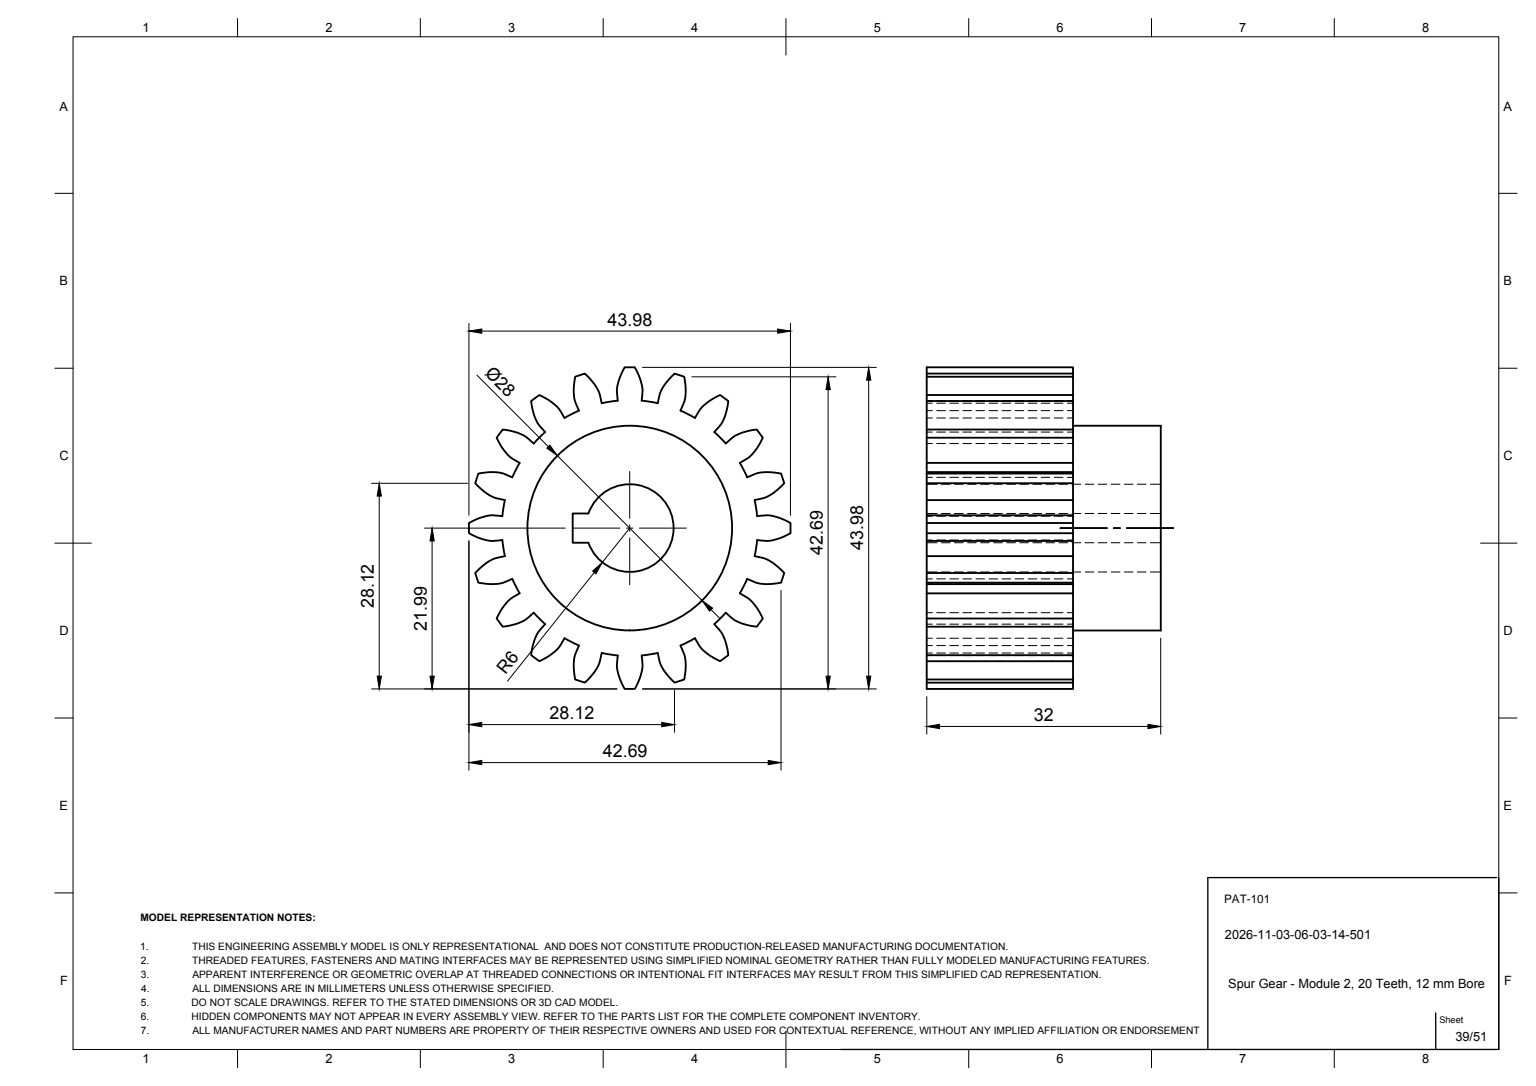
ISO-10303-21;
HEADER;
/* Generated by software containing ST-Developer
 * from STEP Tools, Inc. (www.steptools.com) 
 */

FILE_DESCRIPTION(
/* description */ ('Spur gear reduction stage 2-1 on bearing plates'),
/* implementation_level */ '2;1');

FILE_NAME(
/* name */ 'Spur Gear - Module 2, 20 Teeth, 12 mm Bore.step',
/* time_stamp */ '2026-10-28T03:22:07-07:00',
/* author */ (''),
/* organization */ (''),
/* preprocessor_version */ 'ST-DEVELOPER v20.2',
/* originating_system */ 'Autodesk Translation Framework v15.17.0.0',
/* authorisation */ '');

FILE_SCHEMA (('AUTOMOTIVE_DESIGN { 1 0 10303 214 3 1 1 }'));
ENDSEC;

DATA;
#10=MECHANICAL_DESIGN_GEOMETRIC_PRESENTATION_REPRESENTATION('',(#993),#53909);
#11=(
BOUNDED_SURFACE()
B_SPLINE_SURFACE(5,1,((#21141,#21142),(#21143,#21144),(#21145,#21146),(#21147,
#21148),(#21149,#21150),(#21151,#21152),(#21153,#21154),(#21155,#21156),
(#21157,#21158),(#21159,#21160),(#21161,#21162),(#21163,#21164),(#21165,
#21166),(#21167,#21168),(#21169,#21170),(#21171,#21172),(#21173,#21174),
(#21175,#21176),(#21177,#21178),(#21179,#21180),(#21181,#21182),(#21183,
#21184),(#21185,#21186),(#21187,#21188),(#21189,#21190),(#21191,#21192),
(#21193,#21194),(#21195,#21196),(#21197,#21198),(#21199,#21200),(#21201,
#21202),(#21203,#21204),(#21205,#21206),(#21207,#21208),(#21209,#21210),
(#21211,#21212),(#21213,#21214),(#21215,#21216),(#21217,#21218),(#21219,
#21220),(#21221,#21222),(#21223,#21224),(#21225,#21226),(#21227,#21228),
(#21229,#21230),(#21231,#21232),(#21233,#21234),(#21235,#21236),(#21237,
#21238),(#21239,#21240),(#21241,#21242),(#21243,#21244),(#21245,#21246),
(#21247,#21248),(#21249,#21250),(#21251,#21252),(#21253,#21254),(#21255,
#21256),(#21257,#21258),(#21259,#21260),(#21261,#21262),(#21263,#21264),
(#21265,#21266),(#21267,#21268),(#21269,#21270),(#21271,#21272),(#21273,
#21274),(#21275,#21276),(#21277,#21278),(#21279,#21280)),.UNSPECIFIED.,
 .F.,.F.,.F.)
B_SPLINE_SURFACE_WITH_KNOTS((6,1,1,1,1,1,1,1,1,1,1,1,1,1,1,1,1,1,1,1,1,
1,1,1,1,1,1,1,1,1,1,1,1,1,1,1,1,1,1,1,1,1,1,1,1,1,1,1,1,1,1,1,1,1,1,1,1,
1,1,1,1,1,1,1,1,6),(2,2),(-1.,-0.984615384615383,-0.969230769230768,-0.953846153846152,
-0.938461538461537,-0.923076923076922,-0.907692307692306,-0.892307692307691,
-0.876923076923076,-0.86153846153846,-0.846153846153845,-0.83076923076923,
-0.815384615384614,-0.799999999999999,-0.784615384615384,-0.769230769230768,
-0.753846153846153,-0.738461538461538,-0.723076923076922,-0.707692307692307,
-0.692307692307692,-0.676923076923076,-0.661538461538461,-0.646153846153846,
-0.63076923076923,-0.615384615384615,-0.6,-0.584615384615384,-0.569230769230769,
-0.553846153846154,-0.538461538461538,-0.523076923076923,-0.507692307692308,
-0.492307692307692,-0.476923076923077,-0.461538461538462,-0.446153846153846,
-0.430769230769231,-0.415384615384615,-0.4,-0.384615384615385,-0.369230769230769,
-0.353846153846154,-0.338461538461538,-0.323076923076923,-0.307692307692308,
-0.292307692307692,-0.276923076923077,-0.261538461538462,-0.246153846153846,
-0.230769230769231,-0.215384615384615,-0.2,-0.184615384615385,-0.169230769230769,
-0.153846153846154,-0.138461538461538,-0.123076923076923,-0.107692307692308,
-0.0923076923076923,-0.0769230769230769,-0.0615384615384615,-0.0461538461538462,
-0.0307692307692308,-0.0153846153846154,0.),(-1.,1.),.UNSPECIFIED.)
GEOMETRIC_REPRESENTATION_ITEM()
RATIONAL_B_SPLINE_SURFACE(((1.,1.),(1.,1.),(1.,1.),(1.,1.),(1.,1.),(1.,
1.),(1.,1.),(1.,1.),(1.,1.),(1.,1.),(1.,1.),(1.,1.),(1.,1.),(1.,1.),(1.,
1.),(1.,1.),(1.,1.),(1.,1.),(1.,1.),(1.,1.),(1.,1.),(1.,1.),(1.,1.),(1.,
1.),(1.,1.),(1.,1.),(1.,1.),(1.,1.),(1.,1.),(1.,1.),(1.,1.),(1.,1.),(1.,
1.),(1.,1.),(1.,1.),(1.,1.),(1.,1.),(1.,1.),(1.,1.),(1.,1.),(1.,1.),(1.,
1.),(1.,1.),(1.,1.),(1.,1.),(1.,1.),(1.,1.),(1.,1.),(1.,1.),(1.,1.),(1.,
1.),(1.,1.),(1.,1.),(1.,1.),(1.,1.),(1.,1.),(1.,1.),(1.,1.),(1.,1.),(1.,
1.),(1.,1.),(1.,1.),(1.,1.),(1.,1.),(1.,1.),(1.,1.),(1.,1.),(1.,1.),(1.,
1.),(1.,1.)))
REPRESENTATION_ITEM('')
SURFACE()
);
#12=(
BOUNDED_SURFACE()
B_SPLINE_SURFACE(5,1,((#21359,#21360),(#21361,#21362),(#21363,#21364),(#21365,
#21366),(#21367,#21368),(#21369,#21370),(#21371,#21372),(#21373,#21374),
(#21375,#21376),(#21377,#21378),(#21379,#21380),(#21381,#21382),(#21383,
#21384),(#21385,#21386),(#21387,#21388),(#21389,#21390),(#21391,#21392),
(#21393,#21394),(#21395,#21396),(#21397,#21398),(#21399,#21400),(#21401,
#21402),(#21403,#21404),(#21405,#21406),(#21407,#21408),(#21409,#21410),
(#21411,#21412),(#21413,#21414),(#21415,#21416),(#21417,#21418),(#21419,
#21420),(#21421,#21422),(#21423,#21424),(#21425,#21426),(#21427,#21428),
(#21429,#21430),(#21431,#21432),(#21433,#21434),(#21435,#21436),(#21437,
#21438),(#21439,#21440),(#21441,#21442),(#21443,#21444),(#21445,#21446),
(#21447,#21448),(#21449,#21450),(#21451,#21452),(#21453,#21454),(#21455,
#21456),(#21457,#21458),(#21459,#21460),(#21461,#21462),(#21463,#21464),
(#21465,#21466),(#21467,#21468),(#21469,#21470),(#21471,#21472),(#21473,
#21474),(#21475,#21476),(#21477,#21478),(#21479,#21480),(#21481,#21482),
(#21483,#21484),(#21485,#21486),(#21487,#21488),(#21489,#21490),(#21491,
#21492),(#21493,#21494),(#21495,#21496),(#21497,#21498)),.UNSPECIFIED.,
 .F.,.F.,.F.)
B_SPLINE_SURFACE_WITH_KNOTS((6,1,1,1,1,1,1,1,1,1,1,1,1,1,1,1,1,1,1,1,1,
1,1,1,1,1,1,1,1,1,1,1,1,1,1,1,1,1,1,1,1,1,1,1,1,1,1,1,1,1,1,1,1,1,1,1,1,
1,1,1,1,1,1,1,1,6),(2,2),(-1.,-0.984615384615383,-0.969230769230768,-0.953846153846152,
-0.938461538461537,-0.923076923076922,-0.907692307692306,-0.892307692307691,
-0.876923076923076,-0.86153846153846,-0.846153846153845,-0.83076923076923,
-0.815384615384614,-0.799999999999999,-0.784615384615384,-0.769230769230768,
-0.753846153846153,-0.738461538461538,-0.723076923076922,-0.707692307692307,
-0.692307692307692,-0.676923076923076,-0.661538461538461,-0.646153846153846,
-0.63076923076923,-0.615384615384615,-0.6,-0.584615384615384,-0.569230769230769,
-0.553846153846154,-0.538461538461538,-0.523076923076923,-0.507692307692308,
-0.492307692307692,-0.476923076923077,-0.461538461538462,-0.446153846153846,
-0.430769230769231,-0.415384615384615,-0.4,-0.384615384615385,-0.369230769230769,
-0.353846153846154,-0.338461538461538,-0.323076923076923,-0.307692307692308,
-0.292307692307692,-0.276923076923077,-0.261538461538462,-0.246153846153846,
-0.230769230769231,-0.215384615384615,-0.2,-0.184615384615385,-0.169230769230769,
-0.153846153846154,-0.138461538461538,-0.123076923076923,-0.107692307692308,
-0.0923076923076923,-0.0769230769230769,-0.0615384615384615,-0.0461538461538462,
-0.0307692307692308,-0.0153846153846154,0.),(-1.,1.),.UNSPECIFIED.)
GEOMETRIC_REPRESENTATION_ITEM()
RATIONAL_B_SPLINE_SURFACE(((1.,1.),(1.,1.),(1.,1.),(1.,1.),(1.,1.),(1.,
1.),(1.,1.),(1.,1.),(1.,1.),(1.,1.),(1.,1.),(1.,1.),(1.,1.),(1.,1.),(1.,
1.),(1.,1.),(1.,1.),(1.,1.),(1.,1.),(1.,1.),(1.,1.),(1.,1.),(1.,1.),(1.,
1.),(1.,1.),(1.,1.),(1.,1.),(1.,1.),(1.,1.),(1.,1.),(1.,1.),(1.,1.),(1.,
1.),(1.,1.),(1.,1.),(1.,1.),(1.,1.),(1.,1.),(1.,1.),(1.,1.),(1.,1.),(1.,
1.),(1.,1.),(1.,1.),(1.,1.),(1.,1.),(1.,1.),(1.,1.),(1.,1.),(1.,1.),(1.,
1.),(1.,1.),(1.,1.),(1.,1.),(1.,1.),(1.,1.),(1.,1.),(1.,1.),(1.,1.),(1.,
1.),(1.,1.),(1.,1.),(1.,1.),(1.,1.),(1.,1.),(1.,1.),(1.,1.),(1.,1.),(1.,
1.),(1.,1.)))
REPRESENTATION_ITEM('')
SURFACE()
);
#13=(
BOUNDED_SURFACE()
B_SPLINE_SURFACE(5,1,((#21575,#21576),(#21577,#21578),(#21579,#21580),(#21581,
#21582),(#21583,#21584),(#21585,#21586),(#21587,#21588),(#21589,#21590),
(#21591,#21592),(#21593,#21594),(#21595,#21596),(#21597,#21598),(#21599,
#21600),(#21601,#21602),(#21603,#21604),(#21605,#21606),(#21607,#21608),
(#21609,#21610),(#21611,#21612),(#21613,#21614),(#21615,#21616),(#21617,
#21618),(#21619,#21620),(#21621,#21622),(#21623,#21624),(#21625,#21626),
(#21627,#21628),(#21629,#21630),(#21631,#21632),(#21633,#21634),(#21635,
#21636),(#21637,#21638),(#21639,#21640),(#21641,#21642),(#21643,#21644),
(#21645,#21646),(#21647,#21648),(#21649,#21650),(#21651,#21652),(#21653,
#21654),(#21655,#21656),(#21657,#21658),(#21659,#21660),(#21661,#21662),
(#21663,#21664),(#21665,#21666),(#21667,#21668),(#21669,#21670),(#21671,
#21672),(#21673,#21674),(#21675,#21676),(#21677,#21678),(#21679,#21680),
(#21681,#21682),(#21683,#21684),(#21685,#21686),(#21687,#21688),(#21689,
#21690),(#21691,#21692),(#21693,#21694),(#21695,#21696),(#21697,#21698),
(#21699,#21700),(#21701,#21702),(#21703,#21704),(#21705,#21706),(#21707,
#21708),(#21709,#21710),(#21711,#21712),(#21713,#21714)),.UNSPECIFIED.,
 .F.,.F.,.F.)
B_SPLINE_SURFACE_WITH_KNOTS((6,1,1,1,1,1,1,1,1,1,1,1,1,1,1,1,1,1,1,1,1,
1,1,1,1,1,1,1,1,1,1,1,1,1,1,1,1,1,1,1,1,1,1,1,1,1,1,1,1,1,1,1,1,1,1,1,1,
1,1,1,1,1,1,1,1,6),(2,2),(-1.,-0.984615384615383,-0.969230769230768,-0.953846153846152,
-0.938461538461537,-0.923076923076922,-0.907692307692306,-0.892307692307691,
-0.876923076923076,-0.86153846153846,-0.846153846153845,-0.83076923076923,
-0.815384615384614,-0.799999999999999,-0.784615384615384,-0.769230769230768,
-0.753846153846153,-0.738461538461538,-0.723076923076922,-0.707692307692307,
-0.692307692307692,-0.676923076923076,-0.661538461538461,-0.646153846153846,
-0.63076923076923,-0.615384615384615,-0.6,-0.584615384615384,-0.569230769230769,
-0.553846153846154,-0.538461538461538,-0.523076923076923,-0.507692307692308,
-0.492307692307692,-0.476923076923077,-0.461538461538462,-0.446153846153846,
-0.430769230769231,-0.415384615384615,-0.4,-0.384615384615385,-0.369230769230769,
-0.353846153846154,-0.338461538461538,-0.323076923076923,-0.307692307692308,
-0.292307692307692,-0.276923076923077,-0.261538461538462,-0.246153846153846,
-0.230769230769231,-0.215384615384615,-0.2,-0.184615384615385,-0.169230769230769,
-0.153846153846154,-0.138461538461538,-0.123076923076923,-0.107692307692308,
-0.0923076923076923,-0.0769230769230769,-0.0615384615384615,-0.0461538461538462,
-0.0307692307692308,-0.0153846153846154,0.),(-1.,1.),.UNSPECIFIED.)
GEOMETRIC_REPRESENTATION_ITEM()
RATIONAL_B_SPLINE_SURFACE(((1.,1.),(1.,1.),(1.,1.),(1.,1.),(1.,1.),(1.,
1.),(1.,1.),(1.,1.),(1.,1.),(1.,1.),(1.,1.),(1.,1.),(1.,1.),(1.,1.),(1.,
1.),(1.,1.),(1.,1.),(1.,1.),(1.,1.),(1.,1.),(1.,1.),(1.,1.),(1.,1.),(1.,
1.),(1.,1.),(1.,1.),(1.,1.),(1.,1.),(1.,1.),(1.,1.),(1.,1.),(1.,1.),(1.,
1.),(1.,1.),(1.,1.),(1.,1.),(1.,1.),(1.,1.),(1.,1.),(1.,1.),(1.,1.),(1.,
1.),(1.,1.),(1.,1.),(1.,1.),(1.,1.),(1.,1.),(1.,1.),(1.,1.),(1.,1.),(1.,
1.),(1.,1.),(1.,1.),(1.,1.),(1.,1.),(1.,1.),(1.,1.),(1.,1.),(1.,1.),(1.,
1.),(1.,1.),(1.,1.),(1.,1.),(1.,1.),(1.,1.),(1.,1.),(1.,1.),(1.,1.),(1.,
1.),(1.,1.)))
REPRESENTATION_ITEM('')
SURFACE()
);
#14=(
BOUNDED_SURFACE()
B_SPLINE_SURFACE(5,1,((#21791,#21792),(#21793,#21794),(#21795,#21796),(#21797,
#21798),(#21799,#21800),(#21801,#21802),(#21803,#21804),(#21805,#21806),
(#21807,#21808),(#21809,#21810),(#21811,#21812),(#21813,#21814),(#21815,
#21816),(#21817,#21818),(#21819,#21820),(#21821,#21822),(#21823,#21824),
(#21825,#21826),(#21827,#21828),(#21829,#21830),(#21831,#21832),(#21833,
#21834),(#21835,#21836),(#21837,#21838),(#21839,#21840),(#21841,#21842),
(#21843,#21844),(#21845,#21846),(#21847,#21848),(#21849,#21850),(#21851,
#21852),(#21853,#21854),(#21855,#21856),(#21857,#21858),(#21859,#21860),
(#21861,#21862),(#21863,#21864),(#21865,#21866),(#21867,#21868),(#21869,
#21870),(#21871,#21872),(#21873,#21874),(#21875,#21876),(#21877,#21878),
(#21879,#21880),(#21881,#21882),(#21883,#21884),(#21885,#21886),(#21887,
#21888),(#21889,#21890),(#21891,#21892),(#21893,#21894),(#21895,#21896),
(#21897,#21898),(#21899,#21900),(#21901,#21902),(#21903,#21904),(#21905,
#21906),(#21907,#21908),(#21909,#21910),(#21911,#21912),(#21913,#21914),
(#21915,#21916),(#21917,#21918),(#21919,#21920),(#21921,#21922),(#21923,
#21924),(#21925,#21926),(#21927,#21928),(#21929,#21930)),.UNSPECIFIED.,
 .F.,.F.,.F.)
B_SPLINE_SURFACE_WITH_KNOTS((6,1,1,1,1,1,1,1,1,1,1,1,1,1,1,1,1,1,1,1,1,
1,1,1,1,1,1,1,1,1,1,1,1,1,1,1,1,1,1,1,1,1,1,1,1,1,1,1,1,1,1,1,1,1,1,1,1,
1,1,1,1,1,1,1,1,6),(2,2),(-1.,-0.984615384615383,-0.969230769230768,-0.953846153846152,
-0.938461538461537,-0.923076923076922,-0.907692307692306,-0.892307692307691,
-0.876923076923076,-0.86153846153846,-0.846153846153845,-0.83076923076923,
-0.815384615384614,-0.799999999999999,-0.784615384615384,-0.769230769230768,
-0.753846153846153,-0.738461538461538,-0.723076923076922,-0.707692307692307,
-0.692307692307692,-0.676923076923076,-0.661538461538461,-0.646153846153846,
-0.63076923076923,-0.615384615384615,-0.6,-0.584615384615384,-0.569230769230769,
-0.553846153846154,-0.538461538461538,-0.523076923076923,-0.507692307692308,
-0.492307692307692,-0.476923076923077,-0.461538461538462,-0.446153846153846,
-0.430769230769231,-0.415384615384615,-0.4,-0.384615384615385,-0.369230769230769,
-0.353846153846154,-0.338461538461538,-0.323076923076923,-0.307692307692308,
-0.292307692307692,-0.276923076923077,-0.261538461538462,-0.246153846153846,
-0.230769230769231,-0.215384615384615,-0.2,-0.184615384615385,-0.169230769230769,
-0.153846153846154,-0.138461538461538,-0.123076923076923,-0.107692307692308,
-0.0923076923076923,-0.0769230769230769,-0.0615384615384615,-0.0461538461538462,
-0.0307692307692308,-0.0153846153846154,0.),(-1.,1.),.UNSPECIFIED.)
GEOMETRIC_REPRESENTATION_ITEM()
RATIONAL_B_SPLINE_SURFACE(((1.,1.),(1.,1.),(1.,1.),(1.,1.),(1.,1.),(1.,
1.),(1.,1.),(1.,1.),(1.,1.),(1.,1.),(1.,1.),(1.,1.),(1.,1.),(1.,1.),(1.,
1.),(1.,1.),(1.,1.),(1.,1.),(1.,1.),(1.,1.),(1.,1.),(1.,1.),(1.,1.),(1.,
1.),(1.,1.),(1.,1.),(1.,1.),(1.,1.),(1.,1.),(1.,1.),(1.,1.),(1.,1.),(1.,
1.),(1.,1.),(1.,1.),(1.,1.),(1.,1.),(1.,1.),(1.,1.),(1.,1.),(1.,1.),(1.,
1.),(1.,1.),(1.,1.),(1.,1.),(1.,1.),(1.,1.),(1.,1.),(1.,1.),(1.,1.),(1.,
1.),(1.,1.),(1.,1.),(1.,1.),(1.,1.),(1.,1.),(1.,1.),(1.,1.),(1.,1.),(1.,
1.),(1.,1.),(1.,1.),(1.,1.),(1.,1.),(1.,1.),(1.,1.),(1.,1.),(1.,1.),(1.,
1.),(1.,1.)))
REPRESENTATION_ITEM('')
SURFACE()
);
#15=(
BOUNDED_SURFACE()
B_SPLINE_SURFACE(5,1,((#22007,#22008),(#22009,#22010),(#22011,#22012),(#22013,
#22014),(#22015,#22016),(#22017,#22018),(#22019,#22020),(#22021,#22022),
(#22023,#22024),(#22025,#22026),(#22027,#22028),(#22029,#22030),(#22031,
#22032),(#22033,#22034),(#22035,#22036),(#22037,#22038),(#22039,#22040),
(#22041,#22042),(#22043,#22044),(#22045,#22046),(#22047,#22048),(#22049,
#22050),(#22051,#22052),(#22053,#22054),(#22055,#22056),(#22057,#22058),
(#22059,#22060),(#22061,#22062),(#22063,#22064),(#22065,#22066),(#22067,
#22068),(#22069,#22070),(#22071,#22072),(#22073,#22074),(#22075,#22076),
(#22077,#22078),(#22079,#22080),(#22081,#22082),(#22083,#22084),(#22085,
#22086),(#22087,#22088),(#22089,#22090),(#22091,#22092),(#22093,#22094),
(#22095,#22096),(#22097,#22098),(#22099,#22100),(#22101,#22102),(#22103,
#22104),(#22105,#22106),(#22107,#22108),(#22109,#22110),(#22111,#22112),
(#22113,#22114),(#22115,#22116),(#22117,#22118),(#22119,#22120),(#22121,
#22122),(#22123,#22124),(#22125,#22126),(#22127,#22128),(#22129,#22130),
(#22131,#22132),(#22133,#22134),(#22135,#22136),(#22137,#22138),(#22139,
#22140),(#22141,#22142),(#22143,#22144),(#22145,#22146)),.UNSPECIFIED.,
 .F.,.F.,.F.)
B_SPLINE_SURFACE_WITH_KNOTS((6,1,1,1,1,1,1,1,1,1,1,1,1,1,1,1,1,1,1,1,1,
1,1,1,1,1,1,1,1,1,1,1,1,1,1,1,1,1,1,1,1,1,1,1,1,1,1,1,1,1,1,1,1,1,1,1,1,
1,1,1,1,1,1,1,1,6),(2,2),(-1.,-0.984615384615383,-0.969230769230768,-0.953846153846152,
-0.938461538461537,-0.923076923076922,-0.907692307692306,-0.892307692307691,
-0.876923076923076,-0.86153846153846,-0.846153846153845,-0.83076923076923,
-0.815384615384614,-0.799999999999999,-0.784615384615384,-0.769230769230768,
-0.753846153846153,-0.738461538461538,-0.723076923076922,-0.707692307692307,
-0.692307692307692,-0.676923076923076,-0.661538461538461,-0.646153846153846,
-0.63076923076923,-0.615384615384615,-0.6,-0.584615384615384,-0.569230769230769,
-0.553846153846154,-0.538461538461538,-0.523076923076923,-0.507692307692308,
-0.492307692307692,-0.476923076923077,-0.461538461538462,-0.446153846153846,
-0.430769230769231,-0.415384615384615,-0.4,-0.384615384615385,-0.369230769230769,
-0.353846153846154,-0.338461538461538,-0.323076923076923,-0.307692307692308,
-0.292307692307692,-0.276923076923077,-0.261538461538462,-0.246153846153846,
-0.230769230769231,-0.215384615384615,-0.2,-0.184615384615385,-0.169230769230769,
-0.153846153846154,-0.138461538461538,-0.123076923076923,-0.107692307692308,
-0.0923076923076923,-0.0769230769230769,-0.0615384615384615,-0.0461538461538462,
-0.0307692307692308,-0.0153846153846154,0.),(-1.,1.),.UNSPECIFIED.)
GEOMETRIC_REPRESENTATION_ITEM()
RATIONAL_B_SPLINE_SURFACE(((1.,1.),(1.,1.),(1.,1.),(1.,1.),(1.,1.),(1.,
1.),(1.,1.),(1.,1.),(1.,1.),(1.,1.),(1.,1.),(1.,1.),(1.,1.),(1.,1.),(1.,
1.),(1.,1.),(1.,1.),(1.,1.),(1.,1.),(1.,1.),(1.,1.),(1.,1.),(1.,1.),(1.,
1.),(1.,1.),(1.,1.),(1.,1.),(1.,1.),(1.,1.),(1.,1.),(1.,1.),(1.,1.),(1.,
1.),(1.,1.),(1.,1.),(1.,1.),(1.,1.),(1.,1.),(1.,1.),(1.,1.),(1.,1.),(1.,
1.),(1.,1.),(1.,1.),(1.,1.),(1.,1.),(1.,1.),(1.,1.),(1.,1.),(1.,1.),(1.,
1.),(1.,1.),(1.,1.),(1.,1.),(1.,1.),(1.,1.),(1.,1.),(1.,1.),(1.,1.),(1.,
1.),(1.,1.),(1.,1.),(1.,1.),(1.,1.),(1.,1.),(1.,1.),(1.,1.),(1.,1.),(1.,
1.),(1.,1.)))
REPRESENTATION_ITEM('')
SURFACE()
);
#16=(
BOUNDED_SURFACE()
B_SPLINE_SURFACE(5,1,((#22223,#22224),(#22225,#22226),(#22227,#22228),(#22229,
#22230),(#22231,#22232),(#22233,#22234),(#22235,#22236),(#22237,#22238),
(#22239,#22240),(#22241,#22242),(#22243,#22244),(#22245,#22246),(#22247,
#22248),(#22249,#22250),(#22251,#22252),(#22253,#22254),(#22255,#22256),
(#22257,#22258),(#22259,#22260),(#22261,#22262),(#22263,#22264),(#22265,
#22266),(#22267,#22268),(#22269,#22270),(#22271,#22272),(#22273,#22274),
(#22275,#22276),(#22277,#22278),(#22279,#22280),(#22281,#22282),(#22283,
#22284),(#22285,#22286),(#22287,#22288),(#22289,#22290),(#22291,#22292),
(#22293,#22294),(#22295,#22296),(#22297,#22298),(#22299,#22300),(#22301,
#22302),(#22303,#22304),(#22305,#22306),(#22307,#22308),(#22309,#22310),
(#22311,#22312),(#22313,#22314),(#22315,#22316),(#22317,#22318),(#22319,
#22320),(#22321,#22322),(#22323,#22324),(#22325,#22326),(#22327,#22328),
(#22329,#22330),(#22331,#22332),(#22333,#22334),(#22335,#22336),(#22337,
#22338),(#22339,#22340),(#22341,#22342),(#22343,#22344),(#22345,#22346),
(#22347,#22348),(#22349,#22350),(#22351,#22352),(#22353,#22354),(#22355,
#22356),(#22357,#22358),(#22359,#22360),(#22361,#22362)),.UNSPECIFIED.,
 .F.,.F.,.F.)
B_SPLINE_SURFACE_WITH_KNOTS((6,1,1,1,1,1,1,1,1,1,1,1,1,1,1,1,1,1,1,1,1,
1,1,1,1,1,1,1,1,1,1,1,1,1,1,1,1,1,1,1,1,1,1,1,1,1,1,1,1,1,1,1,1,1,1,1,1,
1,1,1,1,1,1,1,1,6),(2,2),(-1.,-0.984615384615383,-0.969230769230768,-0.953846153846152,
-0.938461538461537,-0.923076923076922,-0.907692307692306,-0.892307692307691,
-0.876923076923076,-0.86153846153846,-0.846153846153845,-0.83076923076923,
-0.815384615384614,-0.799999999999999,-0.784615384615384,-0.769230769230768,
-0.753846153846153,-0.738461538461538,-0.723076923076922,-0.707692307692307,
-0.692307692307692,-0.676923076923076,-0.661538461538461,-0.646153846153846,
-0.63076923076923,-0.615384615384615,-0.6,-0.584615384615384,-0.569230769230769,
-0.553846153846154,-0.538461538461538,-0.523076923076923,-0.507692307692308,
-0.492307692307692,-0.476923076923077,-0.461538461538462,-0.446153846153846,
-0.430769230769231,-0.415384615384615,-0.4,-0.384615384615385,-0.369230769230769,
-0.353846153846154,-0.338461538461538,-0.323076923076923,-0.307692307692308,
-0.292307692307692,-0.276923076923077,-0.261538461538462,-0.246153846153846,
-0.230769230769231,-0.215384615384615,-0.2,-0.184615384615385,-0.169230769230769,
-0.153846153846154,-0.138461538461538,-0.123076923076923,-0.107692307692308,
-0.0923076923076923,-0.0769230769230769,-0.0615384615384615,-0.0461538461538462,
-0.0307692307692308,-0.0153846153846154,0.),(-1.,1.),.UNSPECIFIED.)
GEOMETRIC_REPRESENTATION_ITEM()
RATIONAL_B_SPLINE_SURFACE(((1.,1.),(1.,1.),(1.,1.),(1.,1.),(1.,1.),(1.,
1.),(1.,1.),(1.,1.),(1.,1.),(1.,1.),(1.,1.),(1.,1.),(1.,1.),(1.,1.),(1.,
1.),(1.,1.),(1.,1.),(1.,1.),(1.,1.),(1.,1.),(1.,1.),(1.,1.),(1.,1.),(1.,
1.),(1.,1.),(1.,1.),(1.,1.),(1.,1.),(1.,1.),(1.,1.),(1.,1.),(1.,1.),(1.,
1.),(1.,1.),(1.,1.),(1.,1.),(1.,1.),(1.,1.),(1.,1.),(1.,1.),(1.,1.),(1.,
1.),(1.,1.),(1.,1.),(1.,1.),(1.,1.),(1.,1.),(1.,1.),(1.,1.),(1.,1.),(1.,
1.),(1.,1.),(1.,1.),(1.,1.),(1.,1.),(1.,1.),(1.,1.),(1.,1.),(1.,1.),(1.,
1.),(1.,1.),(1.,1.),(1.,1.),(1.,1.),(1.,1.),(1.,1.),(1.,1.),(1.,1.),(1.,
1.),(1.,1.)))
REPRESENTATION_ITEM('')
SURFACE()
);
#17=(
BOUNDED_SURFACE()
B_SPLINE_SURFACE(5,1,((#22439,#22440),(#22441,#22442),(#22443,#22444),(#22445,
#22446),(#22447,#22448),(#22449,#22450),(#22451,#22452),(#22453,#22454),
(#22455,#22456),(#22457,#22458),(#22459,#22460),(#22461,#22462),(#22463,
#22464),(#22465,#22466),(#22467,#22468),(#22469,#22470),(#22471,#22472),
(#22473,#22474),(#22475,#22476),(#22477,#22478),(#22479,#22480),(#22481,
#22482),(#22483,#22484),(#22485,#22486),(#22487,#22488),(#22489,#22490),
(#22491,#22492),(#22493,#22494),(#22495,#22496),(#22497,#22498),(#22499,
#22500),(#22501,#22502),(#22503,#22504),(#22505,#22506),(#22507,#22508),
(#22509,#22510),(#22511,#22512),(#22513,#22514),(#22515,#22516),(#22517,
#22518),(#22519,#22520),(#22521,#22522),(#22523,#22524),(#22525,#22526),
(#22527,#22528),(#22529,#22530),(#22531,#22532),(#22533,#22534),(#22535,
#22536),(#22537,#22538),(#22539,#22540),(#22541,#22542),(#22543,#22544),
(#22545,#22546),(#22547,#22548),(#22549,#22550),(#22551,#22552),(#22553,
#22554),(#22555,#22556),(#22557,#22558),(#22559,#22560),(#22561,#22562),
(#22563,#22564),(#22565,#22566),(#22567,#22568),(#22569,#22570),(#22571,
#22572),(#22573,#22574),(#22575,#22576),(#22577,#22578)),.UNSPECIFIED.,
 .F.,.F.,.F.)
B_SPLINE_SURFACE_WITH_KNOTS((6,1,1,1,1,1,1,1,1,1,1,1,1,1,1,1,1,1,1,1,1,
1,1,1,1,1,1,1,1,1,1,1,1,1,1,1,1,1,1,1,1,1,1,1,1,1,1,1,1,1,1,1,1,1,1,1,1,
1,1,1,1,1,1,1,1,6),(2,2),(-1.,-0.984615384615383,-0.969230769230768,-0.953846153846152,
-0.938461538461537,-0.923076923076922,-0.907692307692306,-0.892307692307691,
-0.876923076923076,-0.86153846153846,-0.846153846153845,-0.83076923076923,
-0.815384615384614,-0.799999999999999,-0.784615384615384,-0.769230769230768,
-0.753846153846153,-0.738461538461538,-0.723076923076922,-0.707692307692307,
-0.692307692307692,-0.676923076923076,-0.661538461538461,-0.646153846153846,
-0.63076923076923,-0.615384615384615,-0.6,-0.584615384615384,-0.569230769230769,
-0.553846153846154,-0.538461538461538,-0.523076923076923,-0.507692307692308,
-0.492307692307692,-0.476923076923077,-0.461538461538462,-0.446153846153846,
-0.430769230769231,-0.415384615384615,-0.4,-0.384615384615385,-0.369230769230769,
-0.353846153846154,-0.338461538461538,-0.323076923076923,-0.307692307692308,
-0.292307692307692,-0.276923076923077,-0.261538461538462,-0.246153846153846,
-0.230769230769231,-0.215384615384615,-0.2,-0.184615384615385,-0.169230769230769,
-0.153846153846154,-0.138461538461538,-0.123076923076923,-0.107692307692308,
-0.0923076923076923,-0.0769230769230769,-0.0615384615384615,-0.0461538461538462,
-0.0307692307692308,-0.0153846153846154,0.),(-1.,1.),.UNSPECIFIED.)
GEOMETRIC_REPRESENTATION_ITEM()
RATIONAL_B_SPLINE_SURFACE(((1.,1.),(1.,1.),(1.,1.),(1.,1.),(1.,1.),(1.,
1.),(1.,1.),(1.,1.),(1.,1.),(1.,1.),(1.,1.),(1.,1.),(1.,1.),(1.,1.),(1.,
1.),(1.,1.),(1.,1.),(1.,1.),(1.,1.),(1.,1.),(1.,1.),(1.,1.),(1.,1.),(1.,
1.),(1.,1.),(1.,1.),(1.,1.),(1.,1.),(1.,1.),(1.,1.),(1.,1.),(1.,1.),(1.,
1.),(1.,1.),(1.,1.),(1.,1.),(1.,1.),(1.,1.),(1.,1.),(1.,1.),(1.,1.),(1.,
1.),(1.,1.),(1.,1.),(1.,1.),(1.,1.),(1.,1.),(1.,1.),(1.,1.),(1.,1.),(1.,
1.),(1.,1.),(1.,1.),(1.,1.),(1.,1.),(1.,1.),(1.,1.),(1.,1.),(1.,1.),(1.,
1.),(1.,1.),(1.,1.),(1.,1.),(1.,1.),(1.,1.),(1.,1.),(1.,1.),(1.,1.),(1.,
1.),(1.,1.)))
REPRESENTATION_ITEM('')
SURFACE()
);
#18=(
BOUNDED_SURFACE()
B_SPLINE_SURFACE(5,1,((#22655,#22656),(#22657,#22658),(#22659,#22660),(#22661,
#22662),(#22663,#22664),(#22665,#22666),(#22667,#22668),(#22669,#22670),
(#22671,#22672),(#22673,#22674),(#22675,#22676),(#22677,#22678),(#22679,
#22680),(#22681,#22682),(#22683,#22684),(#22685,#22686),(#22687,#22688),
(#22689,#22690),(#22691,#22692),(#22693,#22694),(#22695,#22696),(#22697,
#22698),(#22699,#22700),(#22701,#22702),(#22703,#22704),(#22705,#22706),
(#22707,#22708),(#22709,#22710),(#22711,#22712),(#22713,#22714),(#22715,
#22716),(#22717,#22718),(#22719,#22720),(#22721,#22722),(#22723,#22724),
(#22725,#22726),(#22727,#22728),(#22729,#22730),(#22731,#22732),(#22733,
#22734),(#22735,#22736),(#22737,#22738),(#22739,#22740),(#22741,#22742),
(#22743,#22744),(#22745,#22746),(#22747,#22748),(#22749,#22750),(#22751,
#22752),(#22753,#22754),(#22755,#22756),(#22757,#22758),(#22759,#22760),
(#22761,#22762),(#22763,#22764),(#22765,#22766),(#22767,#22768),(#22769,
#22770),(#22771,#22772),(#22773,#22774),(#22775,#22776),(#22777,#22778),
(#22779,#22780),(#22781,#22782),(#22783,#22784),(#22785,#22786),(#22787,
#22788),(#22789,#22790),(#22791,#22792),(#22793,#22794)),.UNSPECIFIED.,
 .F.,.F.,.F.)
B_SPLINE_SURFACE_WITH_KNOTS((6,1,1,1,1,1,1,1,1,1,1,1,1,1,1,1,1,1,1,1,1,
1,1,1,1,1,1,1,1,1,1,1,1,1,1,1,1,1,1,1,1,1,1,1,1,1,1,1,1,1,1,1,1,1,1,1,1,
1,1,1,1,1,1,1,1,6),(2,2),(-1.,-0.984615384615383,-0.969230769230768,-0.953846153846152,
-0.938461538461537,-0.923076923076922,-0.907692307692306,-0.892307692307691,
-0.876923076923076,-0.86153846153846,-0.846153846153845,-0.83076923076923,
-0.815384615384614,-0.799999999999999,-0.784615384615384,-0.769230769230768,
-0.753846153846153,-0.738461538461538,-0.723076923076922,-0.707692307692307,
-0.692307692307692,-0.676923076923076,-0.661538461538461,-0.646153846153846,
-0.63076923076923,-0.615384615384615,-0.6,-0.584615384615384,-0.569230769230769,
-0.553846153846154,-0.538461538461538,-0.523076923076923,-0.507692307692308,
-0.492307692307692,-0.476923076923077,-0.461538461538462,-0.446153846153846,
-0.430769230769231,-0.415384615384615,-0.4,-0.384615384615385,-0.369230769230769,
-0.353846153846154,-0.338461538461538,-0.323076923076923,-0.307692307692308,
-0.292307692307692,-0.276923076923077,-0.261538461538462,-0.246153846153846,
-0.230769230769231,-0.215384615384615,-0.2,-0.184615384615385,-0.169230769230769,
-0.153846153846154,-0.138461538461538,-0.123076923076923,-0.107692307692308,
-0.0923076923076923,-0.0769230769230769,-0.0615384615384615,-0.0461538461538462,
-0.0307692307692308,-0.0153846153846154,0.),(-1.,1.),.UNSPECIFIED.)
GEOMETRIC_REPRESENTATION_ITEM()
RATIONAL_B_SPLINE_SURFACE(((1.,1.),(1.,1.),(1.,1.),(1.,1.),(1.,1.),(1.,
1.),(1.,1.),(1.,1.),(1.,1.),(1.,1.),(1.,1.),(1.,1.),(1.,1.),(1.,1.),(1.,
1.),(1.,1.),(1.,1.),(1.,1.),(1.,1.),(1.,1.),(1.,1.),(1.,1.),(1.,1.),(1.,
1.),(1.,1.),(1.,1.),(1.,1.),(1.,1.),(1.,1.),(1.,1.),(1.,1.),(1.,1.),(1.,
1.),(1.,1.),(1.,1.),(1.,1.),(1.,1.),(1.,1.),(1.,1.),(1.,1.),(1.,1.),(1.,
1.),(1.,1.),(1.,1.),(1.,1.),(1.,1.),(1.,1.),(1.,1.),(1.,1.),(1.,1.),(1.,
1.),(1.,1.),(1.,1.),(1.,1.),(1.,1.),(1.,1.),(1.,1.),(1.,1.),(1.,1.),(1.,
1.),(1.,1.),(1.,1.),(1.,1.),(1.,1.),(1.,1.),(1.,1.),(1.,1.),(1.,1.),(1.,
1.),(1.,1.)))
REPRESENTATION_ITEM('')
SURFACE()
);
#19=(
BOUNDED_SURFACE()
B_SPLINE_SURFACE(5,1,((#22871,#22872),(#22873,#22874),(#22875,#22876),(#22877,
#22878),(#22879,#22880),(#22881,#22882),(#22883,#22884),(#22885,#22886),
(#22887,#22888),(#22889,#22890),(#22891,#22892),(#22893,#22894),(#22895,
#22896),(#22897,#22898),(#22899,#22900),(#22901,#22902),(#22903,#22904),
(#22905,#22906),(#22907,#22908),(#22909,#22910),(#22911,#22912),(#22913,
#22914),(#22915,#22916),(#22917,#22918),(#22919,#22920),(#22921,#22922),
(#22923,#22924),(#22925,#22926),(#22927,#22928),(#22929,#22930),(#22931,
#22932),(#22933,#22934),(#22935,#22936),(#22937,#22938),(#22939,#22940),
(#22941,#22942),(#22943,#22944),(#22945,#22946),(#22947,#22948),(#22949,
#22950),(#22951,#22952),(#22953,#22954),(#22955,#22956),(#22957,#22958),
(#22959,#22960),(#22961,#22962),(#22963,#22964),(#22965,#22966),(#22967,
#22968),(#22969,#22970),(#22971,#22972),(#22973,#22974),(#22975,#22976),
(#22977,#22978),(#22979,#22980),(#22981,#22982),(#22983,#22984),(#22985,
#22986),(#22987,#22988),(#22989,#22990),(#22991,#22992),(#22993,#22994),
(#22995,#22996),(#22997,#22998),(#22999,#23000),(#23001,#23002),(#23003,
#23004),(#23005,#23006),(#23007,#23008),(#23009,#23010)),.UNSPECIFIED.,
 .F.,.F.,.F.)
B_SPLINE_SURFACE_WITH_KNOTS((6,1,1,1,1,1,1,1,1,1,1,1,1,1,1,1,1,1,1,1,1,
1,1,1,1,1,1,1,1,1,1,1,1,1,1,1,1,1,1,1,1,1,1,1,1,1,1,1,1,1,1,1,1,1,1,1,1,
1,1,1,1,1,1,1,1,6),(2,2),(-1.,-0.984615384615383,-0.969230769230768,-0.953846153846152,
-0.938461538461537,-0.923076923076922,-0.907692307692306,-0.892307692307691,
-0.876923076923076,-0.86153846153846,-0.846153846153845,-0.83076923076923,
-0.815384615384614,-0.799999999999999,-0.784615384615384,-0.769230769230768,
-0.753846153846153,-0.738461538461538,-0.723076923076922,-0.707692307692307,
-0.692307692307692,-0.676923076923076,-0.661538461538461,-0.646153846153846,
-0.63076923076923,-0.615384615384615,-0.6,-0.584615384615384,-0.569230769230769,
-0.553846153846154,-0.538461538461538,-0.523076923076923,-0.507692307692308,
-0.492307692307692,-0.476923076923077,-0.461538461538462,-0.446153846153846,
-0.430769230769231,-0.415384615384615,-0.4,-0.384615384615385,-0.369230769230769,
-0.353846153846154,-0.338461538461538,-0.323076923076923,-0.307692307692308,
-0.292307692307692,-0.276923076923077,-0.261538461538462,-0.246153846153846,
-0.230769230769231,-0.215384615384615,-0.2,-0.184615384615385,-0.169230769230769,
-0.153846153846154,-0.138461538461538,-0.123076923076923,-0.107692307692308,
-0.0923076923076923,-0.0769230769230769,-0.0615384615384615,-0.0461538461538462,
-0.0307692307692308,-0.0153846153846154,0.),(-1.,1.),.UNSPECIFIED.)
GEOMETRIC_REPRESENTATION_ITEM()
RATIONAL_B_SPLINE_SURFACE(((1.,1.),(1.,1.),(1.,1.),(1.,1.),(1.,1.),(1.,
1.),(1.,1.),(1.,1.),(1.,1.),(1.,1.),(1.,1.),(1.,1.),(1.,1.),(1.,1.),(1.,
1.),(1.,1.),(1.,1.),(1.,1.),(1.,1.),(1.,1.),(1.,1.),(1.,1.),(1.,1.),(1.,
1.),(1.,1.),(1.,1.),(1.,1.),(1.,1.),(1.,1.),(1.,1.),(1.,1.),(1.,1.),(1.,
1.),(1.,1.),(1.,1.),(1.,1.),(1.,1.),(1.,1.),(1.,1.),(1.,1.),(1.,1.),(1.,
1.),(1.,1.),(1.,1.),(1.,1.),(1.,1.),(1.,1.),(1.,1.),(1.,1.),(1.,1.),(1.,
1.),(1.,1.),(1.,1.),(1.,1.),(1.,1.),(1.,1.),(1.,1.),(1.,1.),(1.,1.),(1.,
1.),(1.,1.),(1.,1.),(1.,1.),(1.,1.),(1.,1.),(1.,1.),(1.,1.),(1.,1.),(1.,
1.),(1.,1.)))
REPRESENTATION_ITEM('')
SURFACE()
);
#20=(
BOUNDED_SURFACE()
B_SPLINE_SURFACE(5,1,((#23087,#23088),(#23089,#23090),(#23091,#23092),(#23093,
#23094),(#23095,#23096),(#23097,#23098),(#23099,#23100),(#23101,#23102),
(#23103,#23104),(#23105,#23106),(#23107,#23108),(#23109,#23110),(#23111,
#23112),(#23113,#23114),(#23115,#23116),(#23117,#23118),(#23119,#23120),
(#23121,#23122),(#23123,#23124),(#23125,#23126),(#23127,#23128),(#23129,
#23130),(#23131,#23132),(#23133,#23134),(#23135,#23136),(#23137,#23138),
(#23139,#23140),(#23141,#23142),(#23143,#23144),(#23145,#23146),(#23147,
#23148),(#23149,#23150),(#23151,#23152),(#23153,#23154),(#23155,#23156),
(#23157,#23158),(#23159,#23160),(#23161,#23162),(#23163,#23164),(#23165,
#23166),(#23167,#23168),(#23169,#23170),(#23171,#23172),(#23173,#23174),
(#23175,#23176),(#23177,#23178),(#23179,#23180),(#23181,#23182),(#23183,
#23184),(#23185,#23186),(#23187,#23188),(#23189,#23190),(#23191,#23192),
(#23193,#23194),(#23195,#23196),(#23197,#23198),(#23199,#23200),(#23201,
#23202),(#23203,#23204),(#23205,#23206),(#23207,#23208),(#23209,#23210),
(#23211,#23212),(#23213,#23214),(#23215,#23216),(#23217,#23218),(#23219,
#23220),(#23221,#23222),(#23223,#23224),(#23225,#23226)),.UNSPECIFIED.,
 .F.,.F.,.F.)
B_SPLINE_SURFACE_WITH_KNOTS((6,1,1,1,1,1,1,1,1,1,1,1,1,1,1,1,1,1,1,1,1,
1,1,1,1,1,1,1,1,1,1,1,1,1,1,1,1,1,1,1,1,1,1,1,1,1,1,1,1,1,1,1,1,1,1,1,1,
1,1,1,1,1,1,1,1,6),(2,2),(-1.,-0.984615384615383,-0.969230769230768,-0.953846153846152,
-0.938461538461537,-0.923076923076922,-0.907692307692306,-0.892307692307691,
-0.876923076923076,-0.86153846153846,-0.846153846153845,-0.83076923076923,
-0.815384615384614,-0.799999999999999,-0.784615384615384,-0.769230769230768,
-0.753846153846153,-0.738461538461538,-0.723076923076922,-0.707692307692307,
-0.692307692307692,-0.676923076923076,-0.661538461538461,-0.646153846153846,
-0.63076923076923,-0.615384615384615,-0.6,-0.584615384615384,-0.569230769230769,
-0.553846153846154,-0.538461538461538,-0.523076923076923,-0.507692307692308,
-0.492307692307692,-0.476923076923077,-0.461538461538462,-0.446153846153846,
-0.430769230769231,-0.415384615384615,-0.4,-0.384615384615385,-0.369230769230769,
-0.353846153846154,-0.338461538461538,-0.323076923076923,-0.307692307692308,
-0.292307692307692,-0.276923076923077,-0.261538461538462,-0.246153846153846,
-0.230769230769231,-0.215384615384615,-0.2,-0.184615384615385,-0.169230769230769,
-0.153846153846154,-0.138461538461538,-0.123076923076923,-0.107692307692308,
-0.0923076923076923,-0.0769230769230769,-0.0615384615384615,-0.0461538461538462,
-0.0307692307692308,-0.0153846153846154,0.),(-1.,1.),.UNSPECIFIED.)
GEOMETRIC_REPRESENTATION_ITEM()
RATIONAL_B_SPLINE_SURFACE(((1.,1.),(1.,1.),(1.,1.),(1.,1.),(1.,1.),(1.,
1.),(1.,1.),(1.,1.),(1.,1.),(1.,1.),(1.,1.),(1.,1.),(1.,1.),(1.,1.),(1.,
1.),(1.,1.),(1.,1.),(1.,1.),(1.,1.),(1.,1.),(1.,1.),(1.,1.),(1.,1.),(1.,
1.),(1.,1.),(1.,1.),(1.,1.),(1.,1.),(1.,1.),(1.,1.),(1.,1.),(1.,1.),(1.,
1.),(1.,1.),(1.,1.),(1.,1.),(1.,1.),(1.,1.),(1.,1.),(1.,1.),(1.,1.),(1.,
1.),(1.,1.),(1.,1.),(1.,1.),(1.,1.),(1.,1.),(1.,1.),(1.,1.),(1.,1.),(1.,
1.),(1.,1.),(1.,1.),(1.,1.),(1.,1.),(1.,1.),(1.,1.),(1.,1.),(1.,1.),(1.,
1.),(1.,1.),(1.,1.),(1.,1.),(1.,1.),(1.,1.),(1.,1.),(1.,1.),(1.,1.),(1.,
1.),(1.,1.)))
REPRESENTATION_ITEM('')
SURFACE()
);
#21=(
BOUNDED_SURFACE()
B_SPLINE_SURFACE(5,1,((#23303,#23304),(#23305,#23306),(#23307,#23308),(#23309,
#23310),(#23311,#23312),(#23313,#23314),(#23315,#23316),(#23317,#23318),
(#23319,#23320),(#23321,#23322),(#23323,#23324),(#23325,#23326),(#23327,
#23328),(#23329,#23330),(#23331,#23332),(#23333,#23334),(#23335,#23336),
(#23337,#23338),(#23339,#23340),(#23341,#23342),(#23343,#23344),(#23345,
#23346),(#23347,#23348),(#23349,#23350),(#23351,#23352),(#23353,#23354),
(#23355,#23356),(#23357,#23358),(#23359,#23360),(#23361,#23362),(#23363,
#23364),(#23365,#23366),(#23367,#23368),(#23369,#23370),(#23371,#23372),
(#23373,#23374),(#23375,#23376),(#23377,#23378),(#23379,#23380),(#23381,
#23382),(#23383,#23384),(#23385,#23386),(#23387,#23388),(#23389,#23390),
(#23391,#23392),(#23393,#23394),(#23395,#23396),(#23397,#23398),(#23399,
#23400),(#23401,#23402),(#23403,#23404),(#23405,#23406),(#23407,#23408),
(#23409,#23410),(#23411,#23412),(#23413,#23414),(#23415,#23416),(#23417,
#23418),(#23419,#23420),(#23421,#23422),(#23423,#23424),(#23425,#23426),
(#23427,#23428),(#23429,#23430),(#23431,#23432),(#23433,#23434),(#23435,
#23436),(#23437,#23438),(#23439,#23440),(#23441,#23442)),.UNSPECIFIED.,
 .F.,.F.,.F.)
B_SPLINE_SURFACE_WITH_KNOTS((6,1,1,1,1,1,1,1,1,1,1,1,1,1,1,1,1,1,1,1,1,
1,1,1,1,1,1,1,1,1,1,1,1,1,1,1,1,1,1,1,1,1,1,1,1,1,1,1,1,1,1,1,1,1,1,1,1,
1,1,1,1,1,1,1,1,6),(2,2),(-1.,-0.984615384615383,-0.969230769230768,-0.953846153846152,
-0.938461538461537,-0.923076923076922,-0.907692307692306,-0.892307692307691,
-0.876923076923076,-0.86153846153846,-0.846153846153845,-0.83076923076923,
-0.815384615384614,-0.799999999999999,-0.784615384615384,-0.769230769230768,
-0.753846153846153,-0.738461538461538,-0.723076923076922,-0.707692307692307,
-0.692307692307692,-0.676923076923076,-0.661538461538461,-0.646153846153846,
-0.63076923076923,-0.615384615384615,-0.6,-0.584615384615384,-0.569230769230769,
-0.553846153846154,-0.538461538461538,-0.523076923076923,-0.507692307692308,
-0.492307692307692,-0.476923076923077,-0.461538461538462,-0.446153846153846,
-0.430769230769231,-0.415384615384615,-0.4,-0.384615384615385,-0.369230769230769,
-0.353846153846154,-0.338461538461538,-0.323076923076923,-0.307692307692308,
-0.292307692307692,-0.276923076923077,-0.261538461538462,-0.246153846153846,
-0.230769230769231,-0.215384615384615,-0.2,-0.184615384615385,-0.169230769230769,
-0.153846153846154,-0.138461538461538,-0.123076923076923,-0.107692307692308,
-0.0923076923076923,-0.0769230769230769,-0.0615384615384615,-0.0461538461538462,
-0.0307692307692308,-0.0153846153846154,0.),(-1.,1.),.UNSPECIFIED.)
GEOMETRIC_REPRESENTATION_ITEM()
RATIONAL_B_SPLINE_SURFACE(((1.,1.),(1.,1.),(1.,1.),(1.,1.),(1.,1.),(1.,
1.),(1.,1.),(1.,1.),(1.,1.),(1.,1.),(1.,1.),(1.,1.),(1.,1.),(1.,1.),(1.,
1.),(1.,1.),(1.,1.),(1.,1.),(1.,1.),(1.,1.),(1.,1.),(1.,1.),(1.,1.),(1.,
1.),(1.,1.),(1.,1.),(1.,1.),(1.,1.),(1.,1.),(1.,1.),(1.,1.),(1.,1.),(1.,
1.),(1.,1.),(1.,1.),(1.,1.),(1.,1.),(1.,1.),(1.,1.),(1.,1.),(1.,1.),(1.,
1.),(1.,1.),(1.,1.),(1.,1.),(1.,1.),(1.,1.),(1.,1.),(1.,1.),(1.,1.),(1.,
1.),(1.,1.),(1.,1.),(1.,1.),(1.,1.),(1.,1.),(1.,1.),(1.,1.),(1.,1.),(1.,
1.),(1.,1.),(1.,1.),(1.,1.),(1.,1.),(1.,1.),(1.,1.),(1.,1.),(1.,1.),(1.,
1.),(1.,1.)))
REPRESENTATION_ITEM('')
SURFACE()
);
#22=(
BOUNDED_SURFACE()
B_SPLINE_SURFACE(5,1,((#23519,#23520),(#23521,#23522),(#23523,#23524),(#23525,
#23526),(#23527,#23528),(#23529,#23530),(#23531,#23532),(#23533,#23534),
(#23535,#23536),(#23537,#23538),(#23539,#23540),(#23541,#23542),(#23543,
#23544),(#23545,#23546),(#23547,#23548),(#23549,#23550),(#23551,#23552),
(#23553,#23554),(#23555,#23556),(#23557,#23558),(#23559,#23560),(#23561,
#23562),(#23563,#23564),(#23565,#23566),(#23567,#23568),(#23569,#23570),
(#23571,#23572),(#23573,#23574),(#23575,#23576),(#23577,#23578),(#23579,
#23580),(#23581,#23582),(#23583,#23584),(#23585,#23586),(#23587,#23588),
(#23589,#23590),(#23591,#23592),(#23593,#23594),(#23595,#23596),(#23597,
#23598),(#23599,#23600),(#23601,#23602),(#23603,#23604),(#23605,#23606),
(#23607,#23608),(#23609,#23610),(#23611,#23612),(#23613,#23614),(#23615,
#23616),(#23617,#23618),(#23619,#23620),(#23621,#23622),(#23623,#23624),
(#23625,#23626),(#23627,#23628),(#23629,#23630),(#23631,#23632),(#23633,
#23634),(#23635,#23636),(#23637,#23638),(#23639,#23640),(#23641,#23642),
(#23643,#23644),(#23645,#23646),(#23647,#23648),(#23649,#23650),(#23651,
#23652),(#23653,#23654),(#23655,#23656),(#23657,#23658)),.UNSPECIFIED.,
 .F.,.F.,.F.)
B_SPLINE_SURFACE_WITH_KNOTS((6,1,1,1,1,1,1,1,1,1,1,1,1,1,1,1,1,1,1,1,1,
1,1,1,1,1,1,1,1,1,1,1,1,1,1,1,1,1,1,1,1,1,1,1,1,1,1,1,1,1,1,1,1,1,1,1,1,
1,1,1,1,1,1,1,1,6),(2,2),(-1.,-0.984615384615383,-0.969230769230768,-0.953846153846152,
-0.938461538461537,-0.923076923076922,-0.907692307692306,-0.892307692307691,
-0.876923076923076,-0.86153846153846,-0.846153846153845,-0.83076923076923,
-0.815384615384614,-0.799999999999999,-0.784615384615384,-0.769230769230768,
-0.753846153846153,-0.738461538461538,-0.723076923076922,-0.707692307692307,
-0.692307692307692,-0.676923076923076,-0.661538461538461,-0.646153846153846,
-0.63076923076923,-0.615384615384615,-0.6,-0.584615384615384,-0.569230769230769,
-0.553846153846154,-0.538461538461538,-0.523076923076923,-0.507692307692308,
-0.492307692307692,-0.476923076923077,-0.461538461538462,-0.446153846153846,
-0.430769230769231,-0.415384615384615,-0.4,-0.384615384615385,-0.369230769230769,
-0.353846153846154,-0.338461538461538,-0.323076923076923,-0.307692307692308,
-0.292307692307692,-0.276923076923077,-0.261538461538462,-0.246153846153846,
-0.230769230769231,-0.215384615384615,-0.2,-0.184615384615385,-0.169230769230769,
-0.153846153846154,-0.138461538461538,-0.123076923076923,-0.107692307692308,
-0.0923076923076923,-0.0769230769230769,-0.0615384615384615,-0.0461538461538462,
-0.0307692307692308,-0.0153846153846154,0.),(-1.,1.),.UNSPECIFIED.)
GEOMETRIC_REPRESENTATION_ITEM()
RATIONAL_B_SPLINE_SURFACE(((1.,1.),(1.,1.),(1.,1.),(1.,1.),(1.,1.),(1.,
1.),(1.,1.),(1.,1.),(1.,1.),(1.,1.),(1.,1.),(1.,1.),(1.,1.),(1.,1.),(1.,
1.),(1.,1.),(1.,1.),(1.,1.),(1.,1.),(1.,1.),(1.,1.),(1.,1.),(1.,1.),(1.,
1.),(1.,1.),(1.,1.),(1.,1.),(1.,1.),(1.,1.),(1.,1.),(1.,1.),(1.,1.),(1.,
1.),(1.,1.),(1.,1.),(1.,1.),(1.,1.),(1.,1.),(1.,1.),(1.,1.),(1.,1.),(1.,
1.),(1.,1.),(1.,1.),(1.,1.),(1.,1.),(1.,1.),(1.,1.),(1.,1.),(1.,1.),(1.,
1.),(1.,1.),(1.,1.),(1.,1.),(1.,1.),(1.,1.),(1.,1.),(1.,1.),(1.,1.),(1.,
1.),(1.,1.),(1.,1.),(1.,1.),(1.,1.),(1.,1.),(1.,1.),(1.,1.),(1.,1.),(1.,
1.),(1.,1.)))
REPRESENTATION_ITEM('')
SURFACE()
);
#23=(
BOUNDED_SURFACE()
B_SPLINE_SURFACE(5,1,((#23735,#23736),(#23737,#23738),(#23739,#23740),(#23741,
#23742),(#23743,#23744),(#23745,#23746),(#23747,#23748),(#23749,#23750),
(#23751,#23752),(#23753,#23754),(#23755,#23756),(#23757,#23758),(#23759,
#23760),(#23761,#23762),(#23763,#23764),(#23765,#23766),(#23767,#23768),
(#23769,#23770),(#23771,#23772),(#23773,#23774),(#23775,#23776),(#23777,
#23778),(#23779,#23780),(#23781,#23782),(#23783,#23784),(#23785,#23786),
(#23787,#23788),(#23789,#23790),(#23791,#23792),(#23793,#23794),(#23795,
#23796),(#23797,#23798),(#23799,#23800),(#23801,#23802),(#23803,#23804),
(#23805,#23806),(#23807,#23808),(#23809,#23810),(#23811,#23812),(#23813,
#23814),(#23815,#23816),(#23817,#23818),(#23819,#23820),(#23821,#23822),
(#23823,#23824),(#23825,#23826),(#23827,#23828),(#23829,#23830),(#23831,
#23832),(#23833,#23834),(#23835,#23836),(#23837,#23838),(#23839,#23840),
(#23841,#23842),(#23843,#23844),(#23845,#23846),(#23847,#23848),(#23849,
#23850),(#23851,#23852),(#23853,#23854),(#23855,#23856),(#23857,#23858),
(#23859,#23860),(#23861,#23862),(#23863,#23864),(#23865,#23866),(#23867,
#23868),(#23869,#23870),(#23871,#23872),(#23873,#23874)),.UNSPECIFIED.,
 .F.,.F.,.F.)
B_SPLINE_SURFACE_WITH_KNOTS((6,1,1,1,1,1,1,1,1,1,1,1,1,1,1,1,1,1,1,1,1,
1,1,1,1,1,1,1,1,1,1,1,1,1,1,1,1,1,1,1,1,1,1,1,1,1,1,1,1,1,1,1,1,1,1,1,1,
1,1,1,1,1,1,1,1,6),(2,2),(-1.,-0.984615384615383,-0.969230769230768,-0.953846153846152,
-0.938461538461537,-0.923076923076922,-0.907692307692306,-0.892307692307691,
-0.876923076923076,-0.86153846153846,-0.846153846153845,-0.83076923076923,
-0.815384615384614,-0.799999999999999,-0.784615384615384,-0.769230769230768,
-0.753846153846153,-0.738461538461538,-0.723076923076922,-0.707692307692307,
-0.692307692307692,-0.676923076923076,-0.661538461538461,-0.646153846153846,
-0.63076923076923,-0.615384615384615,-0.6,-0.584615384615384,-0.569230769230769,
-0.553846153846154,-0.538461538461538,-0.523076923076923,-0.507692307692308,
-0.492307692307692,-0.476923076923077,-0.461538461538462,-0.446153846153846,
-0.430769230769231,-0.415384615384615,-0.4,-0.384615384615385,-0.369230769230769,
-0.353846153846154,-0.338461538461538,-0.323076923076923,-0.307692307692308,
-0.292307692307692,-0.276923076923077,-0.261538461538462,-0.246153846153846,
-0.230769230769231,-0.215384615384615,-0.2,-0.184615384615385,-0.169230769230769,
-0.153846153846154,-0.138461538461538,-0.123076923076923,-0.107692307692308,
-0.0923076923076923,-0.0769230769230769,-0.0615384615384615,-0.0461538461538462,
-0.0307692307692308,-0.0153846153846154,0.),(-1.,1.),.UNSPECIFIED.)
GEOMETRIC_REPRESENTATION_ITEM()
RATIONAL_B_SPLINE_SURFACE(((1.,1.),(1.,1.),(1.,1.),(1.,1.),(1.,1.),(1.,
1.),(1.,1.),(1.,1.),(1.,1.),(1.,1.),(1.,1.),(1.,1.),(1.,1.),(1.,1.),(1.,
1.),(1.,1.),(1.,1.),(1.,1.),(1.,1.),(1.,1.),(1.,1.),(1.,1.),(1.,1.),(1.,
1.),(1.,1.),(1.,1.),(1.,1.),(1.,1.),(1.,1.),(1.,1.),(1.,1.),(1.,1.),(1.,
1.),(1.,1.),(1.,1.),(1.,1.),(1.,1.),(1.,1.),(1.,1.),(1.,1.),(1.,1.),(1.,
1.),(1.,1.),(1.,1.),(1.,1.),(1.,1.),(1.,1.),(1.,1.),(1.,1.),(1.,1.),(1.,
1.),(1.,1.),(1.,1.),(1.,1.),(1.,1.),(1.,1.),(1.,1.),(1.,1.),(1.,1.),(1.,
1.),(1.,1.),(1.,1.),(1.,1.),(1.,1.),(1.,1.),(1.,1.),(1.,1.),(1.,1.),(1.,
1.),(1.,1.)))
REPRESENTATION_ITEM('')
SURFACE()
);
#24=(
BOUNDED_SURFACE()
B_SPLINE_SURFACE(5,1,((#23951,#23952),(#23953,#23954),(#23955,#23956),(#23957,
#23958),(#23959,#23960),(#23961,#23962),(#23963,#23964),(#23965,#23966),
(#23967,#23968),(#23969,#23970),(#23971,#23972),(#23973,#23974),(#23975,
#23976),(#23977,#23978),(#23979,#23980),(#23981,#23982),(#23983,#23984),
(#23985,#23986),(#23987,#23988),(#23989,#23990),(#23991,#23992),(#23993,
#23994),(#23995,#23996),(#23997,#23998),(#23999,#24000),(#24001,#24002),
(#24003,#24004),(#24005,#24006),(#24007,#24008),(#24009,#24010),(#24011,
#24012),(#24013,#24014),(#24015,#24016),(#24017,#24018),(#24019,#24020),
(#24021,#24022),(#24023,#24024),(#24025,#24026),(#24027,#24028),(#24029,
#24030),(#24031,#24032),(#24033,#24034),(#24035,#24036),(#24037,#24038),
(#24039,#24040),(#24041,#24042),(#24043,#24044),(#24045,#24046),(#24047,
#24048),(#24049,#24050),(#24051,#24052),(#24053,#24054),(#24055,#24056),
(#24057,#24058),(#24059,#24060),(#24061,#24062),(#24063,#24064),(#24065,
#24066),(#24067,#24068),(#24069,#24070),(#24071,#24072),(#24073,#24074),
(#24075,#24076),(#24077,#24078),(#24079,#24080),(#24081,#24082),(#24083,
#24084),(#24085,#24086),(#24087,#24088),(#24089,#24090)),.UNSPECIFIED.,
 .F.,.F.,.F.)
B_SPLINE_SURFACE_WITH_KNOTS((6,1,1,1,1,1,1,1,1,1,1,1,1,1,1,1,1,1,1,1,1,
1,1,1,1,1,1,1,1,1,1,1,1,1,1,1,1,1,1,1,1,1,1,1,1,1,1,1,1,1,1,1,1,1,1,1,1,
1,1,1,1,1,1,1,1,6),(2,2),(-1.,-0.984615384615383,-0.969230769230768,-0.953846153846152,
-0.938461538461537,-0.923076923076922,-0.907692307692306,-0.892307692307691,
-0.876923076923076,-0.86153846153846,-0.846153846153845,-0.83076923076923,
-0.815384615384614,-0.799999999999999,-0.784615384615384,-0.769230769230768,
-0.753846153846153,-0.738461538461538,-0.723076923076922,-0.707692307692307,
-0.692307692307692,-0.676923076923076,-0.661538461538461,-0.646153846153846,
-0.63076923076923,-0.615384615384615,-0.6,-0.584615384615384,-0.569230769230769,
-0.553846153846154,-0.538461538461538,-0.523076923076923,-0.507692307692308,
-0.492307692307692,-0.476923076923077,-0.461538461538462,-0.446153846153846,
-0.430769230769231,-0.415384615384615,-0.4,-0.384615384615385,-0.369230769230769,
-0.353846153846154,-0.338461538461538,-0.323076923076923,-0.307692307692308,
-0.292307692307692,-0.276923076923077,-0.261538461538462,-0.246153846153846,
-0.230769230769231,-0.215384615384615,-0.2,-0.184615384615385,-0.169230769230769,
-0.153846153846154,-0.138461538461538,-0.123076923076923,-0.107692307692308,
-0.0923076923076923,-0.0769230769230769,-0.0615384615384615,-0.0461538461538462,
-0.0307692307692308,-0.0153846153846154,0.),(-1.,1.),.UNSPECIFIED.)
GEOMETRIC_REPRESENTATION_ITEM()
RATIONAL_B_SPLINE_SURFACE(((1.,1.),(1.,1.),(1.,1.),(1.,1.),(1.,1.),(1.,
1.),(1.,1.),(1.,1.),(1.,1.),(1.,1.),(1.,1.),(1.,1.),(1.,1.),(1.,1.),(1.,
1.),(1.,1.),(1.,1.),(1.,1.),(1.,1.),(1.,1.),(1.,1.),(1.,1.),(1.,1.),(1.,
1.),(1.,1.),(1.,1.),(1.,1.),(1.,1.),(1.,1.),(1.,1.),(1.,1.),(1.,1.),(1.,
1.),(1.,1.),(1.,1.),(1.,1.),(1.,1.),(1.,1.),(1.,1.),(1.,1.),(1.,1.),(1.,
1.),(1.,1.),(1.,1.),(1.,1.),(1.,1.),(1.,1.),(1.,1.),(1.,1.),(1.,1.),(1.,
1.),(1.,1.),(1.,1.),(1.,1.),(1.,1.),(1.,1.),(1.,1.),(1.,1.),(1.,1.),(1.,
1.),(1.,1.),(1.,1.),(1.,1.),(1.,1.),(1.,1.),(1.,1.),(1.,1.),(1.,1.),(1.,
1.),(1.,1.)))
REPRESENTATION_ITEM('')
SURFACE()
);
#25=(
BOUNDED_SURFACE()
B_SPLINE_SURFACE(5,1,((#24167,#24168),(#24169,#24170),(#24171,#24172),(#24173,
#24174),(#24175,#24176),(#24177,#24178),(#24179,#24180),(#24181,#24182),
(#24183,#24184),(#24185,#24186),(#24187,#24188),(#24189,#24190),(#24191,
#24192),(#24193,#24194),(#24195,#24196),(#24197,#24198),(#24199,#24200),
(#24201,#24202),(#24203,#24204),(#24205,#24206),(#24207,#24208),(#24209,
#24210),(#24211,#24212),(#24213,#24214),(#24215,#24216),(#24217,#24218),
(#24219,#24220),(#24221,#24222),(#24223,#24224),(#24225,#24226),(#24227,
#24228),(#24229,#24230),(#24231,#24232),(#24233,#24234),(#24235,#24236),
(#24237,#24238),(#24239,#24240),(#24241,#24242),(#24243,#24244),(#24245,
#24246),(#24247,#24248),(#24249,#24250),(#24251,#24252),(#24253,#24254),
(#24255,#24256),(#24257,#24258),(#24259,#24260),(#24261,#24262),(#24263,
#24264),(#24265,#24266),(#24267,#24268),(#24269,#24270),(#24271,#24272),
(#24273,#24274),(#24275,#24276),(#24277,#24278),(#24279,#24280),(#24281,
#24282),(#24283,#24284),(#24285,#24286),(#24287,#24288),(#24289,#24290),
(#24291,#24292),(#24293,#24294),(#24295,#24296),(#24297,#24298),(#24299,
#24300),(#24301,#24302),(#24303,#24304),(#24305,#24306)),.UNSPECIFIED.,
 .F.,.F.,.F.)
B_SPLINE_SURFACE_WITH_KNOTS((6,1,1,1,1,1,1,1,1,1,1,1,1,1,1,1,1,1,1,1,1,
1,1,1,1,1,1,1,1,1,1,1,1,1,1,1,1,1,1,1,1,1,1,1,1,1,1,1,1,1,1,1,1,1,1,1,1,
1,1,1,1,1,1,1,1,6),(2,2),(-1.,-0.984615384615383,-0.969230769230768,-0.953846153846152,
-0.938461538461537,-0.923076923076922,-0.907692307692306,-0.892307692307691,
-0.876923076923076,-0.86153846153846,-0.846153846153845,-0.83076923076923,
-0.815384615384614,-0.799999999999999,-0.784615384615384,-0.769230769230768,
-0.753846153846153,-0.738461538461538,-0.723076923076922,-0.707692307692307,
-0.692307692307692,-0.676923076923076,-0.661538461538461,-0.646153846153846,
-0.63076923076923,-0.615384615384615,-0.6,-0.584615384615384,-0.569230769230769,
-0.553846153846154,-0.538461538461538,-0.523076923076923,-0.507692307692308,
-0.492307692307692,-0.476923076923077,-0.461538461538462,-0.446153846153846,
-0.430769230769231,-0.415384615384615,-0.4,-0.384615384615385,-0.369230769230769,
-0.353846153846154,-0.338461538461538,-0.323076923076923,-0.307692307692308,
-0.292307692307692,-0.276923076923077,-0.261538461538462,-0.246153846153846,
-0.230769230769231,-0.215384615384615,-0.2,-0.184615384615385,-0.169230769230769,
-0.153846153846154,-0.138461538461538,-0.123076923076923,-0.107692307692308,
-0.0923076923076923,-0.0769230769230769,-0.0615384615384615,-0.0461538461538462,
-0.0307692307692308,-0.0153846153846154,0.),(-1.,1.),.UNSPECIFIED.)
GEOMETRIC_REPRESENTATION_ITEM()
RATIONAL_B_SPLINE_SURFACE(((1.,1.),(1.,1.),(1.,1.),(1.,1.),(1.,1.),(1.,
1.),(1.,1.),(1.,1.),(1.,1.),(1.,1.),(1.,1.),(1.,1.),(1.,1.),(1.,1.),(1.,
1.),(1.,1.),(1.,1.),(1.,1.),(1.,1.),(1.,1.),(1.,1.),(1.,1.),(1.,1.),(1.,
1.),(1.,1.),(1.,1.),(1.,1.),(1.,1.),(1.,1.),(1.,1.),(1.,1.),(1.,1.),(1.,
1.),(1.,1.),(1.,1.),(1.,1.),(1.,1.),(1.,1.),(1.,1.),(1.,1.),(1.,1.),(1.,
1.),(1.,1.),(1.,1.),(1.,1.),(1.,1.),(1.,1.),(1.,1.),(1.,1.),(1.,1.),(1.,
1.),(1.,1.),(1.,1.),(1.,1.),(1.,1.),(1.,1.),(1.,1.),(1.,1.),(1.,1.),(1.,
1.),(1.,1.),(1.,1.),(1.,1.),(1.,1.),(1.,1.),(1.,1.),(1.,1.),(1.,1.),(1.,
1.),(1.,1.)))
REPRESENTATION_ITEM('')
SURFACE()
);
#26=(
BOUNDED_SURFACE()
B_SPLINE_SURFACE(5,1,((#24383,#24384),(#24385,#24386),(#24387,#24388),(#24389,
#24390),(#24391,#24392),(#24393,#24394),(#24395,#24396),(#24397,#24398),
(#24399,#24400),(#24401,#24402),(#24403,#24404),(#24405,#24406),(#24407,
#24408),(#24409,#24410),(#24411,#24412),(#24413,#24414),(#24415,#24416),
(#24417,#24418),(#24419,#24420),(#24421,#24422),(#24423,#24424),(#24425,
#24426),(#24427,#24428),(#24429,#24430),(#24431,#24432),(#24433,#24434),
(#24435,#24436),(#24437,#24438),(#24439,#24440),(#24441,#24442),(#24443,
#24444),(#24445,#24446),(#24447,#24448),(#24449,#24450),(#24451,#24452),
(#24453,#24454),(#24455,#24456),(#24457,#24458),(#24459,#24460),(#24461,
#24462),(#24463,#24464),(#24465,#24466),(#24467,#24468),(#24469,#24470),
(#24471,#24472),(#24473,#24474),(#24475,#24476),(#24477,#24478),(#24479,
#24480),(#24481,#24482),(#24483,#24484),(#24485,#24486),(#24487,#24488),
(#24489,#24490),(#24491,#24492),(#24493,#24494),(#24495,#24496),(#24497,
#24498),(#24499,#24500),(#24501,#24502),(#24503,#24504),(#24505,#24506),
(#24507,#24508),(#24509,#24510),(#24511,#24512),(#24513,#24514),(#24515,
#24516),(#24517,#24518),(#24519,#24520),(#24521,#24522)),.UNSPECIFIED.,
 .F.,.F.,.F.)
B_SPLINE_SURFACE_WITH_KNOTS((6,1,1,1,1,1,1,1,1,1,1,1,1,1,1,1,1,1,1,1,1,
1,1,1,1,1,1,1,1,1,1,1,1,1,1,1,1,1,1,1,1,1,1,1,1,1,1,1,1,1,1,1,1,1,1,1,1,
1,1,1,1,1,1,1,1,6),(2,2),(-1.,-0.984615384615383,-0.969230769230768,-0.953846153846152,
-0.938461538461537,-0.923076923076922,-0.907692307692306,-0.892307692307691,
-0.876923076923076,-0.86153846153846,-0.846153846153845,-0.83076923076923,
-0.815384615384614,-0.799999999999999,-0.784615384615384,-0.769230769230768,
-0.753846153846153,-0.738461538461538,-0.723076923076922,-0.707692307692307,
-0.692307692307692,-0.676923076923076,-0.661538461538461,-0.646153846153846,
-0.63076923076923,-0.615384615384615,-0.6,-0.584615384615384,-0.569230769230769,
-0.553846153846154,-0.538461538461538,-0.523076923076923,-0.507692307692308,
-0.492307692307692,-0.476923076923077,-0.461538461538462,-0.446153846153846,
-0.430769230769231,-0.415384615384615,-0.4,-0.384615384615385,-0.369230769230769,
-0.353846153846154,-0.338461538461538,-0.323076923076923,-0.307692307692308,
-0.292307692307692,-0.276923076923077,-0.261538461538462,-0.246153846153846,
-0.230769230769231,-0.215384615384615,-0.2,-0.184615384615385,-0.169230769230769,
-0.153846153846154,-0.138461538461538,-0.123076923076923,-0.107692307692308,
-0.0923076923076923,-0.0769230769230769,-0.0615384615384615,-0.0461538461538462,
-0.0307692307692308,-0.0153846153846154,0.),(-1.,1.),.UNSPECIFIED.)
GEOMETRIC_REPRESENTATION_ITEM()
RATIONAL_B_SPLINE_SURFACE(((1.,1.),(1.,1.),(1.,1.),(1.,1.),(1.,1.),(1.,
1.),(1.,1.),(1.,1.),(1.,1.),(1.,1.),(1.,1.),(1.,1.),(1.,1.),(1.,1.),(1.,
1.),(1.,1.),(1.,1.),(1.,1.),(1.,1.),(1.,1.),(1.,1.),(1.,1.),(1.,1.),(1.,
1.),(1.,1.),(1.,1.),(1.,1.),(1.,1.),(1.,1.),(1.,1.),(1.,1.),(1.,1.),(1.,
1.),(1.,1.),(1.,1.),(1.,1.),(1.,1.),(1.,1.),(1.,1.),(1.,1.),(1.,1.),(1.,
1.),(1.,1.),(1.,1.),(1.,1.),(1.,1.),(1.,1.),(1.,1.),(1.,1.),(1.,1.),(1.,
1.),(1.,1.),(1.,1.),(1.,1.),(1.,1.),(1.,1.),(1.,1.),(1.,1.),(1.,1.),(1.,
1.),(1.,1.),(1.,1.),(1.,1.),(1.,1.),(1.,1.),(1.,1.),(1.,1.),(1.,1.),(1.,
1.),(1.,1.)))
REPRESENTATION_ITEM('')
SURFACE()
);
#27=(
BOUNDED_SURFACE()
B_SPLINE_SURFACE(5,1,((#24599,#24600),(#24601,#24602),(#24603,#24604),(#24605,
#24606),(#24607,#24608),(#24609,#24610),(#24611,#24612),(#24613,#24614),
(#24615,#24616),(#24617,#24618),(#24619,#24620),(#24621,#24622),(#24623,
#24624),(#24625,#24626),(#24627,#24628),(#24629,#24630),(#24631,#24632),
(#24633,#24634),(#24635,#24636),(#24637,#24638),(#24639,#24640),(#24641,
#24642),(#24643,#24644),(#24645,#24646),(#24647,#24648),(#24649,#24650),
(#24651,#24652),(#24653,#24654),(#24655,#24656),(#24657,#24658),(#24659,
#24660),(#24661,#24662),(#24663,#24664),(#24665,#24666),(#24667,#24668),
(#24669,#24670),(#24671,#24672),(#24673,#24674),(#24675,#24676),(#24677,
#24678),(#24679,#24680),(#24681,#24682),(#24683,#24684),(#24685,#24686),
(#24687,#24688),(#24689,#24690),(#24691,#24692),(#24693,#24694),(#24695,
#24696),(#24697,#24698),(#24699,#24700),(#24701,#24702),(#24703,#24704),
(#24705,#24706),(#24707,#24708),(#24709,#24710),(#24711,#24712),(#24713,
#24714),(#24715,#24716),(#24717,#24718),(#24719,#24720),(#24721,#24722),
(#24723,#24724),(#24725,#24726),(#24727,#24728),(#24729,#24730),(#24731,
#24732),(#24733,#24734),(#24735,#24736),(#24737,#24738)),.UNSPECIFIED.,
 .F.,.F.,.F.)
B_SPLINE_SURFACE_WITH_KNOTS((6,1,1,1,1,1,1,1,1,1,1,1,1,1,1,1,1,1,1,1,1,
1,1,1,1,1,1,1,1,1,1,1,1,1,1,1,1,1,1,1,1,1,1,1,1,1,1,1,1,1,1,1,1,1,1,1,1,
1,1,1,1,1,1,1,1,6),(2,2),(-1.,-0.984615384615383,-0.969230769230768,-0.953846153846152,
-0.938461538461537,-0.923076923076922,-0.907692307692306,-0.892307692307691,
-0.876923076923076,-0.86153846153846,-0.846153846153845,-0.83076923076923,
-0.815384615384614,-0.799999999999999,-0.784615384615384,-0.769230769230768,
-0.753846153846153,-0.738461538461538,-0.723076923076922,-0.707692307692307,
-0.692307692307692,-0.676923076923076,-0.661538461538461,-0.646153846153846,
-0.63076923076923,-0.615384615384615,-0.6,-0.584615384615384,-0.569230769230769,
-0.553846153846154,-0.538461538461538,-0.523076923076923,-0.507692307692308,
-0.492307692307692,-0.476923076923077,-0.461538461538462,-0.446153846153846,
-0.430769230769231,-0.415384615384615,-0.4,-0.384615384615385,-0.369230769230769,
-0.353846153846154,-0.338461538461538,-0.323076923076923,-0.307692307692308,
-0.292307692307692,-0.276923076923077,-0.261538461538462,-0.246153846153846,
-0.230769230769231,-0.215384615384615,-0.2,-0.184615384615385,-0.169230769230769,
-0.153846153846154,-0.138461538461538,-0.123076923076923,-0.107692307692308,
-0.0923076923076923,-0.0769230769230769,-0.0615384615384615,-0.0461538461538462,
-0.0307692307692308,-0.0153846153846154,0.),(-1.,1.),.UNSPECIFIED.)
GEOMETRIC_REPRESENTATION_ITEM()
RATIONAL_B_SPLINE_SURFACE(((1.,1.),(1.,1.),(1.,1.),(1.,1.),(1.,1.),(1.,
1.),(1.,1.),(1.,1.),(1.,1.),(1.,1.),(1.,1.),(1.,1.),(1.,1.),(1.,1.),(1.,
1.),(1.,1.),(1.,1.),(1.,1.),(1.,1.),(1.,1.),(1.,1.),(1.,1.),(1.,1.),(1.,
1.),(1.,1.),(1.,1.),(1.,1.),(1.,1.),(1.,1.),(1.,1.),(1.,1.),(1.,1.),(1.,
1.),(1.,1.),(1.,1.),(1.,1.),(1.,1.),(1.,1.),(1.,1.),(1.,1.),(1.,1.),(1.,
1.),(1.,1.),(1.,1.),(1.,1.),(1.,1.),(1.,1.),(1.,1.),(1.,1.),(1.,1.),(1.,
1.),(1.,1.),(1.,1.),(1.,1.),(1.,1.),(1.,1.),(1.,1.),(1.,1.),(1.,1.),(1.,
1.),(1.,1.),(1.,1.),(1.,1.),(1.,1.),(1.,1.),(1.,1.),(1.,1.),(1.,1.),(1.,
1.),(1.,1.)))
REPRESENTATION_ITEM('')
SURFACE()
);
#28=(
BOUNDED_SURFACE()
B_SPLINE_SURFACE(5,1,((#24815,#24816),(#24817,#24818),(#24819,#24820),(#24821,
#24822),(#24823,#24824),(#24825,#24826),(#24827,#24828),(#24829,#24830),
(#24831,#24832),(#24833,#24834),(#24835,#24836),(#24837,#24838),(#24839,
#24840),(#24841,#24842),(#24843,#24844),(#24845,#24846),(#24847,#24848),
(#24849,#24850),(#24851,#24852),(#24853,#24854),(#24855,#24856),(#24857,
#24858),(#24859,#24860),(#24861,#24862),(#24863,#24864),(#24865,#24866),
(#24867,#24868),(#24869,#24870),(#24871,#24872),(#24873,#24874),(#24875,
#24876),(#24877,#24878),(#24879,#24880),(#24881,#24882),(#24883,#24884),
(#24885,#24886),(#24887,#24888),(#24889,#24890),(#24891,#24892),(#24893,
#24894),(#24895,#24896),(#24897,#24898),(#24899,#24900),(#24901,#24902),
(#24903,#24904),(#24905,#24906),(#24907,#24908),(#24909,#24910),(#24911,
#24912),(#24913,#24914),(#24915,#24916),(#24917,#24918),(#24919,#24920),
(#24921,#24922),(#24923,#24924),(#24925,#24926),(#24927,#24928),(#24929,
#24930),(#24931,#24932),(#24933,#24934),(#24935,#24936),(#24937,#24938),
(#24939,#24940),(#24941,#24942),(#24943,#24944),(#24945,#24946),(#24947,
#24948),(#24949,#24950),(#24951,#24952),(#24953,#24954)),.UNSPECIFIED.,
 .F.,.F.,.F.)
B_SPLINE_SURFACE_WITH_KNOTS((6,1,1,1,1,1,1,1,1,1,1,1,1,1,1,1,1,1,1,1,1,
1,1,1,1,1,1,1,1,1,1,1,1,1,1,1,1,1,1,1,1,1,1,1,1,1,1,1,1,1,1,1,1,1,1,1,1,
1,1,1,1,1,1,1,1,6),(2,2),(-1.,-0.984615384615383,-0.969230769230768,-0.953846153846152,
-0.938461538461537,-0.923076923076922,-0.907692307692306,-0.892307692307691,
-0.876923076923076,-0.86153846153846,-0.846153846153845,-0.83076923076923,
-0.815384615384614,-0.799999999999999,-0.784615384615384,-0.769230769230768,
-0.753846153846153,-0.738461538461538,-0.723076923076922,-0.707692307692307,
-0.692307692307692,-0.676923076923076,-0.661538461538461,-0.646153846153846,
-0.63076923076923,-0.615384615384615,-0.6,-0.584615384615384,-0.569230769230769,
-0.553846153846154,-0.538461538461538,-0.523076923076923,-0.507692307692308,
-0.492307692307692,-0.476923076923077,-0.461538461538462,-0.446153846153846,
-0.430769230769231,-0.415384615384615,-0.4,-0.384615384615385,-0.369230769230769,
-0.353846153846154,-0.338461538461538,-0.323076923076923,-0.307692307692308,
-0.292307692307692,-0.276923076923077,-0.261538461538462,-0.246153846153846,
-0.230769230769231,-0.215384615384615,-0.2,-0.184615384615385,-0.169230769230769,
-0.153846153846154,-0.138461538461538,-0.123076923076923,-0.107692307692308,
-0.0923076923076923,-0.0769230769230769,-0.0615384615384615,-0.0461538461538462,
-0.0307692307692308,-0.0153846153846154,0.),(-1.,1.),.UNSPECIFIED.)
GEOMETRIC_REPRESENTATION_ITEM()
RATIONAL_B_SPLINE_SURFACE(((1.,1.),(1.,1.),(1.,1.),(1.,1.),(1.,1.),(1.,
1.),(1.,1.),(1.,1.),(1.,1.),(1.,1.),(1.,1.),(1.,1.),(1.,1.),(1.,1.),(1.,
1.),(1.,1.),(1.,1.),(1.,1.),(1.,1.),(1.,1.),(1.,1.),(1.,1.),(1.,1.),(1.,
1.),(1.,1.),(1.,1.),(1.,1.),(1.,1.),(1.,1.),(1.,1.),(1.,1.),(1.,1.),(1.,
1.),(1.,1.),(1.,1.),(1.,1.),(1.,1.),(1.,1.),(1.,1.),(1.,1.),(1.,1.),(1.,
1.),(1.,1.),(1.,1.),(1.,1.),(1.,1.),(1.,1.),(1.,1.),(1.,1.),(1.,1.),(1.,
1.),(1.,1.),(1.,1.),(1.,1.),(1.,1.),(1.,1.),(1.,1.),(1.,1.),(1.,1.),(1.,
1.),(1.,1.),(1.,1.),(1.,1.),(1.,1.),(1.,1.),(1.,1.),(1.,1.),(1.,1.),(1.,
1.),(1.,1.)))
REPRESENTATION_ITEM('')
SURFACE()
);
#29=(
BOUNDED_SURFACE()
B_SPLINE_SURFACE(5,1,((#25031,#25032),(#25033,#25034),(#25035,#25036),(#25037,
#25038),(#25039,#25040),(#25041,#25042),(#25043,#25044),(#25045,#25046),
(#25047,#25048),(#25049,#25050),(#25051,#25052),(#25053,#25054),(#25055,
#25056),(#25057,#25058),(#25059,#25060),(#25061,#25062),(#25063,#25064),
(#25065,#25066),(#25067,#25068),(#25069,#25070),(#25071,#25072),(#25073,
#25074),(#25075,#25076),(#25077,#25078),(#25079,#25080),(#25081,#25082),
(#25083,#25084),(#25085,#25086),(#25087,#25088),(#25089,#25090),(#25091,
#25092),(#25093,#25094),(#25095,#25096),(#25097,#25098),(#25099,#25100),
(#25101,#25102),(#25103,#25104),(#25105,#25106),(#25107,#25108),(#25109,
#25110),(#25111,#25112),(#25113,#25114),(#25115,#25116),(#25117,#25118),
(#25119,#25120),(#25121,#25122),(#25123,#25124),(#25125,#25126),(#25127,
#25128),(#25129,#25130),(#25131,#25132),(#25133,#25134),(#25135,#25136),
(#25137,#25138),(#25139,#25140),(#25141,#25142),(#25143,#25144),(#25145,
#25146),(#25147,#25148),(#25149,#25150),(#25151,#25152),(#25153,#25154),
(#25155,#25156),(#25157,#25158),(#25159,#25160),(#25161,#25162),(#25163,
#25164),(#25165,#25166),(#25167,#25168),(#25169,#25170)),.UNSPECIFIED.,
 .F.,.F.,.F.)
B_SPLINE_SURFACE_WITH_KNOTS((6,1,1,1,1,1,1,1,1,1,1,1,1,1,1,1,1,1,1,1,1,
1,1,1,1,1,1,1,1,1,1,1,1,1,1,1,1,1,1,1,1,1,1,1,1,1,1,1,1,1,1,1,1,1,1,1,1,
1,1,1,1,1,1,1,1,6),(2,2),(-1.,-0.984615384615383,-0.969230769230768,-0.953846153846152,
-0.938461538461537,-0.923076923076922,-0.907692307692306,-0.892307692307691,
-0.876923076923076,-0.86153846153846,-0.846153846153845,-0.83076923076923,
-0.815384615384614,-0.799999999999999,-0.784615384615384,-0.769230769230768,
-0.753846153846153,-0.738461538461538,-0.723076923076922,-0.707692307692307,
-0.692307692307692,-0.676923076923076,-0.661538461538461,-0.646153846153846,
-0.63076923076923,-0.615384615384615,-0.6,-0.584615384615384,-0.569230769230769,
-0.553846153846154,-0.538461538461538,-0.523076923076923,-0.507692307692308,
-0.492307692307692,-0.476923076923077,-0.461538461538462,-0.446153846153846,
-0.430769230769231,-0.415384615384615,-0.4,-0.384615384615385,-0.369230769230769,
-0.353846153846154,-0.338461538461538,-0.323076923076923,-0.307692307692308,
-0.292307692307692,-0.276923076923077,-0.261538461538462,-0.246153846153846,
-0.230769230769231,-0.215384615384615,-0.2,-0.184615384615385,-0.169230769230769,
-0.153846153846154,-0.138461538461538,-0.123076923076923,-0.107692307692308,
-0.0923076923076923,-0.0769230769230769,-0.0615384615384615,-0.0461538461538462,
-0.0307692307692308,-0.0153846153846154,0.),(-1.,1.),.UNSPECIFIED.)
GEOMETRIC_REPRESENTATION_ITEM()
RATIONAL_B_SPLINE_SURFACE(((1.,1.),(1.,1.),(1.,1.),(1.,1.),(1.,1.),(1.,
1.),(1.,1.),(1.,1.),(1.,1.),(1.,1.),(1.,1.),(1.,1.),(1.,1.),(1.,1.),(1.,
1.),(1.,1.),(1.,1.),(1.,1.),(1.,1.),(1.,1.),(1.,1.),(1.,1.),(1.,1.),(1.,
1.),(1.,1.),(1.,1.),(1.,1.),(1.,1.),(1.,1.),(1.,1.),(1.,1.),(1.,1.),(1.,
1.),(1.,1.),(1.,1.),(1.,1.),(1.,1.),(1.,1.),(1.,1.),(1.,1.),(1.,1.),(1.,
1.),(1.,1.),(1.,1.),(1.,1.),(1.,1.),(1.,1.),(1.,1.),(1.,1.),(1.,1.),(1.,
1.),(1.,1.),(1.,1.),(1.,1.),(1.,1.),(1.,1.),(1.,1.),(1.,1.),(1.,1.),(1.,
1.),(1.,1.),(1.,1.),(1.,1.),(1.,1.),(1.,1.),(1.,1.),(1.,1.),(1.,1.),(1.,
1.),(1.,1.)))
REPRESENTATION_ITEM('')
SURFACE()
);
#30=(
BOUNDED_SURFACE()
B_SPLINE_SURFACE(5,1,((#25247,#25248),(#25249,#25250),(#25251,#25252),(#25253,
#25254),(#25255,#25256),(#25257,#25258),(#25259,#25260),(#25261,#25262),
(#25263,#25264),(#25265,#25266),(#25267,#25268),(#25269,#25270),(#25271,
#25272),(#25273,#25274),(#25275,#25276),(#25277,#25278),(#25279,#25280),
(#25281,#25282),(#25283,#25284),(#25285,#25286),(#25287,#25288),(#25289,
#25290),(#25291,#25292),(#25293,#25294),(#25295,#25296),(#25297,#25298),
(#25299,#25300),(#25301,#25302),(#25303,#25304),(#25305,#25306),(#25307,
#25308),(#25309,#25310),(#25311,#25312),(#25313,#25314),(#25315,#25316),
(#25317,#25318),(#25319,#25320),(#25321,#25322),(#25323,#25324),(#25325,
#25326),(#25327,#25328),(#25329,#25330),(#25331,#25332),(#25333,#25334),
(#25335,#25336),(#25337,#25338),(#25339,#25340),(#25341,#25342),(#25343,
#25344),(#25345,#25346),(#25347,#25348),(#25349,#25350),(#25351,#25352),
(#25353,#25354),(#25355,#25356),(#25357,#25358),(#25359,#25360),(#25361,
#25362),(#25363,#25364),(#25365,#25366),(#25367,#25368),(#25369,#25370),
(#25371,#25372),(#25373,#25374),(#25375,#25376),(#25377,#25378),(#25379,
#25380),(#25381,#25382),(#25383,#25384),(#25385,#25386)),.UNSPECIFIED.,
 .F.,.F.,.F.)
B_SPLINE_SURFACE_WITH_KNOTS((6,1,1,1,1,1,1,1,1,1,1,1,1,1,1,1,1,1,1,1,1,
1,1,1,1,1,1,1,1,1,1,1,1,1,1,1,1,1,1,1,1,1,1,1,1,1,1,1,1,1,1,1,1,1,1,1,1,
1,1,1,1,1,1,1,1,6),(2,2),(-1.,-0.984615384615383,-0.969230769230768,-0.953846153846152,
-0.938461538461537,-0.923076923076922,-0.907692307692306,-0.892307692307691,
-0.876923076923076,-0.86153846153846,-0.846153846153845,-0.83076923076923,
-0.815384615384614,-0.799999999999999,-0.784615384615384,-0.769230769230768,
-0.753846153846153,-0.738461538461538,-0.723076923076922,-0.707692307692307,
-0.692307692307692,-0.676923076923076,-0.661538461538461,-0.646153846153846,
-0.63076923076923,-0.615384615384615,-0.6,-0.584615384615384,-0.569230769230769,
-0.553846153846154,-0.538461538461538,-0.523076923076923,-0.507692307692308,
-0.492307692307692,-0.476923076923077,-0.461538461538462,-0.446153846153846,
-0.430769230769231,-0.415384615384615,-0.4,-0.384615384615385,-0.369230769230769,
-0.353846153846154,-0.338461538461538,-0.323076923076923,-0.307692307692308,
-0.292307692307692,-0.276923076923077,-0.261538461538462,-0.246153846153846,
-0.230769230769231,-0.215384615384615,-0.2,-0.184615384615385,-0.169230769230769,
-0.153846153846154,-0.138461538461538,-0.123076923076923,-0.107692307692308,
-0.0923076923076923,-0.0769230769230769,-0.0615384615384615,-0.0461538461538462,
-0.0307692307692308,-0.0153846153846154,0.),(-1.,1.),.UNSPECIFIED.)
GEOMETRIC_REPRESENTATION_ITEM()
RATIONAL_B_SPLINE_SURFACE(((1.,1.),(1.,1.),(1.,1.),(1.,1.),(1.,1.),(1.,
1.),(1.,1.),(1.,1.),(1.,1.),(1.,1.),(1.,1.),(1.,1.),(1.,1.),(1.,1.),(1.,
1.),(1.,1.),(1.,1.),(1.,1.),(1.,1.),(1.,1.),(1.,1.),(1.,1.),(1.,1.),(1.,
1.),(1.,1.),(1.,1.),(1.,1.),(1.,1.),(1.,1.),(1.,1.),(1.,1.),(1.,1.),(1.,
1.),(1.,1.),(1.,1.),(1.,1.),(1.,1.),(1.,1.),(1.,1.),(1.,1.),(1.,1.),(1.,
1.),(1.,1.),(1.,1.),(1.,1.),(1.,1.),(1.,1.),(1.,1.),(1.,1.),(1.,1.),(1.,
1.),(1.,1.),(1.,1.),(1.,1.),(1.,1.),(1.,1.),(1.,1.),(1.,1.),(1.,1.),(1.,
1.),(1.,1.),(1.,1.),(1.,1.),(1.,1.),(1.,1.),(1.,1.),(1.,1.),(1.,1.),(1.,
1.),(1.,1.)))
REPRESENTATION_ITEM('')
SURFACE()
);
#31=(
BOUNDED_SURFACE()
B_SPLINE_SURFACE(5,1,((#25463,#25464),(#25465,#25466),(#25467,#25468),(#25469,
#25470),(#25471,#25472),(#25473,#25474),(#25475,#25476),(#25477,#25478),
(#25479,#25480),(#25481,#25482),(#25483,#25484),(#25485,#25486),(#25487,
#25488),(#25489,#25490),(#25491,#25492),(#25493,#25494),(#25495,#25496),
(#25497,#25498),(#25499,#25500),(#25501,#25502),(#25503,#25504),(#25505,
#25506),(#25507,#25508),(#25509,#25510),(#25511,#25512),(#25513,#25514),
(#25515,#25516),(#25517,#25518),(#25519,#25520),(#25521,#25522),(#25523,
#25524),(#25525,#25526),(#25527,#25528),(#25529,#25530),(#25531,#25532),
(#25533,#25534),(#25535,#25536),(#25537,#25538),(#25539,#25540),(#25541,
#25542),(#25543,#25544),(#25545,#25546),(#25547,#25548),(#25549,#25550),
(#25551,#25552),(#25553,#25554),(#25555,#25556),(#25557,#25558),(#25559,
#25560),(#25561,#25562),(#25563,#25564),(#25565,#25566),(#25567,#25568),
(#25569,#25570),(#25571,#25572),(#25573,#25574),(#25575,#25576),(#25577,
#25578),(#25579,#25580),(#25581,#25582),(#25583,#25584),(#25585,#25586),
(#25587,#25588),(#25589,#25590),(#25591,#25592),(#25593,#25594),(#25595,
#25596),(#25597,#25598),(#25599,#25600),(#25601,#25602)),.UNSPECIFIED.,
 .F.,.F.,.F.)
B_SPLINE_SURFACE_WITH_KNOTS((6,1,1,1,1,1,1,1,1,1,1,1,1,1,1,1,1,1,1,1,1,
1,1,1,1,1,1,1,1,1,1,1,1,1,1,1,1,1,1,1,1,1,1,1,1,1,1,1,1,1,1,1,1,1,1,1,1,
1,1,1,1,1,1,1,1,6),(2,2),(-1.,-0.984615384615383,-0.969230769230768,-0.953846153846152,
-0.938461538461537,-0.923076923076922,-0.907692307692306,-0.892307692307691,
-0.876923076923076,-0.86153846153846,-0.846153846153845,-0.83076923076923,
-0.815384615384614,-0.799999999999999,-0.784615384615384,-0.769230769230768,
-0.753846153846153,-0.738461538461538,-0.723076923076922,-0.707692307692307,
-0.692307692307692,-0.676923076923076,-0.661538461538461,-0.646153846153846,
-0.63076923076923,-0.615384615384615,-0.6,-0.584615384615384,-0.569230769230769,
-0.553846153846154,-0.538461538461538,-0.523076923076923,-0.507692307692308,
-0.492307692307692,-0.476923076923077,-0.461538461538462,-0.446153846153846,
-0.430769230769231,-0.415384615384615,-0.4,-0.384615384615385,-0.369230769230769,
-0.353846153846154,-0.338461538461538,-0.323076923076923,-0.307692307692308,
-0.292307692307692,-0.276923076923077,-0.261538461538462,-0.246153846153846,
-0.230769230769231,-0.215384615384615,-0.2,-0.184615384615385,-0.169230769230769,
-0.153846153846154,-0.138461538461538,-0.123076923076923,-0.107692307692308,
-0.0923076923076923,-0.0769230769230769,-0.0615384615384615,-0.0461538461538462,
-0.0307692307692308,-0.0153846153846154,0.),(-1.,1.),.UNSPECIFIED.)
GEOMETRIC_REPRESENTATION_ITEM()
RATIONAL_B_SPLINE_SURFACE(((1.,1.),(1.,1.),(1.,1.),(1.,1.),(1.,1.),(1.,
1.),(1.,1.),(1.,1.),(1.,1.),(1.,1.),(1.,1.),(1.,1.),(1.,1.),(1.,1.),(1.,
1.),(1.,1.),(1.,1.),(1.,1.),(1.,1.),(1.,1.),(1.,1.),(1.,1.),(1.,1.),(1.,
1.),(1.,1.),(1.,1.),(1.,1.),(1.,1.),(1.,1.),(1.,1.),(1.,1.),(1.,1.),(1.,
1.),(1.,1.),(1.,1.),(1.,1.),(1.,1.),(1.,1.),(1.,1.),(1.,1.),(1.,1.),(1.,
1.),(1.,1.),(1.,1.),(1.,1.),(1.,1.),(1.,1.),(1.,1.),(1.,1.),(1.,1.),(1.,
1.),(1.,1.),(1.,1.),(1.,1.),(1.,1.),(1.,1.),(1.,1.),(1.,1.),(1.,1.),(1.,
1.),(1.,1.),(1.,1.),(1.,1.),(1.,1.),(1.,1.),(1.,1.),(1.,1.),(1.,1.),(1.,
1.),(1.,1.)))
REPRESENTATION_ITEM('')
SURFACE()
);
#32=(
BOUNDED_SURFACE()
B_SPLINE_SURFACE(5,1,((#25679,#25680),(#25681,#25682),(#25683,#25684),(#25685,
#25686),(#25687,#25688),(#25689,#25690),(#25691,#25692),(#25693,#25694),
(#25695,#25696),(#25697,#25698),(#25699,#25700),(#25701,#25702),(#25703,
#25704),(#25705,#25706),(#25707,#25708),(#25709,#25710),(#25711,#25712),
(#25713,#25714),(#25715,#25716),(#25717,#25718),(#25719,#25720),(#25721,
#25722),(#25723,#25724),(#25725,#25726),(#25727,#25728),(#25729,#25730),
(#25731,#25732),(#25733,#25734),(#25735,#25736),(#25737,#25738),(#25739,
#25740),(#25741,#25742),(#25743,#25744),(#25745,#25746),(#25747,#25748),
(#25749,#25750),(#25751,#25752),(#25753,#25754),(#25755,#25756),(#25757,
#25758),(#25759,#25760),(#25761,#25762),(#25763,#25764),(#25765,#25766),
(#25767,#25768),(#25769,#25770),(#25771,#25772),(#25773,#25774),(#25775,
#25776),(#25777,#25778),(#25779,#25780),(#25781,#25782),(#25783,#25784),
(#25785,#25786),(#25787,#25788),(#25789,#25790),(#25791,#25792),(#25793,
#25794),(#25795,#25796),(#25797,#25798),(#25799,#25800),(#25801,#25802),
(#25803,#25804),(#25805,#25806),(#25807,#25808),(#25809,#25810),(#25811,
#25812),(#25813,#25814),(#25815,#25816),(#25817,#25818)),.UNSPECIFIED.,
 .F.,.F.,.F.)
B_SPLINE_SURFACE_WITH_KNOTS((6,1,1,1,1,1,1,1,1,1,1,1,1,1,1,1,1,1,1,1,1,
1,1,1,1,1,1,1,1,1,1,1,1,1,1,1,1,1,1,1,1,1,1,1,1,1,1,1,1,1,1,1,1,1,1,1,1,
1,1,1,1,1,1,1,1,6),(2,2),(-1.,-0.984615384615383,-0.969230769230768,-0.953846153846152,
-0.938461538461537,-0.923076923076922,-0.907692307692306,-0.892307692307691,
-0.876923076923076,-0.86153846153846,-0.846153846153845,-0.83076923076923,
-0.815384615384614,-0.799999999999999,-0.784615384615384,-0.769230769230768,
-0.753846153846153,-0.738461538461538,-0.723076923076922,-0.707692307692307,
-0.692307692307692,-0.676923076923076,-0.661538461538461,-0.646153846153846,
-0.63076923076923,-0.615384615384615,-0.6,-0.584615384615384,-0.569230769230769,
-0.553846153846154,-0.538461538461538,-0.523076923076923,-0.507692307692308,
-0.492307692307692,-0.476923076923077,-0.461538461538462,-0.446153846153846,
-0.430769230769231,-0.415384615384615,-0.4,-0.384615384615385,-0.369230769230769,
-0.353846153846154,-0.338461538461538,-0.323076923076923,-0.307692307692308,
-0.292307692307692,-0.276923076923077,-0.261538461538462,-0.246153846153846,
-0.230769230769231,-0.215384615384615,-0.2,-0.184615384615385,-0.169230769230769,
-0.153846153846154,-0.138461538461538,-0.123076923076923,-0.107692307692308,
-0.0923076923076923,-0.0769230769230769,-0.0615384615384615,-0.0461538461538462,
-0.0307692307692308,-0.0153846153846154,0.),(-1.,1.),.UNSPECIFIED.)
GEOMETRIC_REPRESENTATION_ITEM()
RATIONAL_B_SPLINE_SURFACE(((1.,1.),(1.,1.),(1.,1.),(1.,1.),(1.,1.),(1.,
1.),(1.,1.),(1.,1.),(1.,1.),(1.,1.),(1.,1.),(1.,1.),(1.,1.),(1.,1.),(1.,
1.),(1.,1.),(1.,1.),(1.,1.),(1.,1.),(1.,1.),(1.,1.),(1.,1.),(1.,1.),(1.,
1.),(1.,1.),(1.,1.),(1.,1.),(1.,1.),(1.,1.),(1.,1.),(1.,1.),(1.,1.),(1.,
1.),(1.,1.),(1.,1.),(1.,1.),(1.,1.),(1.,1.),(1.,1.),(1.,1.),(1.,1.),(1.,
1.),(1.,1.),(1.,1.),(1.,1.),(1.,1.),(1.,1.),(1.,1.),(1.,1.),(1.,1.),(1.,
1.),(1.,1.),(1.,1.),(1.,1.),(1.,1.),(1.,1.),(1.,1.),(1.,1.),(1.,1.),(1.,
1.),(1.,1.),(1.,1.),(1.,1.),(1.,1.),(1.,1.),(1.,1.),(1.,1.),(1.,1.),(1.,
1.),(1.,1.)))
REPRESENTATION_ITEM('')
SURFACE()
);
#33=(
BOUNDED_SURFACE()
B_SPLINE_SURFACE(5,1,((#25895,#25896),(#25897,#25898),(#25899,#25900),(#25901,
#25902),(#25903,#25904),(#25905,#25906),(#25907,#25908),(#25909,#25910),
(#25911,#25912),(#25913,#25914),(#25915,#25916),(#25917,#25918),(#25919,
#25920),(#25921,#25922),(#25923,#25924),(#25925,#25926),(#25927,#25928),
(#25929,#25930),(#25931,#25932),(#25933,#25934),(#25935,#25936),(#25937,
#25938),(#25939,#25940),(#25941,#25942),(#25943,#25944),(#25945,#25946),
(#25947,#25948),(#25949,#25950),(#25951,#25952),(#25953,#25954),(#25955,
#25956),(#25957,#25958),(#25959,#25960),(#25961,#25962),(#25963,#25964),
(#25965,#25966),(#25967,#25968),(#25969,#25970),(#25971,#25972),(#25973,
#25974),(#25975,#25976),(#25977,#25978),(#25979,#25980),(#25981,#25982),
(#25983,#25984),(#25985,#25986),(#25987,#25988),(#25989,#25990),(#25991,
#25992),(#25993,#25994),(#25995,#25996),(#25997,#25998),(#25999,#26000),
(#26001,#26002),(#26003,#26004),(#26005,#26006),(#26007,#26008),(#26009,
#26010),(#26011,#26012),(#26013,#26014),(#26015,#26016),(#26017,#26018),
(#26019,#26020),(#26021,#26022),(#26023,#26024),(#26025,#26026),(#26027,
#26028),(#26029,#26030),(#26031,#26032),(#26033,#26034)),.UNSPECIFIED.,
 .F.,.F.,.F.)
B_SPLINE_SURFACE_WITH_KNOTS((6,1,1,1,1,1,1,1,1,1,1,1,1,1,1,1,1,1,1,1,1,
1,1,1,1,1,1,1,1,1,1,1,1,1,1,1,1,1,1,1,1,1,1,1,1,1,1,1,1,1,1,1,1,1,1,1,1,
1,1,1,1,1,1,1,1,6),(2,2),(-1.,-0.984615384615383,-0.969230769230768,-0.953846153846152,
-0.938461538461537,-0.923076923076922,-0.907692307692306,-0.892307692307691,
-0.876923076923076,-0.86153846153846,-0.846153846153845,-0.83076923076923,
-0.815384615384614,-0.799999999999999,-0.784615384615384,-0.769230769230768,
-0.753846153846153,-0.738461538461538,-0.723076923076922,-0.707692307692307,
-0.692307692307692,-0.676923076923076,-0.661538461538461,-0.646153846153846,
-0.63076923076923,-0.615384615384615,-0.6,-0.584615384615384,-0.569230769230769,
-0.553846153846154,-0.538461538461538,-0.523076923076923,-0.507692307692308,
-0.492307692307692,-0.476923076923077,-0.461538461538462,-0.446153846153846,
-0.430769230769231,-0.415384615384615,-0.4,-0.384615384615385,-0.369230769230769,
-0.353846153846154,-0.338461538461538,-0.323076923076923,-0.307692307692308,
-0.292307692307692,-0.276923076923077,-0.261538461538462,-0.246153846153846,
-0.230769230769231,-0.215384615384615,-0.2,-0.184615384615385,-0.169230769230769,
-0.153846153846154,-0.138461538461538,-0.123076923076923,-0.107692307692308,
-0.0923076923076923,-0.0769230769230769,-0.0615384615384615,-0.0461538461538462,
-0.0307692307692308,-0.0153846153846154,0.),(-1.,1.),.UNSPECIFIED.)
GEOMETRIC_REPRESENTATION_ITEM()
RATIONAL_B_SPLINE_SURFACE(((1.,1.),(1.,1.),(1.,1.),(1.,1.),(1.,1.),(1.,
1.),(1.,1.),(1.,1.),(1.,1.),(1.,1.),(1.,1.),(1.,1.),(1.,1.),(1.,1.),(1.,
1.),(1.,1.),(1.,1.),(1.,1.),(1.,1.),(1.,1.),(1.,1.),(1.,1.),(1.,1.),(1.,
1.),(1.,1.),(1.,1.),(1.,1.),(1.,1.),(1.,1.),(1.,1.),(1.,1.),(1.,1.),(1.,
1.),(1.,1.),(1.,1.),(1.,1.),(1.,1.),(1.,1.),(1.,1.),(1.,1.),(1.,1.),(1.,
1.),(1.,1.),(1.,1.),(1.,1.),(1.,1.),(1.,1.),(1.,1.),(1.,1.),(1.,1.),(1.,
1.),(1.,1.),(1.,1.),(1.,1.),(1.,1.),(1.,1.),(1.,1.),(1.,1.),(1.,1.),(1.,
1.),(1.,1.),(1.,1.),(1.,1.),(1.,1.),(1.,1.),(1.,1.),(1.,1.),(1.,1.),(1.,
1.),(1.,1.)))
REPRESENTATION_ITEM('')
SURFACE()
);
#34=(
BOUNDED_SURFACE()
B_SPLINE_SURFACE(5,1,((#26111,#26112),(#26113,#26114),(#26115,#26116),(#26117,
#26118),(#26119,#26120),(#26121,#26122),(#26123,#26124),(#26125,#26126),
(#26127,#26128),(#26129,#26130),(#26131,#26132),(#26133,#26134),(#26135,
#26136),(#26137,#26138),(#26139,#26140),(#26141,#26142),(#26143,#26144),
(#26145,#26146),(#26147,#26148),(#26149,#26150),(#26151,#26152),(#26153,
#26154),(#26155,#26156),(#26157,#26158),(#26159,#26160),(#26161,#26162),
(#26163,#26164),(#26165,#26166),(#26167,#26168),(#26169,#26170),(#26171,
#26172),(#26173,#26174),(#26175,#26176),(#26177,#26178),(#26179,#26180),
(#26181,#26182),(#26183,#26184),(#26185,#26186),(#26187,#26188),(#26189,
#26190),(#26191,#26192),(#26193,#26194),(#26195,#26196),(#26197,#26198),
(#26199,#26200),(#26201,#26202),(#26203,#26204),(#26205,#26206),(#26207,
#26208),(#26209,#26210),(#26211,#26212),(#26213,#26214),(#26215,#26216),
(#26217,#26218),(#26219,#26220),(#26221,#26222),(#26223,#26224),(#26225,
#26226),(#26227,#26228),(#26229,#26230),(#26231,#26232),(#26233,#26234),
(#26235,#26236),(#26237,#26238),(#26239,#26240),(#26241,#26242),(#26243,
#26244),(#26245,#26246),(#26247,#26248),(#26249,#26250)),.UNSPECIFIED.,
 .F.,.F.,.F.)
B_SPLINE_SURFACE_WITH_KNOTS((6,1,1,1,1,1,1,1,1,1,1,1,1,1,1,1,1,1,1,1,1,
1,1,1,1,1,1,1,1,1,1,1,1,1,1,1,1,1,1,1,1,1,1,1,1,1,1,1,1,1,1,1,1,1,1,1,1,
1,1,1,1,1,1,1,1,6),(2,2),(-1.,-0.984615384615383,-0.969230769230768,-0.953846153846152,
-0.938461538461537,-0.923076923076922,-0.907692307692306,-0.892307692307691,
-0.876923076923076,-0.86153846153846,-0.846153846153845,-0.83076923076923,
-0.815384615384614,-0.799999999999999,-0.784615384615384,-0.769230769230768,
-0.753846153846153,-0.738461538461538,-0.723076923076922,-0.707692307692307,
-0.692307692307692,-0.676923076923076,-0.661538461538461,-0.646153846153846,
-0.63076923076923,-0.615384615384615,-0.6,-0.584615384615384,-0.569230769230769,
-0.553846153846154,-0.538461538461538,-0.523076923076923,-0.507692307692308,
-0.492307692307692,-0.476923076923077,-0.461538461538462,-0.446153846153846,
-0.430769230769231,-0.415384615384615,-0.4,-0.384615384615385,-0.369230769230769,
-0.353846153846154,-0.338461538461538,-0.323076923076923,-0.307692307692308,
-0.292307692307692,-0.276923076923077,-0.261538461538462,-0.246153846153846,
-0.230769230769231,-0.215384615384615,-0.2,-0.184615384615385,-0.169230769230769,
-0.153846153846154,-0.138461538461538,-0.123076923076923,-0.107692307692308,
-0.0923076923076923,-0.0769230769230769,-0.0615384615384615,-0.0461538461538462,
-0.0307692307692308,-0.0153846153846154,0.),(-1.,1.),.UNSPECIFIED.)
GEOMETRIC_REPRESENTATION_ITEM()
RATIONAL_B_SPLINE_SURFACE(((1.,1.),(1.,1.),(1.,1.),(1.,1.),(1.,1.),(1.,
1.),(1.,1.),(1.,1.),(1.,1.),(1.,1.),(1.,1.),(1.,1.),(1.,1.),(1.,1.),(1.,
1.),(1.,1.),(1.,1.),(1.,1.),(1.,1.),(1.,1.),(1.,1.),(1.,1.),(1.,1.),(1.,
1.),(1.,1.),(1.,1.),(1.,1.),(1.,1.),(1.,1.),(1.,1.),(1.,1.),(1.,1.),(1.,
1.),(1.,1.),(1.,1.),(1.,1.),(1.,1.),(1.,1.),(1.,1.),(1.,1.),(1.,1.),(1.,
1.),(1.,1.),(1.,1.),(1.,1.),(1.,1.),(1.,1.),(1.,1.),(1.,1.),(1.,1.),(1.,
1.),(1.,1.),(1.,1.),(1.,1.),(1.,1.),(1.,1.),(1.,1.),(1.,1.),(1.,1.),(1.,
1.),(1.,1.),(1.,1.),(1.,1.),(1.,1.),(1.,1.),(1.,1.),(1.,1.),(1.,1.),(1.,
1.),(1.,1.)))
REPRESENTATION_ITEM('')
SURFACE()
);
#35=(
BOUNDED_SURFACE()
B_SPLINE_SURFACE(5,1,((#26327,#26328),(#26329,#26330),(#26331,#26332),(#26333,
#26334),(#26335,#26336),(#26337,#26338),(#26339,#26340),(#26341,#26342),
(#26343,#26344),(#26345,#26346),(#26347,#26348),(#26349,#26350),(#26351,
#26352),(#26353,#26354),(#26355,#26356),(#26357,#26358),(#26359,#26360),
(#26361,#26362),(#26363,#26364),(#26365,#26366),(#26367,#26368),(#26369,
#26370),(#26371,#26372),(#26373,#26374),(#26375,#26376),(#26377,#26378),
(#26379,#26380),(#26381,#26382),(#26383,#26384),(#26385,#26386),(#26387,
#26388),(#26389,#26390),(#26391,#26392),(#26393,#26394),(#26395,#26396),
(#26397,#26398),(#26399,#26400),(#26401,#26402),(#26403,#26404),(#26405,
#26406),(#26407,#26408),(#26409,#26410),(#26411,#26412),(#26413,#26414),
(#26415,#26416),(#26417,#26418),(#26419,#26420),(#26421,#26422),(#26423,
#26424),(#26425,#26426),(#26427,#26428),(#26429,#26430),(#26431,#26432),
(#26433,#26434),(#26435,#26436),(#26437,#26438),(#26439,#26440),(#26441,
#26442),(#26443,#26444),(#26445,#26446),(#26447,#26448),(#26449,#26450),
(#26451,#26452),(#26453,#26454),(#26455,#26456),(#26457,#26458),(#26459,
#26460),(#26461,#26462),(#26463,#26464),(#26465,#26466)),.UNSPECIFIED.,
 .F.,.F.,.F.)
B_SPLINE_SURFACE_WITH_KNOTS((6,1,1,1,1,1,1,1,1,1,1,1,1,1,1,1,1,1,1,1,1,
1,1,1,1,1,1,1,1,1,1,1,1,1,1,1,1,1,1,1,1,1,1,1,1,1,1,1,1,1,1,1,1,1,1,1,1,
1,1,1,1,1,1,1,1,6),(2,2),(-1.,-0.984615384615383,-0.969230769230768,-0.953846153846152,
-0.938461538461537,-0.923076923076922,-0.907692307692306,-0.892307692307691,
-0.876923076923076,-0.86153846153846,-0.846153846153845,-0.83076923076923,
-0.815384615384614,-0.799999999999999,-0.784615384615384,-0.769230769230768,
-0.753846153846153,-0.738461538461538,-0.723076923076922,-0.707692307692307,
-0.692307692307692,-0.676923076923076,-0.661538461538461,-0.646153846153846,
-0.63076923076923,-0.615384615384615,-0.6,-0.584615384615384,-0.569230769230769,
-0.553846153846154,-0.538461538461538,-0.523076923076923,-0.507692307692308,
-0.492307692307692,-0.476923076923077,-0.461538461538462,-0.446153846153846,
-0.430769230769231,-0.415384615384615,-0.4,-0.384615384615385,-0.369230769230769,
-0.353846153846154,-0.338461538461538,-0.323076923076923,-0.307692307692308,
-0.292307692307692,-0.276923076923077,-0.261538461538462,-0.246153846153846,
-0.230769230769231,-0.215384615384615,-0.2,-0.184615384615385,-0.169230769230769,
-0.153846153846154,-0.138461538461538,-0.123076923076923,-0.107692307692308,
-0.0923076923076923,-0.0769230769230769,-0.0615384615384615,-0.0461538461538462,
-0.0307692307692308,-0.0153846153846154,0.),(-1.,1.),.UNSPECIFIED.)
GEOMETRIC_REPRESENTATION_ITEM()
RATIONAL_B_SPLINE_SURFACE(((1.,1.),(1.,1.),(1.,1.),(1.,1.),(1.,1.),(1.,
1.),(1.,1.),(1.,1.),(1.,1.),(1.,1.),(1.,1.),(1.,1.),(1.,1.),(1.,1.),(1.,
1.),(1.,1.),(1.,1.),(1.,1.),(1.,1.),(1.,1.),(1.,1.),(1.,1.),(1.,1.),(1.,
1.),(1.,1.),(1.,1.),(1.,1.),(1.,1.),(1.,1.),(1.,1.),(1.,1.),(1.,1.),(1.,
1.),(1.,1.),(1.,1.),(1.,1.),(1.,1.),(1.,1.),(1.,1.),(1.,1.),(1.,1.),(1.,
1.),(1.,1.),(1.,1.),(1.,1.),(1.,1.),(1.,1.),(1.,1.),(1.,1.),(1.,1.),(1.,
1.),(1.,1.),(1.,1.),(1.,1.),(1.,1.),(1.,1.),(1.,1.),(1.,1.),(1.,1.),(1.,
1.),(1.,1.),(1.,1.),(1.,1.),(1.,1.),(1.,1.),(1.,1.),(1.,1.),(1.,1.),(1.,
1.),(1.,1.)))
REPRESENTATION_ITEM('')
SURFACE()
);
#36=(
BOUNDED_SURFACE()
B_SPLINE_SURFACE(5,1,((#26543,#26544),(#26545,#26546),(#26547,#26548),(#26549,
#26550),(#26551,#26552),(#26553,#26554),(#26555,#26556),(#26557,#26558),
(#26559,#26560),(#26561,#26562),(#26563,#26564),(#26565,#26566),(#26567,
#26568),(#26569,#26570),(#26571,#26572),(#26573,#26574),(#26575,#26576),
(#26577,#26578),(#26579,#26580),(#26581,#26582),(#26583,#26584),(#26585,
#26586),(#26587,#26588),(#26589,#26590),(#26591,#26592),(#26593,#26594),
(#26595,#26596),(#26597,#26598),(#26599,#26600),(#26601,#26602),(#26603,
#26604),(#26605,#26606),(#26607,#26608),(#26609,#26610),(#26611,#26612),
(#26613,#26614),(#26615,#26616),(#26617,#26618),(#26619,#26620),(#26621,
#26622),(#26623,#26624),(#26625,#26626),(#26627,#26628),(#26629,#26630),
(#26631,#26632),(#26633,#26634),(#26635,#26636),(#26637,#26638),(#26639,
#26640),(#26641,#26642),(#26643,#26644),(#26645,#26646),(#26647,#26648),
(#26649,#26650),(#26651,#26652),(#26653,#26654),(#26655,#26656),(#26657,
#26658),(#26659,#26660),(#26661,#26662),(#26663,#26664),(#26665,#26666),
(#26667,#26668),(#26669,#26670),(#26671,#26672),(#26673,#26674),(#26675,
#26676),(#26677,#26678),(#26679,#26680),(#26681,#26682)),.UNSPECIFIED.,
 .F.,.F.,.F.)
B_SPLINE_SURFACE_WITH_KNOTS((6,1,1,1,1,1,1,1,1,1,1,1,1,1,1,1,1,1,1,1,1,
1,1,1,1,1,1,1,1,1,1,1,1,1,1,1,1,1,1,1,1,1,1,1,1,1,1,1,1,1,1,1,1,1,1,1,1,
1,1,1,1,1,1,1,1,6),(2,2),(-1.,-0.984615384615383,-0.969230769230768,-0.953846153846152,
-0.938461538461537,-0.923076923076922,-0.907692307692306,-0.892307692307691,
-0.876923076923076,-0.86153846153846,-0.846153846153845,-0.83076923076923,
-0.815384615384614,-0.799999999999999,-0.784615384615384,-0.769230769230768,
-0.753846153846153,-0.738461538461538,-0.723076923076922,-0.707692307692307,
-0.692307692307692,-0.676923076923076,-0.661538461538461,-0.646153846153846,
-0.63076923076923,-0.615384615384615,-0.6,-0.584615384615384,-0.569230769230769,
-0.553846153846154,-0.538461538461538,-0.523076923076923,-0.507692307692308,
-0.492307692307692,-0.476923076923077,-0.461538461538462,-0.446153846153846,
-0.430769230769231,-0.415384615384615,-0.4,-0.384615384615385,-0.369230769230769,
-0.353846153846154,-0.338461538461538,-0.323076923076923,-0.307692307692308,
-0.292307692307692,-0.276923076923077,-0.261538461538462,-0.246153846153846,
-0.230769230769231,-0.215384615384615,-0.2,-0.184615384615385,-0.169230769230769,
-0.153846153846154,-0.138461538461538,-0.123076923076923,-0.107692307692308,
-0.0923076923076923,-0.0769230769230769,-0.0615384615384615,-0.0461538461538462,
-0.0307692307692308,-0.0153846153846154,0.),(-1.,1.),.UNSPECIFIED.)
GEOMETRIC_REPRESENTATION_ITEM()
RATIONAL_B_SPLINE_SURFACE(((1.,1.),(1.,1.),(1.,1.),(1.,1.),(1.,1.),(1.,
1.),(1.,1.),(1.,1.),(1.,1.),(1.,1.),(1.,1.),(1.,1.),(1.,1.),(1.,1.),(1.,
1.),(1.,1.),(1.,1.),(1.,1.),(1.,1.),(1.,1.),(1.,1.),(1.,1.),(1.,1.),(1.,
1.),(1.,1.),(1.,1.),(1.,1.),(1.,1.),(1.,1.),(1.,1.),(1.,1.),(1.,1.),(1.,
1.),(1.,1.),(1.,1.),(1.,1.),(1.,1.),(1.,1.),(1.,1.),(1.,1.),(1.,1.),(1.,
1.),(1.,1.),(1.,1.),(1.,1.),(1.,1.),(1.,1.),(1.,1.),(1.,1.),(1.,1.),(1.,
1.),(1.,1.),(1.,1.),(1.,1.),(1.,1.),(1.,1.),(1.,1.),(1.,1.),(1.,1.),(1.,
1.),(1.,1.),(1.,1.),(1.,1.),(1.,1.),(1.,1.),(1.,1.),(1.,1.),(1.,1.),(1.,
1.),(1.,1.)))
REPRESENTATION_ITEM('')
SURFACE()
);
#37=(
BOUNDED_SURFACE()
B_SPLINE_SURFACE(5,1,((#26759,#26760),(#26761,#26762),(#26763,#26764),(#26765,
#26766),(#26767,#26768),(#26769,#26770),(#26771,#26772),(#26773,#26774),
(#26775,#26776),(#26777,#26778),(#26779,#26780),(#26781,#26782),(#26783,
#26784),(#26785,#26786),(#26787,#26788),(#26789,#26790),(#26791,#26792),
(#26793,#26794),(#26795,#26796),(#26797,#26798),(#26799,#26800),(#26801,
#26802),(#26803,#26804),(#26805,#26806),(#26807,#26808),(#26809,#26810),
(#26811,#26812),(#26813,#26814),(#26815,#26816),(#26817,#26818),(#26819,
#26820),(#26821,#26822),(#26823,#26824),(#26825,#26826),(#26827,#26828),
(#26829,#26830),(#26831,#26832),(#26833,#26834),(#26835,#26836),(#26837,
#26838),(#26839,#26840),(#26841,#26842),(#26843,#26844),(#26845,#26846),
(#26847,#26848),(#26849,#26850),(#26851,#26852),(#26853,#26854),(#26855,
#26856),(#26857,#26858),(#26859,#26860),(#26861,#26862),(#26863,#26864),
(#26865,#26866),(#26867,#26868),(#26869,#26870),(#26871,#26872),(#26873,
#26874),(#26875,#26876),(#26877,#26878),(#26879,#26880),(#26881,#26882),
(#26883,#26884),(#26885,#26886),(#26887,#26888),(#26889,#26890),(#26891,
#26892),(#26893,#26894),(#26895,#26896),(#26897,#26898)),.UNSPECIFIED.,
 .F.,.F.,.F.)
B_SPLINE_SURFACE_WITH_KNOTS((6,1,1,1,1,1,1,1,1,1,1,1,1,1,1,1,1,1,1,1,1,
1,1,1,1,1,1,1,1,1,1,1,1,1,1,1,1,1,1,1,1,1,1,1,1,1,1,1,1,1,1,1,1,1,1,1,1,
1,1,1,1,1,1,1,1,6),(2,2),(-1.,-0.984615384615383,-0.969230769230768,-0.953846153846152,
-0.938461538461537,-0.923076923076922,-0.907692307692306,-0.892307692307691,
-0.876923076923076,-0.86153846153846,-0.846153846153845,-0.83076923076923,
-0.815384615384614,-0.799999999999999,-0.784615384615384,-0.769230769230768,
-0.753846153846153,-0.738461538461538,-0.723076923076922,-0.707692307692307,
-0.692307692307692,-0.676923076923076,-0.661538461538461,-0.646153846153846,
-0.63076923076923,-0.615384615384615,-0.6,-0.584615384615384,-0.569230769230769,
-0.553846153846154,-0.538461538461538,-0.523076923076923,-0.507692307692308,
-0.492307692307692,-0.476923076923077,-0.461538461538462,-0.446153846153846,
-0.430769230769231,-0.415384615384615,-0.4,-0.384615384615385,-0.369230769230769,
-0.353846153846154,-0.338461538461538,-0.323076923076923,-0.307692307692308,
-0.292307692307692,-0.276923076923077,-0.261538461538462,-0.246153846153846,
-0.230769230769231,-0.215384615384615,-0.2,-0.184615384615385,-0.169230769230769,
-0.153846153846154,-0.138461538461538,-0.123076923076923,-0.107692307692308,
-0.0923076923076923,-0.0769230769230769,-0.0615384615384615,-0.0461538461538462,
-0.0307692307692308,-0.0153846153846154,0.),(-1.,1.),.UNSPECIFIED.)
GEOMETRIC_REPRESENTATION_ITEM()
RATIONAL_B_SPLINE_SURFACE(((1.,1.),(1.,1.),(1.,1.),(1.,1.),(1.,1.),(1.,
1.),(1.,1.),(1.,1.),(1.,1.),(1.,1.),(1.,1.),(1.,1.),(1.,1.),(1.,1.),(1.,
1.),(1.,1.),(1.,1.),(1.,1.),(1.,1.),(1.,1.),(1.,1.),(1.,1.),(1.,1.),(1.,
1.),(1.,1.),(1.,1.),(1.,1.),(1.,1.),(1.,1.),(1.,1.),(1.,1.),(1.,1.),(1.,
1.),(1.,1.),(1.,1.),(1.,1.),(1.,1.),(1.,1.),(1.,1.),(1.,1.),(1.,1.),(1.,
1.),(1.,1.),(1.,1.),(1.,1.),(1.,1.),(1.,1.),(1.,1.),(1.,1.),(1.,1.),(1.,
1.),(1.,1.),(1.,1.),(1.,1.),(1.,1.),(1.,1.),(1.,1.),(1.,1.),(1.,1.),(1.,
1.),(1.,1.),(1.,1.),(1.,1.),(1.,1.),(1.,1.),(1.,1.),(1.,1.),(1.,1.),(1.,
1.),(1.,1.)))
REPRESENTATION_ITEM('')
SURFACE()
);
#38=(
BOUNDED_SURFACE()
B_SPLINE_SURFACE(5,1,((#26975,#26976),(#26977,#26978),(#26979,#26980),(#26981,
#26982),(#26983,#26984),(#26985,#26986),(#26987,#26988),(#26989,#26990),
(#26991,#26992),(#26993,#26994),(#26995,#26996),(#26997,#26998),(#26999,
#27000),(#27001,#27002),(#27003,#27004),(#27005,#27006),(#27007,#27008),
(#27009,#27010),(#27011,#27012),(#27013,#27014),(#27015,#27016),(#27017,
#27018),(#27019,#27020),(#27021,#27022),(#27023,#27024),(#27025,#27026),
(#27027,#27028),(#27029,#27030),(#27031,#27032),(#27033,#27034),(#27035,
#27036),(#27037,#27038),(#27039,#27040),(#27041,#27042),(#27043,#27044),
(#27045,#27046),(#27047,#27048),(#27049,#27050),(#27051,#27052),(#27053,
#27054),(#27055,#27056),(#27057,#27058),(#27059,#27060),(#27061,#27062),
(#27063,#27064),(#27065,#27066),(#27067,#27068),(#27069,#27070),(#27071,
#27072),(#27073,#27074),(#27075,#27076),(#27077,#27078),(#27079,#27080),
(#27081,#27082),(#27083,#27084),(#27085,#27086),(#27087,#27088),(#27089,
#27090),(#27091,#27092),(#27093,#27094),(#27095,#27096),(#27097,#27098),
(#27099,#27100),(#27101,#27102),(#27103,#27104),(#27105,#27106),(#27107,
#27108),(#27109,#27110),(#27111,#27112),(#27113,#27114)),.UNSPECIFIED.,
 .F.,.F.,.F.)
B_SPLINE_SURFACE_WITH_KNOTS((6,1,1,1,1,1,1,1,1,1,1,1,1,1,1,1,1,1,1,1,1,
1,1,1,1,1,1,1,1,1,1,1,1,1,1,1,1,1,1,1,1,1,1,1,1,1,1,1,1,1,1,1,1,1,1,1,1,
1,1,1,1,1,1,1,1,6),(2,2),(-1.,-0.984615384615383,-0.969230769230768,-0.953846153846152,
-0.938461538461537,-0.923076923076922,-0.907692307692306,-0.892307692307691,
-0.876923076923076,-0.86153846153846,-0.846153846153845,-0.83076923076923,
-0.815384615384614,-0.799999999999999,-0.784615384615384,-0.769230769230768,
-0.753846153846153,-0.738461538461538,-0.723076923076922,-0.707692307692307,
-0.692307692307692,-0.676923076923076,-0.661538461538461,-0.646153846153846,
-0.63076923076923,-0.615384615384615,-0.6,-0.584615384615384,-0.569230769230769,
-0.553846153846154,-0.538461538461538,-0.523076923076923,-0.507692307692308,
-0.492307692307692,-0.476923076923077,-0.461538461538462,-0.446153846153846,
-0.430769230769231,-0.415384615384615,-0.4,-0.384615384615385,-0.369230769230769,
-0.353846153846154,-0.338461538461538,-0.323076923076923,-0.307692307692308,
-0.292307692307692,-0.276923076923077,-0.261538461538462,-0.246153846153846,
-0.230769230769231,-0.215384615384615,-0.2,-0.184615384615385,-0.169230769230769,
-0.153846153846154,-0.138461538461538,-0.123076923076923,-0.107692307692308,
-0.0923076923076923,-0.0769230769230769,-0.0615384615384615,-0.0461538461538462,
-0.0307692307692308,-0.0153846153846154,0.),(-1.,1.),.UNSPECIFIED.)
GEOMETRIC_REPRESENTATION_ITEM()
RATIONAL_B_SPLINE_SURFACE(((1.,1.),(1.,1.),(1.,1.),(1.,1.),(1.,1.),(1.,
1.),(1.,1.),(1.,1.),(1.,1.),(1.,1.),(1.,1.),(1.,1.),(1.,1.),(1.,1.),(1.,
1.),(1.,1.),(1.,1.),(1.,1.),(1.,1.),(1.,1.),(1.,1.),(1.,1.),(1.,1.),(1.,
1.),(1.,1.),(1.,1.),(1.,1.),(1.,1.),(1.,1.),(1.,1.),(1.,1.),(1.,1.),(1.,
1.),(1.,1.),(1.,1.),(1.,1.),(1.,1.),(1.,1.),(1.,1.),(1.,1.),(1.,1.),(1.,
1.),(1.,1.),(1.,1.),(1.,1.),(1.,1.),(1.,1.),(1.,1.),(1.,1.),(1.,1.),(1.,
1.),(1.,1.),(1.,1.),(1.,1.),(1.,1.),(1.,1.),(1.,1.),(1.,1.),(1.,1.),(1.,
1.),(1.,1.),(1.,1.),(1.,1.),(1.,1.),(1.,1.),(1.,1.),(1.,1.),(1.,1.),(1.,
1.),(1.,1.)))
REPRESENTATION_ITEM('')
SURFACE()
);
#39=(
BOUNDED_SURFACE()
B_SPLINE_SURFACE(5,1,((#27191,#27192),(#27193,#27194),(#27195,#27196),(#27197,
#27198),(#27199,#27200),(#27201,#27202),(#27203,#27204),(#27205,#27206),
(#27207,#27208),(#27209,#27210),(#27211,#27212),(#27213,#27214),(#27215,
#27216),(#27217,#27218),(#27219,#27220),(#27221,#27222),(#27223,#27224),
(#27225,#27226),(#27227,#27228),(#27229,#27230),(#27231,#27232),(#27233,
#27234),(#27235,#27236),(#27237,#27238),(#27239,#27240),(#27241,#27242),
(#27243,#27244),(#27245,#27246),(#27247,#27248),(#27249,#27250),(#27251,
#27252),(#27253,#27254),(#27255,#27256),(#27257,#27258),(#27259,#27260),
(#27261,#27262),(#27263,#27264),(#27265,#27266),(#27267,#27268),(#27269,
#27270),(#27271,#27272),(#27273,#27274),(#27275,#27276),(#27277,#27278),
(#27279,#27280),(#27281,#27282),(#27283,#27284),(#27285,#27286),(#27287,
#27288),(#27289,#27290),(#27291,#27292),(#27293,#27294),(#27295,#27296),
(#27297,#27298),(#27299,#27300),(#27301,#27302),(#27303,#27304),(#27305,
#27306),(#27307,#27308),(#27309,#27310),(#27311,#27312),(#27313,#27314),
(#27315,#27316),(#27317,#27318),(#27319,#27320),(#27321,#27322),(#27323,
#27324),(#27325,#27326),(#27327,#27328),(#27329,#27330)),.UNSPECIFIED.,
 .F.,.F.,.F.)
B_SPLINE_SURFACE_WITH_KNOTS((6,1,1,1,1,1,1,1,1,1,1,1,1,1,1,1,1,1,1,1,1,
1,1,1,1,1,1,1,1,1,1,1,1,1,1,1,1,1,1,1,1,1,1,1,1,1,1,1,1,1,1,1,1,1,1,1,1,
1,1,1,1,1,1,1,1,6),(2,2),(-1.,-0.984615384615383,-0.969230769230768,-0.953846153846152,
-0.938461538461537,-0.923076923076922,-0.907692307692306,-0.892307692307691,
-0.876923076923076,-0.86153846153846,-0.846153846153845,-0.83076923076923,
-0.815384615384614,-0.799999999999999,-0.784615384615384,-0.769230769230768,
-0.753846153846153,-0.738461538461538,-0.723076923076922,-0.707692307692307,
-0.692307692307692,-0.676923076923076,-0.661538461538461,-0.646153846153846,
-0.63076923076923,-0.615384615384615,-0.6,-0.584615384615384,-0.569230769230769,
-0.553846153846154,-0.538461538461538,-0.523076923076923,-0.507692307692308,
-0.492307692307692,-0.476923076923077,-0.461538461538462,-0.446153846153846,
-0.430769230769231,-0.415384615384615,-0.4,-0.384615384615385,-0.369230769230769,
-0.353846153846154,-0.338461538461538,-0.323076923076923,-0.307692307692308,
-0.292307692307692,-0.276923076923077,-0.261538461538462,-0.246153846153846,
-0.230769230769231,-0.215384615384615,-0.2,-0.184615384615385,-0.169230769230769,
-0.153846153846154,-0.138461538461538,-0.123076923076923,-0.107692307692308,
-0.0923076923076923,-0.0769230769230769,-0.0615384615384615,-0.0461538461538462,
-0.0307692307692308,-0.0153846153846154,0.),(-1.,1.),.UNSPECIFIED.)
GEOMETRIC_REPRESENTATION_ITEM()
RATIONAL_B_SPLINE_SURFACE(((1.,1.),(1.,1.),(1.,1.),(1.,1.),(1.,1.),(1.,
1.),(1.,1.),(1.,1.),(1.,1.),(1.,1.),(1.,1.),(1.,1.),(1.,1.),(1.,1.),(1.,
1.),(1.,1.),(1.,1.),(1.,1.),(1.,1.),(1.,1.),(1.,1.),(1.,1.),(1.,1.),(1.,
1.),(1.,1.),(1.,1.),(1.,1.),(1.,1.),(1.,1.),(1.,1.),(1.,1.),(1.,1.),(1.,
1.),(1.,1.),(1.,1.),(1.,1.),(1.,1.),(1.,1.),(1.,1.),(1.,1.),(1.,1.),(1.,
1.),(1.,1.),(1.,1.),(1.,1.),(1.,1.),(1.,1.),(1.,1.),(1.,1.),(1.,1.),(1.,
1.),(1.,1.),(1.,1.),(1.,1.),(1.,1.),(1.,1.),(1.,1.),(1.,1.),(1.,1.),(1.,
1.),(1.,1.),(1.,1.),(1.,1.),(1.,1.),(1.,1.),(1.,1.),(1.,1.),(1.,1.),(1.,
1.),(1.,1.)))
REPRESENTATION_ITEM('')
SURFACE()
);
#40=(
BOUNDED_SURFACE()
B_SPLINE_SURFACE(5,1,((#27407,#27408),(#27409,#27410),(#27411,#27412),(#27413,
#27414),(#27415,#27416),(#27417,#27418),(#27419,#27420),(#27421,#27422),
(#27423,#27424),(#27425,#27426),(#27427,#27428),(#27429,#27430),(#27431,
#27432),(#27433,#27434),(#27435,#27436),(#27437,#27438),(#27439,#27440),
(#27441,#27442),(#27443,#27444),(#27445,#27446),(#27447,#27448),(#27449,
#27450),(#27451,#27452),(#27453,#27454),(#27455,#27456),(#27457,#27458),
(#27459,#27460),(#27461,#27462),(#27463,#27464),(#27465,#27466),(#27467,
#27468),(#27469,#27470),(#27471,#27472),(#27473,#27474),(#27475,#27476),
(#27477,#27478),(#27479,#27480),(#27481,#27482),(#27483,#27484),(#27485,
#27486),(#27487,#27488),(#27489,#27490),(#27491,#27492),(#27493,#27494),
(#27495,#27496),(#27497,#27498),(#27499,#27500),(#27501,#27502),(#27503,
#27504),(#27505,#27506),(#27507,#27508),(#27509,#27510),(#27511,#27512),
(#27513,#27514),(#27515,#27516),(#27517,#27518),(#27519,#27520),(#27521,
#27522),(#27523,#27524),(#27525,#27526),(#27527,#27528),(#27529,#27530),
(#27531,#27532),(#27533,#27534),(#27535,#27536),(#27537,#27538),(#27539,
#27540),(#27541,#27542),(#27543,#27544),(#27545,#27546)),.UNSPECIFIED.,
 .F.,.F.,.F.)
B_SPLINE_SURFACE_WITH_KNOTS((6,1,1,1,1,1,1,1,1,1,1,1,1,1,1,1,1,1,1,1,1,
1,1,1,1,1,1,1,1,1,1,1,1,1,1,1,1,1,1,1,1,1,1,1,1,1,1,1,1,1,1,1,1,1,1,1,1,
1,1,1,1,1,1,1,1,6),(2,2),(-1.,-0.984615384615383,-0.969230769230768,-0.953846153846152,
-0.938461538461537,-0.923076923076922,-0.907692307692306,-0.892307692307691,
-0.876923076923076,-0.86153846153846,-0.846153846153845,-0.83076923076923,
-0.815384615384614,-0.799999999999999,-0.784615384615384,-0.769230769230768,
-0.753846153846153,-0.738461538461538,-0.723076923076922,-0.707692307692307,
-0.692307692307692,-0.676923076923076,-0.661538461538461,-0.646153846153846,
-0.63076923076923,-0.615384615384615,-0.6,-0.584615384615384,-0.569230769230769,
-0.553846153846154,-0.538461538461538,-0.523076923076923,-0.507692307692308,
-0.492307692307692,-0.476923076923077,-0.461538461538462,-0.446153846153846,
-0.430769230769231,-0.415384615384615,-0.4,-0.384615384615385,-0.369230769230769,
-0.353846153846154,-0.338461538461538,-0.323076923076923,-0.307692307692308,
-0.292307692307692,-0.276923076923077,-0.261538461538462,-0.246153846153846,
-0.230769230769231,-0.215384615384615,-0.2,-0.184615384615385,-0.169230769230769,
-0.153846153846154,-0.138461538461538,-0.123076923076923,-0.107692307692308,
-0.0923076923076923,-0.0769230769230769,-0.0615384615384615,-0.0461538461538462,
-0.0307692307692308,-0.0153846153846154,0.),(-1.,1.),.UNSPECIFIED.)
GEOMETRIC_REPRESENTATION_ITEM()
RATIONAL_B_SPLINE_SURFACE(((1.,1.),(1.,1.),(1.,1.),(1.,1.),(1.,1.),(1.,
1.),(1.,1.),(1.,1.),(1.,1.),(1.,1.),(1.,1.),(1.,1.),(1.,1.),(1.,1.),(1.,
1.),(1.,1.),(1.,1.),(1.,1.),(1.,1.),(1.,1.),(1.,1.),(1.,1.),(1.,1.),(1.,
1.),(1.,1.),(1.,1.),(1.,1.),(1.,1.),(1.,1.),(1.,1.),(1.,1.),(1.,1.),(1.,
1.),(1.,1.),(1.,1.),(1.,1.),(1.,1.),(1.,1.),(1.,1.),(1.,1.),(1.,1.),(1.,
1.),(1.,1.),(1.,1.),(1.,1.),(1.,1.),(1.,1.),(1.,1.),(1.,1.),(1.,1.),(1.,
1.),(1.,1.),(1.,1.),(1.,1.),(1.,1.),(1.,1.),(1.,1.),(1.,1.),(1.,1.),(1.,
1.),(1.,1.),(1.,1.),(1.,1.),(1.,1.),(1.,1.),(1.,1.),(1.,1.),(1.,1.),(1.,
1.),(1.,1.)))
REPRESENTATION_ITEM('')
SURFACE()
);
#41=(
BOUNDED_SURFACE()
B_SPLINE_SURFACE(5,1,((#27623,#27624),(#27625,#27626),(#27627,#27628),(#27629,
#27630),(#27631,#27632),(#27633,#27634),(#27635,#27636),(#27637,#27638),
(#27639,#27640),(#27641,#27642),(#27643,#27644),(#27645,#27646),(#27647,
#27648),(#27649,#27650),(#27651,#27652),(#27653,#27654),(#27655,#27656),
(#27657,#27658),(#27659,#27660),(#27661,#27662),(#27663,#27664),(#27665,
#27666),(#27667,#27668),(#27669,#27670),(#27671,#27672),(#27673,#27674),
(#27675,#27676),(#27677,#27678),(#27679,#27680),(#27681,#27682),(#27683,
#27684),(#27685,#27686),(#27687,#27688),(#27689,#27690),(#27691,#27692),
(#27693,#27694),(#27695,#27696),(#27697,#27698),(#27699,#27700),(#27701,
#27702),(#27703,#27704),(#27705,#27706),(#27707,#27708),(#27709,#27710),
(#27711,#27712),(#27713,#27714),(#27715,#27716),(#27717,#27718),(#27719,
#27720),(#27721,#27722),(#27723,#27724),(#27725,#27726),(#27727,#27728),
(#27729,#27730),(#27731,#27732),(#27733,#27734),(#27735,#27736),(#27737,
#27738),(#27739,#27740),(#27741,#27742),(#27743,#27744),(#27745,#27746),
(#27747,#27748),(#27749,#27750),(#27751,#27752),(#27753,#27754),(#27755,
#27756),(#27757,#27758),(#27759,#27760),(#27761,#27762)),.UNSPECIFIED.,
 .F.,.F.,.F.)
B_SPLINE_SURFACE_WITH_KNOTS((6,1,1,1,1,1,1,1,1,1,1,1,1,1,1,1,1,1,1,1,1,
1,1,1,1,1,1,1,1,1,1,1,1,1,1,1,1,1,1,1,1,1,1,1,1,1,1,1,1,1,1,1,1,1,1,1,1,
1,1,1,1,1,1,1,1,6),(2,2),(-1.,-0.984615384615383,-0.969230769230768,-0.953846153846152,
-0.938461538461537,-0.923076923076922,-0.907692307692306,-0.892307692307691,
-0.876923076923076,-0.86153846153846,-0.846153846153845,-0.83076923076923,
-0.815384615384614,-0.799999999999999,-0.784615384615384,-0.769230769230768,
-0.753846153846153,-0.738461538461538,-0.723076923076922,-0.707692307692307,
-0.692307692307692,-0.676923076923076,-0.661538461538461,-0.646153846153846,
-0.63076923076923,-0.615384615384615,-0.6,-0.584615384615384,-0.569230769230769,
-0.553846153846154,-0.538461538461538,-0.523076923076923,-0.507692307692308,
-0.492307692307692,-0.476923076923077,-0.461538461538462,-0.446153846153846,
-0.430769230769231,-0.415384615384615,-0.4,-0.384615384615385,-0.369230769230769,
-0.353846153846154,-0.338461538461538,-0.323076923076923,-0.307692307692308,
-0.292307692307692,-0.276923076923077,-0.261538461538462,-0.246153846153846,
-0.230769230769231,-0.215384615384615,-0.2,-0.184615384615385,-0.169230769230769,
-0.153846153846154,-0.138461538461538,-0.123076923076923,-0.107692307692308,
-0.0923076923076923,-0.0769230769230769,-0.0615384615384615,-0.0461538461538462,
-0.0307692307692308,-0.0153846153846154,0.),(-1.,1.),.UNSPECIFIED.)
GEOMETRIC_REPRESENTATION_ITEM()
RATIONAL_B_SPLINE_SURFACE(((1.,1.),(1.,1.),(1.,1.),(1.,1.),(1.,1.),(1.,
1.),(1.,1.),(1.,1.),(1.,1.),(1.,1.),(1.,1.),(1.,1.),(1.,1.),(1.,1.),(1.,
1.),(1.,1.),(1.,1.),(1.,1.),(1.,1.),(1.,1.),(1.,1.),(1.,1.),(1.,1.),(1.,
1.),(1.,1.),(1.,1.),(1.,1.),(1.,1.),(1.,1.),(1.,1.),(1.,1.),(1.,1.),(1.,
1.),(1.,1.),(1.,1.),(1.,1.),(1.,1.),(1.,1.),(1.,1.),(1.,1.),(1.,1.),(1.,
1.),(1.,1.),(1.,1.),(1.,1.),(1.,1.),(1.,1.),(1.,1.),(1.,1.),(1.,1.),(1.,
1.),(1.,1.),(1.,1.),(1.,1.),(1.,1.),(1.,1.),(1.,1.),(1.,1.),(1.,1.),(1.,
1.),(1.,1.),(1.,1.),(1.,1.),(1.,1.),(1.,1.),(1.,1.),(1.,1.),(1.,1.),(1.,
1.),(1.,1.)))
REPRESENTATION_ITEM('')
SURFACE()
);
#42=(
BOUNDED_SURFACE()
B_SPLINE_SURFACE(5,1,((#27839,#27840),(#27841,#27842),(#27843,#27844),(#27845,
#27846),(#27847,#27848),(#27849,#27850),(#27851,#27852),(#27853,#27854),
(#27855,#27856),(#27857,#27858),(#27859,#27860),(#27861,#27862),(#27863,
#27864),(#27865,#27866),(#27867,#27868),(#27869,#27870),(#27871,#27872),
(#27873,#27874),(#27875,#27876),(#27877,#27878),(#27879,#27880),(#27881,
#27882),(#27883,#27884),(#27885,#27886),(#27887,#27888),(#27889,#27890),
(#27891,#27892),(#27893,#27894),(#27895,#27896),(#27897,#27898),(#27899,
#27900),(#27901,#27902),(#27903,#27904),(#27905,#27906),(#27907,#27908),
(#27909,#27910),(#27911,#27912),(#27913,#27914),(#27915,#27916),(#27917,
#27918),(#27919,#27920),(#27921,#27922),(#27923,#27924),(#27925,#27926),
(#27927,#27928),(#27929,#27930),(#27931,#27932),(#27933,#27934),(#27935,
#27936),(#27937,#27938),(#27939,#27940),(#27941,#27942),(#27943,#27944),
(#27945,#27946),(#27947,#27948),(#27949,#27950),(#27951,#27952),(#27953,
#27954),(#27955,#27956),(#27957,#27958),(#27959,#27960),(#27961,#27962),
(#27963,#27964),(#27965,#27966),(#27967,#27968),(#27969,#27970),(#27971,
#27972),(#27973,#27974),(#27975,#27976),(#27977,#27978)),.UNSPECIFIED.,
 .F.,.F.,.F.)
B_SPLINE_SURFACE_WITH_KNOTS((6,1,1,1,1,1,1,1,1,1,1,1,1,1,1,1,1,1,1,1,1,
1,1,1,1,1,1,1,1,1,1,1,1,1,1,1,1,1,1,1,1,1,1,1,1,1,1,1,1,1,1,1,1,1,1,1,1,
1,1,1,1,1,1,1,1,6),(2,2),(-1.,-0.984615384615383,-0.969230769230768,-0.953846153846152,
-0.938461538461537,-0.923076923076922,-0.907692307692306,-0.892307692307691,
-0.876923076923076,-0.86153846153846,-0.846153846153845,-0.83076923076923,
-0.815384615384614,-0.799999999999999,-0.784615384615384,-0.769230769230768,
-0.753846153846153,-0.738461538461538,-0.723076923076922,-0.707692307692307,
-0.692307692307692,-0.676923076923076,-0.661538461538461,-0.646153846153846,
-0.63076923076923,-0.615384615384615,-0.6,-0.584615384615384,-0.569230769230769,
-0.553846153846154,-0.538461538461538,-0.523076923076923,-0.507692307692308,
-0.492307692307692,-0.476923076923077,-0.461538461538462,-0.446153846153846,
-0.430769230769231,-0.415384615384615,-0.4,-0.384615384615385,-0.369230769230769,
-0.353846153846154,-0.338461538461538,-0.323076923076923,-0.307692307692308,
-0.292307692307692,-0.276923076923077,-0.261538461538462,-0.246153846153846,
-0.230769230769231,-0.215384615384615,-0.2,-0.184615384615385,-0.169230769230769,
-0.153846153846154,-0.138461538461538,-0.123076923076923,-0.107692307692308,
-0.0923076923076923,-0.0769230769230769,-0.0615384615384615,-0.0461538461538462,
-0.0307692307692308,-0.0153846153846154,0.),(-1.,1.),.UNSPECIFIED.)
GEOMETRIC_REPRESENTATION_ITEM()
RATIONAL_B_SPLINE_SURFACE(((1.,1.),(1.,1.),(1.,1.),(1.,1.),(1.,1.),(1.,
1.),(1.,1.),(1.,1.),(1.,1.),(1.,1.),(1.,1.),(1.,1.),(1.,1.),(1.,1.),(1.,
1.),(1.,1.),(1.,1.),(1.,1.),(1.,1.),(1.,1.),(1.,1.),(1.,1.),(1.,1.),(1.,
1.),(1.,1.),(1.,1.),(1.,1.),(1.,1.),(1.,1.),(1.,1.),(1.,1.),(1.,1.),(1.,
1.),(1.,1.),(1.,1.),(1.,1.),(1.,1.),(1.,1.),(1.,1.),(1.,1.),(1.,1.),(1.,
1.),(1.,1.),(1.,1.),(1.,1.),(1.,1.),(1.,1.),(1.,1.),(1.,1.),(1.,1.),(1.,
1.),(1.,1.),(1.,1.),(1.,1.),(1.,1.),(1.,1.),(1.,1.),(1.,1.),(1.,1.),(1.,
1.),(1.,1.),(1.,1.),(1.,1.),(1.,1.),(1.,1.),(1.,1.),(1.,1.),(1.,1.),(1.,
1.),(1.,1.)))
REPRESENTATION_ITEM('')
SURFACE()
);
#43=(
BOUNDED_SURFACE()
B_SPLINE_SURFACE(5,1,((#28055,#28056),(#28057,#28058),(#28059,#28060),(#28061,
#28062),(#28063,#28064),(#28065,#28066),(#28067,#28068),(#28069,#28070),
(#28071,#28072),(#28073,#28074),(#28075,#28076),(#28077,#28078),(#28079,
#28080),(#28081,#28082),(#28083,#28084),(#28085,#28086),(#28087,#28088),
(#28089,#28090),(#28091,#28092),(#28093,#28094),(#28095,#28096),(#28097,
#28098),(#28099,#28100),(#28101,#28102),(#28103,#28104),(#28105,#28106),
(#28107,#28108),(#28109,#28110),(#28111,#28112),(#28113,#28114),(#28115,
#28116),(#28117,#28118),(#28119,#28120),(#28121,#28122),(#28123,#28124),
(#28125,#28126),(#28127,#28128),(#28129,#28130),(#28131,#28132),(#28133,
#28134),(#28135,#28136),(#28137,#28138),(#28139,#28140),(#28141,#28142),
(#28143,#28144),(#28145,#28146),(#28147,#28148),(#28149,#28150),(#28151,
#28152),(#28153,#28154),(#28155,#28156),(#28157,#28158),(#28159,#28160),
(#28161,#28162),(#28163,#28164),(#28165,#28166),(#28167,#28168),(#28169,
#28170),(#28171,#28172),(#28173,#28174),(#28175,#28176),(#28177,#28178),
(#28179,#28180),(#28181,#28182),(#28183,#28184),(#28185,#28186),(#28187,
#28188),(#28189,#28190),(#28191,#28192),(#28193,#28194)),.UNSPECIFIED.,
 .F.,.F.,.F.)
B_SPLINE_SURFACE_WITH_KNOTS((6,1,1,1,1,1,1,1,1,1,1,1,1,1,1,1,1,1,1,1,1,
1,1,1,1,1,1,1,1,1,1,1,1,1,1,1,1,1,1,1,1,1,1,1,1,1,1,1,1,1,1,1,1,1,1,1,1,
1,1,1,1,1,1,1,1,6),(2,2),(-1.,-0.984615384615383,-0.969230769230768,-0.953846153846152,
-0.938461538461537,-0.923076923076922,-0.907692307692306,-0.892307692307691,
-0.876923076923076,-0.86153846153846,-0.846153846153845,-0.83076923076923,
-0.815384615384614,-0.799999999999999,-0.784615384615384,-0.769230769230768,
-0.753846153846153,-0.738461538461538,-0.723076923076922,-0.707692307692307,
-0.692307692307692,-0.676923076923076,-0.661538461538461,-0.646153846153846,
-0.63076923076923,-0.615384615384615,-0.6,-0.584615384615384,-0.569230769230769,
-0.553846153846154,-0.538461538461538,-0.523076923076923,-0.507692307692308,
-0.492307692307692,-0.476923076923077,-0.461538461538462,-0.446153846153846,
-0.430769230769231,-0.415384615384615,-0.4,-0.384615384615385,-0.369230769230769,
-0.353846153846154,-0.338461538461538,-0.323076923076923,-0.307692307692308,
-0.292307692307692,-0.276923076923077,-0.261538461538462,-0.246153846153846,
-0.230769230769231,-0.215384615384615,-0.2,-0.184615384615385,-0.169230769230769,
-0.153846153846154,-0.138461538461538,-0.123076923076923,-0.107692307692308,
-0.0923076923076923,-0.0769230769230769,-0.0615384615384615,-0.0461538461538462,
-0.0307692307692308,-0.0153846153846154,0.),(-1.,1.),.UNSPECIFIED.)
GEOMETRIC_REPRESENTATION_ITEM()
RATIONAL_B_SPLINE_SURFACE(((1.,1.),(1.,1.),(1.,1.),(1.,1.),(1.,1.),(1.,
1.),(1.,1.),(1.,1.),(1.,1.),(1.,1.),(1.,1.),(1.,1.),(1.,1.),(1.,1.),(1.,
1.),(1.,1.),(1.,1.),(1.,1.),(1.,1.),(1.,1.),(1.,1.),(1.,1.),(1.,1.),(1.,
1.),(1.,1.),(1.,1.),(1.,1.),(1.,1.),(1.,1.),(1.,1.),(1.,1.),(1.,1.),(1.,
1.),(1.,1.),(1.,1.),(1.,1.),(1.,1.),(1.,1.),(1.,1.),(1.,1.),(1.,1.),(1.,
1.),(1.,1.),(1.,1.),(1.,1.),(1.,1.),(1.,1.),(1.,1.),(1.,1.),(1.,1.),(1.,
1.),(1.,1.),(1.,1.),(1.,1.),(1.,1.),(1.,1.),(1.,1.),(1.,1.),(1.,1.),(1.,
1.),(1.,1.),(1.,1.),(1.,1.),(1.,1.),(1.,1.),(1.,1.),(1.,1.),(1.,1.),(1.,
1.),(1.,1.)))
REPRESENTATION_ITEM('')
SURFACE()
);
#44=(
BOUNDED_SURFACE()
B_SPLINE_SURFACE(5,1,((#28271,#28272),(#28273,#28274),(#28275,#28276),(#28277,
#28278),(#28279,#28280),(#28281,#28282),(#28283,#28284),(#28285,#28286),
(#28287,#28288),(#28289,#28290),(#28291,#28292),(#28293,#28294),(#28295,
#28296),(#28297,#28298),(#28299,#28300),(#28301,#28302),(#28303,#28304),
(#28305,#28306),(#28307,#28308),(#28309,#28310),(#28311,#28312),(#28313,
#28314),(#28315,#28316),(#28317,#28318),(#28319,#28320),(#28321,#28322),
(#28323,#28324),(#28325,#28326),(#28327,#28328),(#28329,#28330),(#28331,
#28332),(#28333,#28334),(#28335,#28336),(#28337,#28338),(#28339,#28340),
(#28341,#28342),(#28343,#28344),(#28345,#28346),(#28347,#28348),(#28349,
#28350),(#28351,#28352),(#28353,#28354),(#28355,#28356),(#28357,#28358),
(#28359,#28360),(#28361,#28362),(#28363,#28364),(#28365,#28366),(#28367,
#28368),(#28369,#28370),(#28371,#28372),(#28373,#28374),(#28375,#28376),
(#28377,#28378),(#28379,#28380),(#28381,#28382),(#28383,#28384),(#28385,
#28386),(#28387,#28388),(#28389,#28390),(#28391,#28392),(#28393,#28394),
(#28395,#28396),(#28397,#28398),(#28399,#28400),(#28401,#28402),(#28403,
#28404),(#28405,#28406),(#28407,#28408),(#28409,#28410)),.UNSPECIFIED.,
 .F.,.F.,.F.)
B_SPLINE_SURFACE_WITH_KNOTS((6,1,1,1,1,1,1,1,1,1,1,1,1,1,1,1,1,1,1,1,1,
1,1,1,1,1,1,1,1,1,1,1,1,1,1,1,1,1,1,1,1,1,1,1,1,1,1,1,1,1,1,1,1,1,1,1,1,
1,1,1,1,1,1,1,1,6),(2,2),(-1.,-0.984615384615383,-0.969230769230768,-0.953846153846152,
-0.938461538461537,-0.923076923076922,-0.907692307692306,-0.892307692307691,
-0.876923076923076,-0.86153846153846,-0.846153846153845,-0.83076923076923,
-0.815384615384614,-0.799999999999999,-0.784615384615384,-0.769230769230768,
-0.753846153846153,-0.738461538461538,-0.723076923076922,-0.707692307692307,
-0.692307692307692,-0.676923076923076,-0.661538461538461,-0.646153846153846,
-0.63076923076923,-0.615384615384615,-0.6,-0.584615384615384,-0.569230769230769,
-0.553846153846154,-0.538461538461538,-0.523076923076923,-0.507692307692308,
-0.492307692307692,-0.476923076923077,-0.461538461538462,-0.446153846153846,
-0.430769230769231,-0.415384615384615,-0.4,-0.384615384615385,-0.369230769230769,
-0.353846153846154,-0.338461538461538,-0.323076923076923,-0.307692307692308,
-0.292307692307692,-0.276923076923077,-0.261538461538462,-0.246153846153846,
-0.230769230769231,-0.215384615384615,-0.2,-0.184615384615385,-0.169230769230769,
-0.153846153846154,-0.138461538461538,-0.123076923076923,-0.107692307692308,
-0.0923076923076923,-0.0769230769230769,-0.0615384615384615,-0.0461538461538462,
-0.0307692307692308,-0.0153846153846154,0.),(-1.,1.),.UNSPECIFIED.)
GEOMETRIC_REPRESENTATION_ITEM()
RATIONAL_B_SPLINE_SURFACE(((1.,1.),(1.,1.),(1.,1.),(1.,1.),(1.,1.),(1.,
1.),(1.,1.),(1.,1.),(1.,1.),(1.,1.),(1.,1.),(1.,1.),(1.,1.),(1.,1.),(1.,
1.),(1.,1.),(1.,1.),(1.,1.),(1.,1.),(1.,1.),(1.,1.),(1.,1.),(1.,1.),(1.,
1.),(1.,1.),(1.,1.),(1.,1.),(1.,1.),(1.,1.),(1.,1.),(1.,1.),(1.,1.),(1.,
1.),(1.,1.),(1.,1.),(1.,1.),(1.,1.),(1.,1.),(1.,1.),(1.,1.),(1.,1.),(1.,
1.),(1.,1.),(1.,1.),(1.,1.),(1.,1.),(1.,1.),(1.,1.),(1.,1.),(1.,1.),(1.,
1.),(1.,1.),(1.,1.),(1.,1.),(1.,1.),(1.,1.),(1.,1.),(1.,1.),(1.,1.),(1.,
1.),(1.,1.),(1.,1.),(1.,1.),(1.,1.),(1.,1.),(1.,1.),(1.,1.),(1.,1.),(1.,
1.),(1.,1.)))
REPRESENTATION_ITEM('')
SURFACE()
);
#45=(
BOUNDED_SURFACE()
B_SPLINE_SURFACE(5,1,((#28487,#28488),(#28489,#28490),(#28491,#28492),(#28493,
#28494),(#28495,#28496),(#28497,#28498),(#28499,#28500),(#28501,#28502),
(#28503,#28504),(#28505,#28506),(#28507,#28508),(#28509,#28510),(#28511,
#28512),(#28513,#28514),(#28515,#28516),(#28517,#28518),(#28519,#28520),
(#28521,#28522),(#28523,#28524),(#28525,#28526),(#28527,#28528),(#28529,
#28530),(#28531,#28532),(#28533,#28534),(#28535,#28536),(#28537,#28538),
(#28539,#28540),(#28541,#28542),(#28543,#28544),(#28545,#28546),(#28547,
#28548),(#28549,#28550),(#28551,#28552),(#28553,#28554),(#28555,#28556),
(#28557,#28558),(#28559,#28560),(#28561,#28562),(#28563,#28564),(#28565,
#28566),(#28567,#28568),(#28569,#28570),(#28571,#28572),(#28573,#28574),
(#28575,#28576),(#28577,#28578),(#28579,#28580),(#28581,#28582),(#28583,
#28584),(#28585,#28586),(#28587,#28588),(#28589,#28590),(#28591,#28592),
(#28593,#28594),(#28595,#28596),(#28597,#28598),(#28599,#28600),(#28601,
#28602),(#28603,#28604),(#28605,#28606),(#28607,#28608),(#28609,#28610),
(#28611,#28612),(#28613,#28614),(#28615,#28616),(#28617,#28618),(#28619,
#28620),(#28621,#28622),(#28623,#28624),(#28625,#28626)),.UNSPECIFIED.,
 .F.,.F.,.F.)
B_SPLINE_SURFACE_WITH_KNOTS((6,1,1,1,1,1,1,1,1,1,1,1,1,1,1,1,1,1,1,1,1,
1,1,1,1,1,1,1,1,1,1,1,1,1,1,1,1,1,1,1,1,1,1,1,1,1,1,1,1,1,1,1,1,1,1,1,1,
1,1,1,1,1,1,1,1,6),(2,2),(-1.,-0.984615384615383,-0.969230769230768,-0.953846153846152,
-0.938461538461537,-0.923076923076922,-0.907692307692306,-0.892307692307691,
-0.876923076923076,-0.86153846153846,-0.846153846153845,-0.83076923076923,
-0.815384615384614,-0.799999999999999,-0.784615384615384,-0.769230769230768,
-0.753846153846153,-0.738461538461538,-0.723076923076922,-0.707692307692307,
-0.692307692307692,-0.676923076923076,-0.661538461538461,-0.646153846153846,
-0.63076923076923,-0.615384615384615,-0.6,-0.584615384615384,-0.569230769230769,
-0.553846153846154,-0.538461538461538,-0.523076923076923,-0.507692307692308,
-0.492307692307692,-0.476923076923077,-0.461538461538462,-0.446153846153846,
-0.430769230769231,-0.415384615384615,-0.4,-0.384615384615385,-0.369230769230769,
-0.353846153846154,-0.338461538461538,-0.323076923076923,-0.307692307692308,
-0.292307692307692,-0.276923076923077,-0.261538461538462,-0.246153846153846,
-0.230769230769231,-0.215384615384615,-0.2,-0.184615384615385,-0.169230769230769,
-0.153846153846154,-0.138461538461538,-0.123076923076923,-0.107692307692308,
-0.0923076923076923,-0.0769230769230769,-0.0615384615384615,-0.0461538461538462,
-0.0307692307692308,-0.0153846153846154,0.),(-1.,1.),.UNSPECIFIED.)
GEOMETRIC_REPRESENTATION_ITEM()
RATIONAL_B_SPLINE_SURFACE(((1.,1.),(1.,1.),(1.,1.),(1.,1.),(1.,1.),(1.,
1.),(1.,1.),(1.,1.),(1.,1.),(1.,1.),(1.,1.),(1.,1.),(1.,1.),(1.,1.),(1.,
1.),(1.,1.),(1.,1.),(1.,1.),(1.,1.),(1.,1.),(1.,1.),(1.,1.),(1.,1.),(1.,
1.),(1.,1.),(1.,1.),(1.,1.),(1.,1.),(1.,1.),(1.,1.),(1.,1.),(1.,1.),(1.,
1.),(1.,1.),(1.,1.),(1.,1.),(1.,1.),(1.,1.),(1.,1.),(1.,1.),(1.,1.),(1.,
1.),(1.,1.),(1.,1.),(1.,1.),(1.,1.),(1.,1.),(1.,1.),(1.,1.),(1.,1.),(1.,
1.),(1.,1.),(1.,1.),(1.,1.),(1.,1.),(1.,1.),(1.,1.),(1.,1.),(1.,1.),(1.,
1.),(1.,1.),(1.,1.),(1.,1.),(1.,1.),(1.,1.),(1.,1.),(1.,1.),(1.,1.),(1.,
1.),(1.,1.)))
REPRESENTATION_ITEM('')
SURFACE()
);
#46=(
BOUNDED_SURFACE()
B_SPLINE_SURFACE(5,1,((#28703,#28704),(#28705,#28706),(#28707,#28708),(#28709,
#28710),(#28711,#28712),(#28713,#28714),(#28715,#28716),(#28717,#28718),
(#28719,#28720),(#28721,#28722),(#28723,#28724),(#28725,#28726),(#28727,
#28728),(#28729,#28730),(#28731,#28732),(#28733,#28734),(#28735,#28736),
(#28737,#28738),(#28739,#28740),(#28741,#28742),(#28743,#28744),(#28745,
#28746),(#28747,#28748),(#28749,#28750),(#28751,#28752),(#28753,#28754),
(#28755,#28756),(#28757,#28758),(#28759,#28760),(#28761,#28762),(#28763,
#28764),(#28765,#28766),(#28767,#28768),(#28769,#28770),(#28771,#28772),
(#28773,#28774),(#28775,#28776),(#28777,#28778),(#28779,#28780),(#28781,
#28782),(#28783,#28784),(#28785,#28786),(#28787,#28788),(#28789,#28790),
(#28791,#28792),(#28793,#28794),(#28795,#28796),(#28797,#28798),(#28799,
#28800),(#28801,#28802),(#28803,#28804),(#28805,#28806),(#28807,#28808),
(#28809,#28810),(#28811,#28812),(#28813,#28814),(#28815,#28816),(#28817,
#28818),(#28819,#28820),(#28821,#28822),(#28823,#28824),(#28825,#28826),
(#28827,#28828),(#28829,#28830),(#28831,#28832),(#28833,#28834),(#28835,
#28836),(#28837,#28838),(#28839,#28840),(#28841,#28842)),.UNSPECIFIED.,
 .F.,.F.,.F.)
B_SPLINE_SURFACE_WITH_KNOTS((6,1,1,1,1,1,1,1,1,1,1,1,1,1,1,1,1,1,1,1,1,
1,1,1,1,1,1,1,1,1,1,1,1,1,1,1,1,1,1,1,1,1,1,1,1,1,1,1,1,1,1,1,1,1,1,1,1,
1,1,1,1,1,1,1,1,6),(2,2),(-1.,-0.984615384615383,-0.969230769230768,-0.953846153846152,
-0.938461538461537,-0.923076923076922,-0.907692307692306,-0.892307692307691,
-0.876923076923076,-0.86153846153846,-0.846153846153845,-0.83076923076923,
-0.815384615384614,-0.799999999999999,-0.784615384615384,-0.769230769230768,
-0.753846153846153,-0.738461538461538,-0.723076923076922,-0.707692307692307,
-0.692307692307692,-0.676923076923076,-0.661538461538461,-0.646153846153846,
-0.63076923076923,-0.615384615384615,-0.6,-0.584615384615384,-0.569230769230769,
-0.553846153846154,-0.538461538461538,-0.523076923076923,-0.507692307692308,
-0.492307692307692,-0.476923076923077,-0.461538461538462,-0.446153846153846,
-0.430769230769231,-0.415384615384615,-0.4,-0.384615384615385,-0.369230769230769,
-0.353846153846154,-0.338461538461538,-0.323076923076923,-0.307692307692308,
-0.292307692307692,-0.276923076923077,-0.261538461538462,-0.246153846153846,
-0.230769230769231,-0.215384615384615,-0.2,-0.184615384615385,-0.169230769230769,
-0.153846153846154,-0.138461538461538,-0.123076923076923,-0.107692307692308,
-0.0923076923076923,-0.0769230769230769,-0.0615384615384615,-0.0461538461538462,
-0.0307692307692308,-0.0153846153846154,0.),(-1.,1.),.UNSPECIFIED.)
GEOMETRIC_REPRESENTATION_ITEM()
RATIONAL_B_SPLINE_SURFACE(((1.,1.),(1.,1.),(1.,1.),(1.,1.),(1.,1.),(1.,
1.),(1.,1.),(1.,1.),(1.,1.),(1.,1.),(1.,1.),(1.,1.),(1.,1.),(1.,1.),(1.,
1.),(1.,1.),(1.,1.),(1.,1.),(1.,1.),(1.,1.),(1.,1.),(1.,1.),(1.,1.),(1.,
1.),(1.,1.),(1.,1.),(1.,1.),(1.,1.),(1.,1.),(1.,1.),(1.,1.),(1.,1.),(1.,
1.),(1.,1.),(1.,1.),(1.,1.),(1.,1.),(1.,1.),(1.,1.),(1.,1.),(1.,1.),(1.,
1.),(1.,1.),(1.,1.),(1.,1.),(1.,1.),(1.,1.),(1.,1.),(1.,1.),(1.,1.),(1.,
1.),(1.,1.),(1.,1.),(1.,1.),(1.,1.),(1.,1.),(1.,1.),(1.,1.),(1.,1.),(1.,
1.),(1.,1.),(1.,1.),(1.,1.),(1.,1.),(1.,1.),(1.,1.),(1.,1.),(1.,1.),(1.,
1.),(1.,1.)))
REPRESENTATION_ITEM('')
SURFACE()
);
#47=(
BOUNDED_SURFACE()
B_SPLINE_SURFACE(5,1,((#28919,#28920),(#28921,#28922),(#28923,#28924),(#28925,
#28926),(#28927,#28928),(#28929,#28930),(#28931,#28932),(#28933,#28934),
(#28935,#28936),(#28937,#28938),(#28939,#28940),(#28941,#28942),(#28943,
#28944),(#28945,#28946),(#28947,#28948),(#28949,#28950),(#28951,#28952),
(#28953,#28954),(#28955,#28956),(#28957,#28958),(#28959,#28960),(#28961,
#28962),(#28963,#28964),(#28965,#28966),(#28967,#28968),(#28969,#28970),
(#28971,#28972),(#28973,#28974),(#28975,#28976),(#28977,#28978),(#28979,
#28980),(#28981,#28982),(#28983,#28984),(#28985,#28986),(#28987,#28988),
(#28989,#28990),(#28991,#28992),(#28993,#28994),(#28995,#28996),(#28997,
#28998),(#28999,#29000),(#29001,#29002),(#29003,#29004),(#29005,#29006),
(#29007,#29008),(#29009,#29010),(#29011,#29012),(#29013,#29014),(#29015,
#29016),(#29017,#29018),(#29019,#29020),(#29021,#29022),(#29023,#29024),
(#29025,#29026),(#29027,#29028),(#29029,#29030),(#29031,#29032),(#29033,
#29034),(#29035,#29036),(#29037,#29038),(#29039,#29040),(#29041,#29042),
(#29043,#29044),(#29045,#29046),(#29047,#29048),(#29049,#29050),(#29051,
#29052),(#29053,#29054),(#29055,#29056),(#29057,#29058)),.UNSPECIFIED.,
 .F.,.F.,.F.)
B_SPLINE_SURFACE_WITH_KNOTS((6,1,1,1,1,1,1,1,1,1,1,1,1,1,1,1,1,1,1,1,1,
1,1,1,1,1,1,1,1,1,1,1,1,1,1,1,1,1,1,1,1,1,1,1,1,1,1,1,1,1,1,1,1,1,1,1,1,
1,1,1,1,1,1,1,1,6),(2,2),(-1.,-0.984615384615383,-0.969230769230768,-0.953846153846152,
-0.938461538461537,-0.923076923076922,-0.907692307692306,-0.892307692307691,
-0.876923076923076,-0.86153846153846,-0.846153846153845,-0.83076923076923,
-0.815384615384614,-0.799999999999999,-0.784615384615384,-0.769230769230768,
-0.753846153846153,-0.738461538461538,-0.723076923076922,-0.707692307692307,
-0.692307692307692,-0.676923076923076,-0.661538461538461,-0.646153846153846,
-0.63076923076923,-0.615384615384615,-0.6,-0.584615384615384,-0.569230769230769,
-0.553846153846154,-0.538461538461538,-0.523076923076923,-0.507692307692308,
-0.492307692307692,-0.476923076923077,-0.461538461538462,-0.446153846153846,
-0.430769230769231,-0.415384615384615,-0.4,-0.384615384615385,-0.369230769230769,
-0.353846153846154,-0.338461538461538,-0.323076923076923,-0.307692307692308,
-0.292307692307692,-0.276923076923077,-0.261538461538462,-0.246153846153846,
-0.230769230769231,-0.215384615384615,-0.2,-0.184615384615385,-0.169230769230769,
-0.153846153846154,-0.138461538461538,-0.123076923076923,-0.107692307692308,
-0.0923076923076923,-0.0769230769230769,-0.0615384615384615,-0.0461538461538462,
-0.0307692307692308,-0.0153846153846154,0.),(-1.,1.),.UNSPECIFIED.)
GEOMETRIC_REPRESENTATION_ITEM()
RATIONAL_B_SPLINE_SURFACE(((1.,1.),(1.,1.),(1.,1.),(1.,1.),(1.,1.),(1.,
1.),(1.,1.),(1.,1.),(1.,1.),(1.,1.),(1.,1.),(1.,1.),(1.,1.),(1.,1.),(1.,
1.),(1.,1.),(1.,1.),(1.,1.),(1.,1.),(1.,1.),(1.,1.),(1.,1.),(1.,1.),(1.,
1.),(1.,1.),(1.,1.),(1.,1.),(1.,1.),(1.,1.),(1.,1.),(1.,1.),(1.,1.),(1.,
1.),(1.,1.),(1.,1.),(1.,1.),(1.,1.),(1.,1.),(1.,1.),(1.,1.),(1.,1.),(1.,
1.),(1.,1.),(1.,1.),(1.,1.),(1.,1.),(1.,1.),(1.,1.),(1.,1.),(1.,1.),(1.,
1.),(1.,1.),(1.,1.),(1.,1.),(1.,1.),(1.,1.),(1.,1.),(1.,1.),(1.,1.),(1.,
1.),(1.,1.),(1.,1.),(1.,1.),(1.,1.),(1.,1.),(1.,1.),(1.,1.),(1.,1.),(1.,
1.),(1.,1.)))
REPRESENTATION_ITEM('')
SURFACE()
);
#48=(
BOUNDED_SURFACE()
B_SPLINE_SURFACE(5,1,((#29135,#29136),(#29137,#29138),(#29139,#29140),(#29141,
#29142),(#29143,#29144),(#29145,#29146),(#29147,#29148),(#29149,#29150),
(#29151,#29152),(#29153,#29154),(#29155,#29156),(#29157,#29158),(#29159,
#29160),(#29161,#29162),(#29163,#29164),(#29165,#29166),(#29167,#29168),
(#29169,#29170),(#29171,#29172),(#29173,#29174),(#29175,#29176),(#29177,
#29178),(#29179,#29180),(#29181,#29182),(#29183,#29184),(#29185,#29186),
(#29187,#29188),(#29189,#29190),(#29191,#29192),(#29193,#29194),(#29195,
#29196),(#29197,#29198),(#29199,#29200),(#29201,#29202),(#29203,#29204),
(#29205,#29206),(#29207,#29208),(#29209,#29210),(#29211,#29212),(#29213,
#29214),(#29215,#29216),(#29217,#29218),(#29219,#29220),(#29221,#29222),
(#29223,#29224),(#29225,#29226),(#29227,#29228),(#29229,#29230),(#29231,
#29232),(#29233,#29234),(#29235,#29236),(#29237,#29238),(#29239,#29240),
(#29241,#29242),(#29243,#29244),(#29245,#29246),(#29247,#29248),(#29249,
#29250),(#29251,#29252),(#29253,#29254),(#29255,#29256),(#29257,#29258),
(#29259,#29260),(#29261,#29262),(#29263,#29264),(#29265,#29266),(#29267,
#29268),(#29269,#29270),(#29271,#29272),(#29273,#29274)),.UNSPECIFIED.,
 .F.,.F.,.F.)
B_SPLINE_SURFACE_WITH_KNOTS((6,1,1,1,1,1,1,1,1,1,1,1,1,1,1,1,1,1,1,1,1,
1,1,1,1,1,1,1,1,1,1,1,1,1,1,1,1,1,1,1,1,1,1,1,1,1,1,1,1,1,1,1,1,1,1,1,1,
1,1,1,1,1,1,1,1,6),(2,2),(-1.,-0.984615384615383,-0.969230769230768,-0.953846153846152,
-0.938461538461537,-0.923076923076922,-0.907692307692306,-0.892307692307691,
-0.876923076923076,-0.86153846153846,-0.846153846153845,-0.83076923076923,
-0.815384615384614,-0.799999999999999,-0.784615384615384,-0.769230769230768,
-0.753846153846153,-0.738461538461538,-0.723076923076922,-0.707692307692307,
-0.692307692307692,-0.676923076923076,-0.661538461538461,-0.646153846153846,
-0.63076923076923,-0.615384615384615,-0.6,-0.584615384615384,-0.569230769230769,
-0.553846153846154,-0.538461538461538,-0.523076923076923,-0.507692307692308,
-0.492307692307692,-0.476923076923077,-0.461538461538462,-0.446153846153846,
-0.430769230769231,-0.415384615384615,-0.4,-0.384615384615385,-0.369230769230769,
-0.353846153846154,-0.338461538461538,-0.323076923076923,-0.307692307692308,
-0.292307692307692,-0.276923076923077,-0.261538461538462,-0.246153846153846,
-0.230769230769231,-0.215384615384615,-0.2,-0.184615384615385,-0.169230769230769,
-0.153846153846154,-0.138461538461538,-0.123076923076923,-0.107692307692308,
-0.0923076923076923,-0.0769230769230769,-0.0615384615384615,-0.0461538461538462,
-0.0307692307692308,-0.0153846153846154,0.),(-1.,1.),.UNSPECIFIED.)
GEOMETRIC_REPRESENTATION_ITEM()
RATIONAL_B_SPLINE_SURFACE(((1.,1.),(1.,1.),(1.,1.),(1.,1.),(1.,1.),(1.,
1.),(1.,1.),(1.,1.),(1.,1.),(1.,1.),(1.,1.),(1.,1.),(1.,1.),(1.,1.),(1.,
1.),(1.,1.),(1.,1.),(1.,1.),(1.,1.),(1.,1.),(1.,1.),(1.,1.),(1.,1.),(1.,
1.),(1.,1.),(1.,1.),(1.,1.),(1.,1.),(1.,1.),(1.,1.),(1.,1.),(1.,1.),(1.,
1.),(1.,1.),(1.,1.),(1.,1.),(1.,1.),(1.,1.),(1.,1.),(1.,1.),(1.,1.),(1.,
1.),(1.,1.),(1.,1.),(1.,1.),(1.,1.),(1.,1.),(1.,1.),(1.,1.),(1.,1.),(1.,
1.),(1.,1.),(1.,1.),(1.,1.),(1.,1.),(1.,1.),(1.,1.),(1.,1.),(1.,1.),(1.,
1.),(1.,1.),(1.,1.),(1.,1.),(1.,1.),(1.,1.),(1.,1.),(1.,1.),(1.,1.),(1.,
1.),(1.,1.)))
REPRESENTATION_ITEM('')
SURFACE()
);
#49=(
BOUNDED_SURFACE()
B_SPLINE_SURFACE(5,1,((#29351,#29352),(#29353,#29354),(#29355,#29356),(#29357,
#29358),(#29359,#29360),(#29361,#29362),(#29363,#29364),(#29365,#29366),
(#29367,#29368),(#29369,#29370),(#29371,#29372),(#29373,#29374),(#29375,
#29376),(#29377,#29378),(#29379,#29380),(#29381,#29382),(#29383,#29384),
(#29385,#29386),(#29387,#29388),(#29389,#29390),(#29391,#29392),(#29393,
#29394),(#29395,#29396),(#29397,#29398),(#29399,#29400),(#29401,#29402),
(#29403,#29404),(#29405,#29406),(#29407,#29408),(#29409,#29410),(#29411,
#29412),(#29413,#29414),(#29415,#29416),(#29417,#29418),(#29419,#29420),
(#29421,#29422),(#29423,#29424),(#29425,#29426),(#29427,#29428),(#29429,
#29430),(#29431,#29432),(#29433,#29434),(#29435,#29436),(#29437,#29438),
(#29439,#29440),(#29441,#29442),(#29443,#29444),(#29445,#29446),(#29447,
#29448),(#29449,#29450),(#29451,#29452),(#29453,#29454),(#29455,#29456),
(#29457,#29458),(#29459,#29460),(#29461,#29462),(#29463,#29464),(#29465,
#29466),(#29467,#29468),(#29469,#29470),(#29471,#29472),(#29473,#29474),
(#29475,#29476),(#29477,#29478),(#29479,#29480),(#29481,#29482),(#29483,
#29484),(#29485,#29486),(#29487,#29488),(#29489,#29490)),.UNSPECIFIED.,
 .F.,.F.,.F.)
B_SPLINE_SURFACE_WITH_KNOTS((6,1,1,1,1,1,1,1,1,1,1,1,1,1,1,1,1,1,1,1,1,
1,1,1,1,1,1,1,1,1,1,1,1,1,1,1,1,1,1,1,1,1,1,1,1,1,1,1,1,1,1,1,1,1,1,1,1,
1,1,1,1,1,1,1,1,6),(2,2),(-1.,-0.984615384615383,-0.969230769230768,-0.953846153846152,
-0.938461538461537,-0.923076923076922,-0.907692307692306,-0.892307692307691,
-0.876923076923076,-0.86153846153846,-0.846153846153845,-0.83076923076923,
-0.815384615384614,-0.799999999999999,-0.784615384615384,-0.769230769230768,
-0.753846153846153,-0.738461538461538,-0.723076923076922,-0.707692307692307,
-0.692307692307692,-0.676923076923076,-0.661538461538461,-0.646153846153846,
-0.63076923076923,-0.615384615384615,-0.6,-0.584615384615384,-0.569230769230769,
-0.553846153846154,-0.538461538461538,-0.523076923076923,-0.507692307692308,
-0.492307692307692,-0.476923076923077,-0.461538461538462,-0.446153846153846,
-0.430769230769231,-0.415384615384615,-0.4,-0.384615384615385,-0.369230769230769,
-0.353846153846154,-0.338461538461538,-0.323076923076923,-0.307692307692308,
-0.292307692307692,-0.276923076923077,-0.261538461538462,-0.246153846153846,
-0.230769230769231,-0.215384615384615,-0.2,-0.184615384615385,-0.169230769230769,
-0.153846153846154,-0.138461538461538,-0.123076923076923,-0.107692307692308,
-0.0923076923076923,-0.0769230769230769,-0.0615384615384615,-0.0461538461538462,
-0.0307692307692308,-0.0153846153846154,0.),(-1.,1.),.UNSPECIFIED.)
GEOMETRIC_REPRESENTATION_ITEM()
RATIONAL_B_SPLINE_SURFACE(((1.,1.),(1.,1.),(1.,1.),(1.,1.),(1.,1.),(1.,
1.),(1.,1.),(1.,1.),(1.,1.),(1.,1.),(1.,1.),(1.,1.),(1.,1.),(1.,1.),(1.,
1.),(1.,1.),(1.,1.),(1.,1.),(1.,1.),(1.,1.),(1.,1.),(1.,1.),(1.,1.),(1.,
1.),(1.,1.),(1.,1.),(1.,1.),(1.,1.),(1.,1.),(1.,1.),(1.,1.),(1.,1.),(1.,
1.),(1.,1.),(1.,1.),(1.,1.),(1.,1.),(1.,1.),(1.,1.),(1.,1.),(1.,1.),(1.,
1.),(1.,1.),(1.,1.),(1.,1.),(1.,1.),(1.,1.),(1.,1.),(1.,1.),(1.,1.),(1.,
1.),(1.,1.),(1.,1.),(1.,1.),(1.,1.),(1.,1.),(1.,1.),(1.,1.),(1.,1.),(1.,
1.),(1.,1.),(1.,1.),(1.,1.),(1.,1.),(1.,1.),(1.,1.),(1.,1.),(1.,1.),(1.,
1.),(1.,1.)))
REPRESENTATION_ITEM('')
SURFACE()
);
#50=(
BOUNDED_SURFACE()
B_SPLINE_SURFACE(5,1,((#29567,#29568),(#29569,#29570),(#29571,#29572),(#29573,
#29574),(#29575,#29576),(#29577,#29578),(#29579,#29580),(#29581,#29582),
(#29583,#29584),(#29585,#29586),(#29587,#29588),(#29589,#29590),(#29591,
#29592),(#29593,#29594),(#29595,#29596),(#29597,#29598),(#29599,#29600),
(#29601,#29602),(#29603,#29604),(#29605,#29606),(#29607,#29608),(#29609,
#29610),(#29611,#29612),(#29613,#29614),(#29615,#29616),(#29617,#29618),
(#29619,#29620),(#29621,#29622),(#29623,#29624),(#29625,#29626),(#29627,
#29628),(#29629,#29630),(#29631,#29632),(#29633,#29634),(#29635,#29636),
(#29637,#29638),(#29639,#29640),(#29641,#29642),(#29643,#29644),(#29645,
#29646),(#29647,#29648),(#29649,#29650),(#29651,#29652),(#29653,#29654),
(#29655,#29656),(#29657,#29658),(#29659,#29660),(#29661,#29662),(#29663,
#29664),(#29665,#29666),(#29667,#29668),(#29669,#29670),(#29671,#29672),
(#29673,#29674),(#29675,#29676),(#29677,#29678),(#29679,#29680),(#29681,
#29682),(#29683,#29684),(#29685,#29686),(#29687,#29688),(#29689,#29690),
(#29691,#29692),(#29693,#29694),(#29695,#29696),(#29697,#29698),(#29699,
#29700),(#29701,#29702),(#29703,#29704),(#29705,#29706)),.UNSPECIFIED.,
 .F.,.F.,.F.)
B_SPLINE_SURFACE_WITH_KNOTS((6,1,1,1,1,1,1,1,1,1,1,1,1,1,1,1,1,1,1,1,1,
1,1,1,1,1,1,1,1,1,1,1,1,1,1,1,1,1,1,1,1,1,1,1,1,1,1,1,1,1,1,1,1,1,1,1,1,
1,1,1,1,1,1,1,1,6),(2,2),(-1.,-0.984615384615383,-0.969230769230768,-0.953846153846152,
-0.938461538461537,-0.923076923076922,-0.907692307692306,-0.892307692307691,
-0.876923076923076,-0.86153846153846,-0.846153846153845,-0.83076923076923,
-0.815384615384614,-0.799999999999999,-0.784615384615384,-0.769230769230768,
-0.753846153846153,-0.738461538461538,-0.723076923076922,-0.707692307692307,
-0.692307692307692,-0.676923076923076,-0.661538461538461,-0.646153846153846,
-0.63076923076923,-0.615384615384615,-0.6,-0.584615384615384,-0.569230769230769,
-0.553846153846154,-0.538461538461538,-0.523076923076923,-0.507692307692308,
-0.492307692307692,-0.476923076923077,-0.461538461538462,-0.446153846153846,
-0.430769230769231,-0.415384615384615,-0.4,-0.384615384615385,-0.369230769230769,
-0.353846153846154,-0.338461538461538,-0.323076923076923,-0.307692307692308,
-0.292307692307692,-0.276923076923077,-0.261538461538462,-0.246153846153846,
-0.230769230769231,-0.215384615384615,-0.2,-0.184615384615385,-0.169230769230769,
-0.153846153846154,-0.138461538461538,-0.123076923076923,-0.107692307692308,
-0.0923076923076923,-0.0769230769230769,-0.0615384615384615,-0.0461538461538462,
-0.0307692307692308,-0.0153846153846154,0.),(-1.,1.),.UNSPECIFIED.)
GEOMETRIC_REPRESENTATION_ITEM()
RATIONAL_B_SPLINE_SURFACE(((1.,1.),(1.,1.),(1.,1.),(1.,1.),(1.,1.),(1.,
1.),(1.,1.),(1.,1.),(1.,1.),(1.,1.),(1.,1.),(1.,1.),(1.,1.),(1.,1.),(1.,
1.),(1.,1.),(1.,1.),(1.,1.),(1.,1.),(1.,1.),(1.,1.),(1.,1.),(1.,1.),(1.,
1.),(1.,1.),(1.,1.),(1.,1.),(1.,1.),(1.,1.),(1.,1.),(1.,1.),(1.,1.),(1.,
1.),(1.,1.),(1.,1.),(1.,1.),(1.,1.),(1.,1.),(1.,1.),(1.,1.),(1.,1.),(1.,
1.),(1.,1.),(1.,1.),(1.,1.),(1.,1.),(1.,1.),(1.,1.),(1.,1.),(1.,1.),(1.,
1.),(1.,1.),(1.,1.),(1.,1.),(1.,1.),(1.,1.),(1.,1.),(1.,1.),(1.,1.),(1.,
1.),(1.,1.),(1.,1.),(1.,1.),(1.,1.),(1.,1.),(1.,1.),(1.,1.),(1.,1.),(1.,
1.),(1.,1.)))
REPRESENTATION_ITEM('')
SURFACE()
);
#131=(
BOUNDED_CURVE()
B_SPLINE_CURVE(5,(#18215,#18216,#18217,#18218,#18219,#18220,#18221,#18222,
#18223,#18224,#18225,#18226,#18227,#18228,#18229,#18230,#18231,#18232,#18233,
#18234,#18235,#18236,#18237,#18238,#18239,#18240,#18241,#18242,#18243,#18244,
#18245,#18246,#18247,#18248,#18249,#18250,#18251,#18252,#18253,#18254,#18255,
#18256,#18257,#18258,#18259,#18260,#18261,#18262,#18263,#18264,#18265,#18266,
#18267,#18268,#18269,#18270,#18271,#18272,#18273,#18274,#18275,#18276,#18277,
#18278,#18279,#18280,#18281,#18282,#18283,#18284),.UNSPECIFIED.,.F.,.F.)
B_SPLINE_CURVE_WITH_KNOTS((6,1,1,1,1,1,1,1,1,1,1,1,1,1,1,1,1,1,1,1,1,1,
1,1,1,1,1,1,1,1,1,1,1,1,1,1,1,1,1,1,1,1,1,1,1,1,1,1,1,1,1,1,1,1,1,1,1,1,
1,1,1,1,1,1,1,6),(0.,0.0153846153846154,0.0307692307692308,0.0461538461538462,
0.0615384615384615,0.0769230769230769,0.0923076923076923,0.107692307692308,
0.123076923076923,0.138461538461538,0.153846153846154,0.169230769230769,
0.184615384615385,0.2,0.215384615384615,0.230769230769231,0.246153846153846,
0.261538461538462,0.276923076923077,0.292307692307692,0.307692307692308,
0.323076923076923,0.338461538461538,0.353846153846154,0.369230769230769,
0.384615384615385,0.4,0.415384615384615,0.430769230769231,0.446153846153846,
0.461538461538462,0.476923076923077,0.492307692307692,0.507692307692308,
0.523076923076923,0.538461538461538,0.553846153846154,0.569230769230769,
0.584615384615384,0.6,0.615384615384615,0.63076923076923,0.646153846153846,
0.661538461538461,0.676923076923076,0.692307692307692,0.707692307692307,
0.723076923076922,0.738461538461538,0.753846153846153,0.769230769230768,
0.784615384615384,0.799999999999999,0.815384615384614,0.83076923076923,
0.846153846153845,0.86153846153846,0.876923076923076,0.892307692307691,
0.907692307692306,0.923076923076922,0.938461538461537,0.953846153846152,
0.969230769230768,0.984615384615383,1.),.UNSPECIFIED.)
CURVE()
GEOMETRIC_REPRESENTATION_ITEM()
RATIONAL_B_SPLINE_CURVE((1.,1.,1.,1.,1.,1.,1.,1.,1.,1.,1.,1.,1.,1.,1.,1.,
1.,1.,1.,1.,1.,1.,1.,1.,1.,1.,1.,1.,1.,1.,1.,1.,1.,1.,1.,1.,1.,1.,1.,1.,
1.,1.,1.,1.,1.,1.,1.,1.,1.,1.,1.,1.,1.,1.,1.,1.,1.,1.,1.,1.,1.,1.,1.,1.,
1.,1.,1.,1.,1.,1.))
REPRESENTATION_ITEM('')
);
#132=(
BOUNDED_CURVE()
B_SPLINE_CURVE(5,(#18288,#18289,#18290,#18291,#18292,#18293,#18294,#18295,
#18296,#18297,#18298,#18299,#18300,#18301,#18302,#18303,#18304,#18305,#18306,
#18307,#18308,#18309,#18310,#18311,#18312,#18313,#18314,#18315,#18316,#18317,
#18318,#18319,#18320,#18321,#18322,#18323,#18324,#18325,#18326,#18327,#18328,
#18329,#18330,#18331,#18332,#18333,#18334,#18335,#18336,#18337,#18338,#18339,
#18340,#18341,#18342,#18343,#18344,#18345,#18346,#18347,#18348,#18349,#18350,
#18351,#18352,#18353,#18354,#18355,#18356,#18357),.UNSPECIFIED.,.F.,.F.)
B_SPLINE_CURVE_WITH_KNOTS((6,1,1,1,1,1,1,1,1,1,1,1,1,1,1,1,1,1,1,1,1,1,
1,1,1,1,1,1,1,1,1,1,1,1,1,1,1,1,1,1,1,1,1,1,1,1,1,1,1,1,1,1,1,1,1,1,1,1,
1,1,1,1,1,1,1,6),(0.,0.0153846153846154,0.0307692307692308,0.0461538461538462,
0.0615384615384615,0.0769230769230769,0.0923076923076923,0.107692307692308,
0.123076923076923,0.138461538461538,0.153846153846154,0.169230769230769,
0.184615384615385,0.2,0.215384615384615,0.230769230769231,0.246153846153846,
0.261538461538462,0.276923076923077,0.292307692307692,0.307692307692308,
0.323076923076923,0.338461538461538,0.353846153846154,0.369230769230769,
0.384615384615385,0.4,0.415384615384615,0.430769230769231,0.446153846153846,
0.461538461538462,0.476923076923077,0.492307692307692,0.507692307692308,
0.523076923076923,0.538461538461538,0.553846153846154,0.569230769230769,
0.584615384615384,0.6,0.615384615384615,0.63076923076923,0.646153846153846,
0.661538461538461,0.676923076923076,0.692307692307692,0.707692307692307,
0.723076923076922,0.738461538461538,0.753846153846153,0.769230769230768,
0.784615384615384,0.799999999999999,0.815384615384614,0.83076923076923,
0.846153846153845,0.86153846153846,0.876923076923076,0.892307692307691,
0.907692307692306,0.923076923076922,0.938461538461537,0.953846153846152,
0.969230769230768,0.984615384615383,1.),.UNSPECIFIED.)
CURVE()
GEOMETRIC_REPRESENTATION_ITEM()
RATIONAL_B_SPLINE_CURVE((1.,1.,1.,1.,1.,1.,1.,1.,1.,1.,1.,1.,1.,1.,1.,1.,
1.,1.,1.,1.,1.,1.,1.,1.,1.,1.,1.,1.,1.,1.,1.,1.,1.,1.,1.,1.,1.,1.,1.,1.,
1.,1.,1.,1.,1.,1.,1.,1.,1.,1.,1.,1.,1.,1.,1.,1.,1.,1.,1.,1.,1.,1.,1.,1.,
1.,1.,1.,1.,1.,1.))
REPRESENTATION_ITEM('')
);
#133=(
BOUNDED_CURVE()
B_SPLINE_CURVE(5,(#18361,#18362,#18363,#18364,#18365,#18366,#18367,#18368,
#18369,#18370,#18371,#18372,#18373,#18374,#18375,#18376,#18377,#18378,#18379,
#18380,#18381,#18382,#18383,#18384,#18385,#18386,#18387,#18388,#18389,#18390,
#18391,#18392,#18393,#18394,#18395,#18396,#18397,#18398,#18399,#18400,#18401,
#18402,#18403,#18404,#18405,#18406,#18407,#18408,#18409,#18410,#18411,#18412,
#18413,#18414,#18415,#18416,#18417,#18418,#18419,#18420,#18421,#18422,#18423,
#18424,#18425,#18426,#18427,#18428,#18429,#18430),.UNSPECIFIED.,.F.,.F.)
B_SPLINE_CURVE_WITH_KNOTS((6,1,1,1,1,1,1,1,1,1,1,1,1,1,1,1,1,1,1,1,1,1,
1,1,1,1,1,1,1,1,1,1,1,1,1,1,1,1,1,1,1,1,1,1,1,1,1,1,1,1,1,1,1,1,1,1,1,1,
1,1,1,1,1,1,1,6),(0.,0.0153846153846154,0.0307692307692308,0.0461538461538462,
0.0615384615384615,0.0769230769230769,0.0923076923076923,0.107692307692308,
0.123076923076923,0.138461538461538,0.153846153846154,0.169230769230769,
0.184615384615385,0.2,0.215384615384615,0.230769230769231,0.246153846153846,
0.261538461538462,0.276923076923077,0.292307692307692,0.307692307692308,
0.323076923076923,0.338461538461538,0.353846153846154,0.369230769230769,
0.384615384615385,0.4,0.415384615384615,0.430769230769231,0.446153846153846,
0.461538461538462,0.476923076923077,0.492307692307692,0.507692307692308,
0.523076923076923,0.538461538461538,0.553846153846154,0.569230769230769,
0.584615384615384,0.6,0.615384615384615,0.63076923076923,0.646153846153846,
0.661538461538461,0.676923076923076,0.692307692307692,0.707692307692307,
0.723076923076922,0.738461538461538,0.753846153846153,0.769230769230768,
0.784615384615384,0.799999999999999,0.815384615384614,0.83076923076923,
0.846153846153845,0.86153846153846,0.876923076923076,0.892307692307691,
0.907692307692306,0.923076923076922,0.938461538461537,0.953846153846152,
0.969230769230768,0.984615384615383,1.),.UNSPECIFIED.)
CURVE()
GEOMETRIC_REPRESENTATION_ITEM()
RATIONAL_B_SPLINE_CURVE((1.,1.,1.,1.,1.,1.,1.,1.,1.,1.,1.,1.,1.,1.,1.,1.,
1.,1.,1.,1.,1.,1.,1.,1.,1.,1.,1.,1.,1.,1.,1.,1.,1.,1.,1.,1.,1.,1.,1.,1.,
1.,1.,1.,1.,1.,1.,1.,1.,1.,1.,1.,1.,1.,1.,1.,1.,1.,1.,1.,1.,1.,1.,1.,1.,
1.,1.,1.,1.,1.,1.))
REPRESENTATION_ITEM('')
);
#134=(
BOUNDED_CURVE()
B_SPLINE_CURVE(5,(#18434,#18435,#18436,#18437,#18438,#18439,#18440,#18441,
#18442,#18443,#18444,#18445,#18446,#18447,#18448,#18449,#18450,#18451,#18452,
#18453,#18454,#18455,#18456,#18457,#18458,#18459,#18460,#18461,#18462,#18463,
#18464,#18465,#18466,#18467,#18468,#18469,#18470,#18471,#18472,#18473,#18474,
#18475,#18476,#18477,#18478,#18479,#18480,#18481,#18482,#18483,#18484,#18485,
#18486,#18487,#18488,#18489,#18490,#18491,#18492,#18493,#18494,#18495,#18496,
#18497,#18498,#18499,#18500,#18501,#18502,#18503),.UNSPECIFIED.,.F.,.F.)
B_SPLINE_CURVE_WITH_KNOTS((6,1,1,1,1,1,1,1,1,1,1,1,1,1,1,1,1,1,1,1,1,1,
1,1,1,1,1,1,1,1,1,1,1,1,1,1,1,1,1,1,1,1,1,1,1,1,1,1,1,1,1,1,1,1,1,1,1,1,
1,1,1,1,1,1,1,6),(0.,0.0153846153846154,0.0307692307692308,0.0461538461538462,
0.0615384615384615,0.0769230769230769,0.0923076923076923,0.107692307692308,
0.123076923076923,0.138461538461538,0.153846153846154,0.169230769230769,
0.184615384615385,0.2,0.215384615384615,0.230769230769231,0.246153846153846,
0.261538461538462,0.276923076923077,0.292307692307692,0.307692307692308,
0.323076923076923,0.338461538461538,0.353846153846154,0.369230769230769,
0.384615384615385,0.4,0.415384615384615,0.430769230769231,0.446153846153846,
0.461538461538462,0.476923076923077,0.492307692307692,0.507692307692308,
0.523076923076923,0.538461538461538,0.553846153846154,0.569230769230769,
0.584615384615384,0.6,0.615384615384615,0.63076923076923,0.646153846153846,
0.661538461538461,0.676923076923076,0.692307692307692,0.707692307692307,
0.723076923076922,0.738461538461538,0.753846153846153,0.769230769230768,
0.784615384615384,0.799999999999999,0.815384615384614,0.83076923076923,
0.846153846153845,0.86153846153846,0.876923076923076,0.892307692307691,
0.907692307692306,0.923076923076922,0.938461538461537,0.953846153846152,
0.969230769230768,0.984615384615383,1.),.UNSPECIFIED.)
CURVE()
GEOMETRIC_REPRESENTATION_ITEM()
RATIONAL_B_SPLINE_CURVE((1.,1.,1.,1.,1.,1.,1.,1.,1.,1.,1.,1.,1.,1.,1.,1.,
1.,1.,1.,1.,1.,1.,1.,1.,1.,1.,1.,1.,1.,1.,1.,1.,1.,1.,1.,1.,1.,1.,1.,1.,
1.,1.,1.,1.,1.,1.,1.,1.,1.,1.,1.,1.,1.,1.,1.,1.,1.,1.,1.,1.,1.,1.,1.,1.,
1.,1.,1.,1.,1.,1.))
REPRESENTATION_ITEM('')
);
#135=(
BOUNDED_CURVE()
B_SPLINE_CURVE(5,(#18507,#18508,#18509,#18510,#18511,#18512,#18513,#18514,
#18515,#18516,#18517,#18518,#18519,#18520,#18521,#18522,#18523,#18524,#18525,
#18526,#18527,#18528,#18529,#18530,#18531,#18532,#18533,#18534,#18535,#18536,
#18537,#18538,#18539,#18540,#18541,#18542,#18543,#18544,#18545,#18546,#18547,
#18548,#18549,#18550,#18551,#18552,#18553,#18554,#18555,#18556,#18557,#18558,
#18559,#18560,#18561,#18562,#18563,#18564,#18565,#18566,#18567,#18568,#18569,
#18570,#18571,#18572,#18573,#18574,#18575,#18576),.UNSPECIFIED.,.F.,.F.)
B_SPLINE_CURVE_WITH_KNOTS((6,1,1,1,1,1,1,1,1,1,1,1,1,1,1,1,1,1,1,1,1,1,
1,1,1,1,1,1,1,1,1,1,1,1,1,1,1,1,1,1,1,1,1,1,1,1,1,1,1,1,1,1,1,1,1,1,1,1,
1,1,1,1,1,1,1,6),(0.,0.0153846153846154,0.0307692307692308,0.0461538461538462,
0.0615384615384615,0.0769230769230769,0.0923076923076923,0.107692307692308,
0.123076923076923,0.138461538461538,0.153846153846154,0.169230769230769,
0.184615384615385,0.2,0.215384615384615,0.230769230769231,0.246153846153846,
0.261538461538462,0.276923076923077,0.292307692307692,0.307692307692308,
0.323076923076923,0.338461538461538,0.353846153846154,0.369230769230769,
0.384615384615385,0.4,0.415384615384615,0.430769230769231,0.446153846153846,
0.461538461538462,0.476923076923077,0.492307692307692,0.507692307692308,
0.523076923076923,0.538461538461538,0.553846153846154,0.569230769230769,
0.584615384615384,0.6,0.615384615384615,0.63076923076923,0.646153846153846,
0.661538461538461,0.676923076923076,0.692307692307692,0.707692307692307,
0.723076923076922,0.738461538461538,0.753846153846153,0.769230769230768,
0.784615384615384,0.799999999999999,0.815384615384614,0.83076923076923,
0.846153846153845,0.86153846153846,0.876923076923076,0.892307692307691,
0.907692307692306,0.923076923076922,0.938461538461537,0.953846153846152,
0.969230769230768,0.984615384615383,1.),.UNSPECIFIED.)
CURVE()
GEOMETRIC_REPRESENTATION_ITEM()
RATIONAL_B_SPLINE_CURVE((1.,1.,1.,1.,1.,1.,1.,1.,1.,1.,1.,1.,1.,1.,1.,1.,
1.,1.,1.,1.,1.,1.,1.,1.,1.,1.,1.,1.,1.,1.,1.,1.,1.,1.,1.,1.,1.,1.,1.,1.,
1.,1.,1.,1.,1.,1.,1.,1.,1.,1.,1.,1.,1.,1.,1.,1.,1.,1.,1.,1.,1.,1.,1.,1.,
1.,1.,1.,1.,1.,1.))
REPRESENTATION_ITEM('')
);
#136=(
BOUNDED_CURVE()
B_SPLINE_CURVE(5,(#18580,#18581,#18582,#18583,#18584,#18585,#18586,#18587,
#18588,#18589,#18590,#18591,#18592,#18593,#18594,#18595,#18596,#18597,#18598,
#18599,#18600,#18601,#18602,#18603,#18604,#18605,#18606,#18607,#18608,#18609,
#18610,#18611,#18612,#18613,#18614,#18615,#18616,#18617,#18618,#18619,#18620,
#18621,#18622,#18623,#18624,#18625,#18626,#18627,#18628,#18629,#18630,#18631,
#18632,#18633,#18634,#18635,#18636,#18637,#18638,#18639,#18640,#18641,#18642,
#18643,#18644,#18645,#18646,#18647,#18648,#18649),.UNSPECIFIED.,.F.,.F.)
B_SPLINE_CURVE_WITH_KNOTS((6,1,1,1,1,1,1,1,1,1,1,1,1,1,1,1,1,1,1,1,1,1,
1,1,1,1,1,1,1,1,1,1,1,1,1,1,1,1,1,1,1,1,1,1,1,1,1,1,1,1,1,1,1,1,1,1,1,1,
1,1,1,1,1,1,1,6),(0.,0.0153846153846154,0.0307692307692308,0.0461538461538462,
0.0615384615384615,0.0769230769230769,0.0923076923076923,0.107692307692308,
0.123076923076923,0.138461538461538,0.153846153846154,0.169230769230769,
0.184615384615385,0.2,0.215384615384615,0.230769230769231,0.246153846153846,
0.261538461538462,0.276923076923077,0.292307692307692,0.307692307692308,
0.323076923076923,0.338461538461538,0.353846153846154,0.369230769230769,
0.384615384615385,0.4,0.415384615384615,0.430769230769231,0.446153846153846,
0.461538461538462,0.476923076923077,0.492307692307692,0.507692307692308,
0.523076923076923,0.538461538461538,0.553846153846154,0.569230769230769,
0.584615384615384,0.6,0.615384615384615,0.63076923076923,0.646153846153846,
0.661538461538461,0.676923076923076,0.692307692307692,0.707692307692307,
0.723076923076922,0.738461538461538,0.753846153846153,0.769230769230768,
0.784615384615384,0.799999999999999,0.815384615384614,0.83076923076923,
0.846153846153845,0.86153846153846,0.876923076923076,0.892307692307691,
0.907692307692306,0.923076923076922,0.938461538461537,0.953846153846152,
0.969230769230768,0.984615384615383,1.),.UNSPECIFIED.)
CURVE()
GEOMETRIC_REPRESENTATION_ITEM()
RATIONAL_B_SPLINE_CURVE((1.,1.,1.,1.,1.,1.,1.,1.,1.,1.,1.,1.,1.,1.,1.,1.,
1.,1.,1.,1.,1.,1.,1.,1.,1.,1.,1.,1.,1.,1.,1.,1.,1.,1.,1.,1.,1.,1.,1.,1.,
1.,1.,1.,1.,1.,1.,1.,1.,1.,1.,1.,1.,1.,1.,1.,1.,1.,1.,1.,1.,1.,1.,1.,1.,
1.,1.,1.,1.,1.,1.))
REPRESENTATION_ITEM('')
);
#137=(
BOUNDED_CURVE()
B_SPLINE_CURVE(5,(#18653,#18654,#18655,#18656,#18657,#18658,#18659,#18660,
#18661,#18662,#18663,#18664,#18665,#18666,#18667,#18668,#18669,#18670,#18671,
#18672,#18673,#18674,#18675,#18676,#18677,#18678,#18679,#18680,#18681,#18682,
#18683,#18684,#18685,#18686,#18687,#18688,#18689,#18690,#18691,#18692,#18693,
#18694,#18695,#18696,#18697,#18698,#18699,#18700,#18701,#18702,#18703,#18704,
#18705,#18706,#18707,#18708,#18709,#18710,#18711,#18712,#18713,#18714,#18715,
#18716,#18717,#18718,#18719,#18720,#18721,#18722),.UNSPECIFIED.,.F.,.F.)
B_SPLINE_CURVE_WITH_KNOTS((6,1,1,1,1,1,1,1,1,1,1,1,1,1,1,1,1,1,1,1,1,1,
1,1,1,1,1,1,1,1,1,1,1,1,1,1,1,1,1,1,1,1,1,1,1,1,1,1,1,1,1,1,1,1,1,1,1,1,
1,1,1,1,1,1,1,6),(0.,0.0153846153846154,0.0307692307692308,0.0461538461538462,
0.0615384615384615,0.0769230769230769,0.0923076923076923,0.107692307692308,
0.123076923076923,0.138461538461538,0.153846153846154,0.169230769230769,
0.184615384615385,0.2,0.215384615384615,0.230769230769231,0.246153846153846,
0.261538461538462,0.276923076923077,0.292307692307692,0.307692307692308,
0.323076923076923,0.338461538461538,0.353846153846154,0.369230769230769,
0.384615384615385,0.4,0.415384615384615,0.430769230769231,0.446153846153846,
0.461538461538462,0.476923076923077,0.492307692307692,0.507692307692308,
0.523076923076923,0.538461538461538,0.553846153846154,0.569230769230769,
0.584615384615384,0.6,0.615384615384615,0.63076923076923,0.646153846153846,
0.661538461538461,0.676923076923076,0.692307692307692,0.707692307692307,
0.723076923076922,0.738461538461538,0.753846153846153,0.769230769230768,
0.784615384615384,0.799999999999999,0.815384615384614,0.83076923076923,
0.846153846153845,0.86153846153846,0.876923076923076,0.892307692307691,
0.907692307692306,0.923076923076922,0.938461538461537,0.953846153846152,
0.969230769230768,0.984615384615383,1.),.UNSPECIFIED.)
CURVE()
GEOMETRIC_REPRESENTATION_ITEM()
RATIONAL_B_SPLINE_CURVE((1.,1.,1.,1.,1.,1.,1.,1.,1.,1.,1.,1.,1.,1.,1.,1.,
1.,1.,1.,1.,1.,1.,1.,1.,1.,1.,1.,1.,1.,1.,1.,1.,1.,1.,1.,1.,1.,1.,1.,1.,
1.,1.,1.,1.,1.,1.,1.,1.,1.,1.,1.,1.,1.,1.,1.,1.,1.,1.,1.,1.,1.,1.,1.,1.,
1.,1.,1.,1.,1.,1.))
REPRESENTATION_ITEM('')
);
#138=(
BOUNDED_CURVE()
B_SPLINE_CURVE(5,(#18726,#18727,#18728,#18729,#18730,#18731,#18732,#18733,
#18734,#18735,#18736,#18737,#18738,#18739,#18740,#18741,#18742,#18743,#18744,
#18745,#18746,#18747,#18748,#18749,#18750,#18751,#18752,#18753,#18754,#18755,
#18756,#18757,#18758,#18759,#18760,#18761,#18762,#18763,#18764,#18765,#18766,
#18767,#18768,#18769,#18770,#18771,#18772,#18773,#18774,#18775,#18776,#18777,
#18778,#18779,#18780,#18781,#18782,#18783,#18784,#18785,#18786,#18787,#18788,
#18789,#18790,#18791,#18792,#18793,#18794,#18795),.UNSPECIFIED.,.F.,.F.)
B_SPLINE_CURVE_WITH_KNOTS((6,1,1,1,1,1,1,1,1,1,1,1,1,1,1,1,1,1,1,1,1,1,
1,1,1,1,1,1,1,1,1,1,1,1,1,1,1,1,1,1,1,1,1,1,1,1,1,1,1,1,1,1,1,1,1,1,1,1,
1,1,1,1,1,1,1,6),(0.,0.0153846153846154,0.0307692307692308,0.0461538461538462,
0.0615384615384615,0.0769230769230769,0.0923076923076923,0.107692307692308,
0.123076923076923,0.138461538461538,0.153846153846154,0.169230769230769,
0.184615384615385,0.2,0.215384615384615,0.230769230769231,0.246153846153846,
0.261538461538462,0.276923076923077,0.292307692307692,0.307692307692308,
0.323076923076923,0.338461538461538,0.353846153846154,0.369230769230769,
0.384615384615385,0.4,0.415384615384615,0.430769230769231,0.446153846153846,
0.461538461538462,0.476923076923077,0.492307692307692,0.507692307692308,
0.523076923076923,0.538461538461538,0.553846153846154,0.569230769230769,
0.584615384615384,0.6,0.615384615384615,0.63076923076923,0.646153846153846,
0.661538461538461,0.676923076923076,0.692307692307692,0.707692307692307,
0.723076923076922,0.738461538461538,0.753846153846153,0.769230769230768,
0.784615384615384,0.799999999999999,0.815384615384614,0.83076923076923,
0.846153846153845,0.86153846153846,0.876923076923076,0.892307692307691,
0.907692307692306,0.923076923076922,0.938461538461537,0.953846153846152,
0.969230769230768,0.984615384615383,1.),.UNSPECIFIED.)
CURVE()
GEOMETRIC_REPRESENTATION_ITEM()
RATIONAL_B_SPLINE_CURVE((1.,1.,1.,1.,1.,1.,1.,1.,1.,1.,1.,1.,1.,1.,1.,1.,
1.,1.,1.,1.,1.,1.,1.,1.,1.,1.,1.,1.,1.,1.,1.,1.,1.,1.,1.,1.,1.,1.,1.,1.,
1.,1.,1.,1.,1.,1.,1.,1.,1.,1.,1.,1.,1.,1.,1.,1.,1.,1.,1.,1.,1.,1.,1.,1.,
1.,1.,1.,1.,1.,1.))
REPRESENTATION_ITEM('')
);
#139=(
BOUNDED_CURVE()
B_SPLINE_CURVE(5,(#18799,#18800,#18801,#18802,#18803,#18804,#18805,#18806,
#18807,#18808,#18809,#18810,#18811,#18812,#18813,#18814,#18815,#18816,#18817,
#18818,#18819,#18820,#18821,#18822,#18823,#18824,#18825,#18826,#18827,#18828,
#18829,#18830,#18831,#18832,#18833,#18834,#18835,#18836,#18837,#18838,#18839,
#18840,#18841,#18842,#18843,#18844,#18845,#18846,#18847,#18848,#18849,#18850,
#18851,#18852,#18853,#18854,#18855,#18856,#18857,#18858,#18859,#18860,#18861,
#18862,#18863,#18864,#18865,#18866,#18867,#18868),.UNSPECIFIED.,.F.,.F.)
B_SPLINE_CURVE_WITH_KNOTS((6,1,1,1,1,1,1,1,1,1,1,1,1,1,1,1,1,1,1,1,1,1,
1,1,1,1,1,1,1,1,1,1,1,1,1,1,1,1,1,1,1,1,1,1,1,1,1,1,1,1,1,1,1,1,1,1,1,1,
1,1,1,1,1,1,1,6),(0.,0.0153846153846154,0.0307692307692308,0.0461538461538462,
0.0615384615384615,0.0769230769230769,0.0923076923076923,0.107692307692308,
0.123076923076923,0.138461538461538,0.153846153846154,0.169230769230769,
0.184615384615385,0.2,0.215384615384615,0.230769230769231,0.246153846153846,
0.261538461538462,0.276923076923077,0.292307692307692,0.307692307692308,
0.323076923076923,0.338461538461538,0.353846153846154,0.369230769230769,
0.384615384615385,0.4,0.415384615384615,0.430769230769231,0.446153846153846,
0.461538461538462,0.476923076923077,0.492307692307692,0.507692307692308,
0.523076923076923,0.538461538461538,0.553846153846154,0.569230769230769,
0.584615384615384,0.6,0.615384615384615,0.63076923076923,0.646153846153846,
0.661538461538461,0.676923076923076,0.692307692307692,0.707692307692307,
0.723076923076922,0.738461538461538,0.753846153846153,0.769230769230768,
0.784615384615384,0.799999999999999,0.815384615384614,0.83076923076923,
0.846153846153845,0.86153846153846,0.876923076923076,0.892307692307691,
0.907692307692306,0.923076923076922,0.938461538461537,0.953846153846152,
0.969230769230768,0.984615384615383,1.),.UNSPECIFIED.)
CURVE()
GEOMETRIC_REPRESENTATION_ITEM()
RATIONAL_B_SPLINE_CURVE((1.,1.,1.,1.,1.,1.,1.,1.,1.,1.,1.,1.,1.,1.,1.,1.,
1.,1.,1.,1.,1.,1.,1.,1.,1.,1.,1.,1.,1.,1.,1.,1.,1.,1.,1.,1.,1.,1.,1.,1.,
1.,1.,1.,1.,1.,1.,1.,1.,1.,1.,1.,1.,1.,1.,1.,1.,1.,1.,1.,1.,1.,1.,1.,1.,
1.,1.,1.,1.,1.,1.))
REPRESENTATION_ITEM('')
);
#140=(
BOUNDED_CURVE()
B_SPLINE_CURVE(5,(#18872,#18873,#18874,#18875,#18876,#18877,#18878,#18879,
#18880,#18881,#18882,#18883,#18884,#18885,#18886,#18887,#18888,#18889,#18890,
#18891,#18892,#18893,#18894,#18895,#18896,#18897,#18898,#18899,#18900,#18901,
#18902,#18903,#18904,#18905,#18906,#18907,#18908,#18909,#18910,#18911,#18912,
#18913,#18914,#18915,#18916,#18917,#18918,#18919,#18920,#18921,#18922,#18923,
#18924,#18925,#18926,#18927,#18928,#18929,#18930,#18931,#18932,#18933,#18934,
#18935,#18936,#18937,#18938,#18939,#18940,#18941),.UNSPECIFIED.,.F.,.F.)
B_SPLINE_CURVE_WITH_KNOTS((6,1,1,1,1,1,1,1,1,1,1,1,1,1,1,1,1,1,1,1,1,1,
1,1,1,1,1,1,1,1,1,1,1,1,1,1,1,1,1,1,1,1,1,1,1,1,1,1,1,1,1,1,1,1,1,1,1,1,
1,1,1,1,1,1,1,6),(0.,0.0153846153846154,0.0307692307692308,0.0461538461538462,
0.0615384615384615,0.0769230769230769,0.0923076923076923,0.107692307692308,
0.123076923076923,0.138461538461538,0.153846153846154,0.169230769230769,
0.184615384615385,0.2,0.215384615384615,0.230769230769231,0.246153846153846,
0.261538461538462,0.276923076923077,0.292307692307692,0.307692307692308,
0.323076923076923,0.338461538461538,0.353846153846154,0.369230769230769,
0.384615384615385,0.4,0.415384615384615,0.430769230769231,0.446153846153846,
0.461538461538462,0.476923076923077,0.492307692307692,0.507692307692308,
0.523076923076923,0.538461538461538,0.553846153846154,0.569230769230769,
0.584615384615384,0.6,0.615384615384615,0.63076923076923,0.646153846153846,
0.661538461538461,0.676923076923076,0.692307692307692,0.707692307692307,
0.723076923076922,0.738461538461538,0.753846153846153,0.769230769230768,
0.784615384615384,0.799999999999999,0.815384615384614,0.83076923076923,
0.846153846153845,0.86153846153846,0.876923076923076,0.892307692307691,
0.907692307692306,0.923076923076922,0.938461538461537,0.953846153846152,
0.969230769230768,0.984615384615383,1.),.UNSPECIFIED.)
CURVE()
GEOMETRIC_REPRESENTATION_ITEM()
RATIONAL_B_SPLINE_CURVE((1.,1.,1.,1.,1.,1.,1.,1.,1.,1.,1.,1.,1.,1.,1.,1.,
1.,1.,1.,1.,1.,1.,1.,1.,1.,1.,1.,1.,1.,1.,1.,1.,1.,1.,1.,1.,1.,1.,1.,1.,
1.,1.,1.,1.,1.,1.,1.,1.,1.,1.,1.,1.,1.,1.,1.,1.,1.,1.,1.,1.,1.,1.,1.,1.,
1.,1.,1.,1.,1.,1.))
REPRESENTATION_ITEM('')
);
#141=(
BOUNDED_CURVE()
B_SPLINE_CURVE(5,(#18945,#18946,#18947,#18948,#18949,#18950,#18951,#18952,
#18953,#18954,#18955,#18956,#18957,#18958,#18959,#18960,#18961,#18962,#18963,
#18964,#18965,#18966,#18967,#18968,#18969,#18970,#18971,#18972,#18973,#18974,
#18975,#18976,#18977,#18978,#18979,#18980,#18981,#18982,#18983,#18984,#18985,
#18986,#18987,#18988,#18989,#18990,#18991,#18992,#18993,#18994,#18995,#18996,
#18997,#18998,#18999,#19000,#19001,#19002,#19003,#19004,#19005,#19006,#19007,
#19008,#19009,#19010,#19011,#19012,#19013,#19014),.UNSPECIFIED.,.F.,.F.)
B_SPLINE_CURVE_WITH_KNOTS((6,1,1,1,1,1,1,1,1,1,1,1,1,1,1,1,1,1,1,1,1,1,
1,1,1,1,1,1,1,1,1,1,1,1,1,1,1,1,1,1,1,1,1,1,1,1,1,1,1,1,1,1,1,1,1,1,1,1,
1,1,1,1,1,1,1,6),(0.,0.0153846153846154,0.0307692307692308,0.0461538461538462,
0.0615384615384615,0.0769230769230769,0.0923076923076923,0.107692307692308,
0.123076923076923,0.138461538461538,0.153846153846154,0.169230769230769,
0.184615384615385,0.2,0.215384615384615,0.230769230769231,0.246153846153846,
0.261538461538462,0.276923076923077,0.292307692307692,0.307692307692308,
0.323076923076923,0.338461538461538,0.353846153846154,0.369230769230769,
0.384615384615385,0.4,0.415384615384615,0.430769230769231,0.446153846153846,
0.461538461538462,0.476923076923077,0.492307692307692,0.507692307692308,
0.523076923076923,0.538461538461538,0.553846153846154,0.569230769230769,
0.584615384615384,0.6,0.615384615384615,0.63076923076923,0.646153846153846,
0.661538461538461,0.676923076923076,0.692307692307692,0.707692307692307,
0.723076923076922,0.738461538461538,0.753846153846153,0.769230769230768,
0.784615384615384,0.799999999999999,0.815384615384614,0.83076923076923,
0.846153846153845,0.86153846153846,0.876923076923076,0.892307692307691,
0.907692307692306,0.923076923076922,0.938461538461537,0.953846153846152,
0.969230769230768,0.984615384615383,1.),.UNSPECIFIED.)
CURVE()
GEOMETRIC_REPRESENTATION_ITEM()
RATIONAL_B_SPLINE_CURVE((1.,1.,1.,1.,1.,1.,1.,1.,1.,1.,1.,1.,1.,1.,1.,1.,
1.,1.,1.,1.,1.,1.,1.,1.,1.,1.,1.,1.,1.,1.,1.,1.,1.,1.,1.,1.,1.,1.,1.,1.,
1.,1.,1.,1.,1.,1.,1.,1.,1.,1.,1.,1.,1.,1.,1.,1.,1.,1.,1.,1.,1.,1.,1.,1.,
1.,1.,1.,1.,1.,1.))
REPRESENTATION_ITEM('')
);
#142=(
BOUNDED_CURVE()
B_SPLINE_CURVE(5,(#19018,#19019,#19020,#19021,#19022,#19023,#19024,#19025,
#19026,#19027,#19028,#19029,#19030,#19031,#19032,#19033,#19034,#19035,#19036,
#19037,#19038,#19039,#19040,#19041,#19042,#19043,#19044,#19045,#19046,#19047,
#19048,#19049,#19050,#19051,#19052,#19053,#19054,#19055,#19056,#19057,#19058,
#19059,#19060,#19061,#19062,#19063,#19064,#19065,#19066,#19067,#19068,#19069,
#19070,#19071,#19072,#19073,#19074,#19075,#19076,#19077,#19078,#19079,#19080,
#19081,#19082,#19083,#19084,#19085,#19086,#19087),.UNSPECIFIED.,.F.,.F.)
B_SPLINE_CURVE_WITH_KNOTS((6,1,1,1,1,1,1,1,1,1,1,1,1,1,1,1,1,1,1,1,1,1,
1,1,1,1,1,1,1,1,1,1,1,1,1,1,1,1,1,1,1,1,1,1,1,1,1,1,1,1,1,1,1,1,1,1,1,1,
1,1,1,1,1,1,1,6),(0.,0.0153846153846154,0.0307692307692308,0.0461538461538462,
0.0615384615384615,0.0769230769230769,0.0923076923076923,0.107692307692308,
0.123076923076923,0.138461538461538,0.153846153846154,0.169230769230769,
0.184615384615385,0.2,0.215384615384615,0.230769230769231,0.246153846153846,
0.261538461538462,0.276923076923077,0.292307692307692,0.307692307692308,
0.323076923076923,0.338461538461538,0.353846153846154,0.369230769230769,
0.384615384615385,0.4,0.415384615384615,0.430769230769231,0.446153846153846,
0.461538461538462,0.476923076923077,0.492307692307692,0.507692307692308,
0.523076923076923,0.538461538461538,0.553846153846154,0.569230769230769,
0.584615384615384,0.6,0.615384615384615,0.63076923076923,0.646153846153846,
0.661538461538461,0.676923076923076,0.692307692307692,0.707692307692307,
0.723076923076922,0.738461538461538,0.753846153846153,0.769230769230768,
0.784615384615384,0.799999999999999,0.815384615384614,0.83076923076923,
0.846153846153845,0.86153846153846,0.876923076923076,0.892307692307691,
0.907692307692306,0.923076923076922,0.938461538461537,0.953846153846152,
0.969230769230768,0.984615384615383,1.),.UNSPECIFIED.)
CURVE()
GEOMETRIC_REPRESENTATION_ITEM()
RATIONAL_B_SPLINE_CURVE((1.,1.,1.,1.,1.,1.,1.,1.,1.,1.,1.,1.,1.,1.,1.,1.,
1.,1.,1.,1.,1.,1.,1.,1.,1.,1.,1.,1.,1.,1.,1.,1.,1.,1.,1.,1.,1.,1.,1.,1.,
1.,1.,1.,1.,1.,1.,1.,1.,1.,1.,1.,1.,1.,1.,1.,1.,1.,1.,1.,1.,1.,1.,1.,1.,
1.,1.,1.,1.,1.,1.))
REPRESENTATION_ITEM('')
);
#143=(
BOUNDED_CURVE()
B_SPLINE_CURVE(5,(#19091,#19092,#19093,#19094,#19095,#19096,#19097,#19098,
#19099,#19100,#19101,#19102,#19103,#19104,#19105,#19106,#19107,#19108,#19109,
#19110,#19111,#19112,#19113,#19114,#19115,#19116,#19117,#19118,#19119,#19120,
#19121,#19122,#19123,#19124,#19125,#19126,#19127,#19128,#19129,#19130,#19131,
#19132,#19133,#19134,#19135,#19136,#19137,#19138,#19139,#19140,#19141,#19142,
#19143,#19144,#19145,#19146,#19147,#19148,#19149,#19150,#19151,#19152,#19153,
#19154,#19155,#19156,#19157,#19158,#19159,#19160),.UNSPECIFIED.,.F.,.F.)
B_SPLINE_CURVE_WITH_KNOTS((6,1,1,1,1,1,1,1,1,1,1,1,1,1,1,1,1,1,1,1,1,1,
1,1,1,1,1,1,1,1,1,1,1,1,1,1,1,1,1,1,1,1,1,1,1,1,1,1,1,1,1,1,1,1,1,1,1,1,
1,1,1,1,1,1,1,6),(0.,0.0153846153846154,0.0307692307692308,0.0461538461538462,
0.0615384615384615,0.0769230769230769,0.0923076923076923,0.107692307692308,
0.123076923076923,0.138461538461538,0.153846153846154,0.169230769230769,
0.184615384615385,0.2,0.215384615384615,0.230769230769231,0.246153846153846,
0.261538461538462,0.276923076923077,0.292307692307692,0.307692307692308,
0.323076923076923,0.338461538461538,0.353846153846154,0.369230769230769,
0.384615384615385,0.4,0.415384615384615,0.430769230769231,0.446153846153846,
0.461538461538462,0.476923076923077,0.492307692307692,0.507692307692308,
0.523076923076923,0.538461538461538,0.553846153846154,0.569230769230769,
0.584615384615384,0.6,0.615384615384615,0.63076923076923,0.646153846153846,
0.661538461538461,0.676923076923076,0.692307692307692,0.707692307692307,
0.723076923076922,0.738461538461538,0.753846153846153,0.769230769230768,
0.784615384615384,0.799999999999999,0.815384615384614,0.83076923076923,
0.846153846153845,0.86153846153846,0.876923076923076,0.892307692307691,
0.907692307692306,0.923076923076922,0.938461538461537,0.953846153846152,
0.969230769230768,0.984615384615383,1.),.UNSPECIFIED.)
CURVE()
GEOMETRIC_REPRESENTATION_ITEM()
RATIONAL_B_SPLINE_CURVE((1.,1.,1.,1.,1.,1.,1.,1.,1.,1.,1.,1.,1.,1.,1.,1.,
1.,1.,1.,1.,1.,1.,1.,1.,1.,1.,1.,1.,1.,1.,1.,1.,1.,1.,1.,1.,1.,1.,1.,1.,
1.,1.,1.,1.,1.,1.,1.,1.,1.,1.,1.,1.,1.,1.,1.,1.,1.,1.,1.,1.,1.,1.,1.,1.,
1.,1.,1.,1.,1.,1.))
REPRESENTATION_ITEM('')
);
#144=(
BOUNDED_CURVE()
B_SPLINE_CURVE(5,(#19164,#19165,#19166,#19167,#19168,#19169,#19170,#19171,
#19172,#19173,#19174,#19175,#19176,#19177,#19178,#19179,#19180,#19181,#19182,
#19183,#19184,#19185,#19186,#19187,#19188,#19189,#19190,#19191,#19192,#19193,
#19194,#19195,#19196,#19197,#19198,#19199,#19200,#19201,#19202,#19203,#19204,
#19205,#19206,#19207,#19208,#19209,#19210,#19211,#19212,#19213,#19214,#19215,
#19216,#19217,#19218,#19219,#19220,#19221,#19222,#19223,#19224,#19225,#19226,
#19227,#19228,#19229,#19230,#19231,#19232,#19233),.UNSPECIFIED.,.F.,.F.)
B_SPLINE_CURVE_WITH_KNOTS((6,1,1,1,1,1,1,1,1,1,1,1,1,1,1,1,1,1,1,1,1,1,
1,1,1,1,1,1,1,1,1,1,1,1,1,1,1,1,1,1,1,1,1,1,1,1,1,1,1,1,1,1,1,1,1,1,1,1,
1,1,1,1,1,1,1,6),(0.,0.0153846153846154,0.0307692307692308,0.0461538461538462,
0.0615384615384615,0.0769230769230769,0.0923076923076923,0.107692307692308,
0.123076923076923,0.138461538461538,0.153846153846154,0.169230769230769,
0.184615384615385,0.2,0.215384615384615,0.230769230769231,0.246153846153846,
0.261538461538462,0.276923076923077,0.292307692307692,0.307692307692308,
0.323076923076923,0.338461538461538,0.353846153846154,0.369230769230769,
0.384615384615385,0.4,0.415384615384615,0.430769230769231,0.446153846153846,
0.461538461538462,0.476923076923077,0.492307692307692,0.507692307692308,
0.523076923076923,0.538461538461538,0.553846153846154,0.569230769230769,
0.584615384615384,0.6,0.615384615384615,0.63076923076923,0.646153846153846,
0.661538461538461,0.676923076923076,0.692307692307692,0.707692307692307,
0.723076923076922,0.738461538461538,0.753846153846153,0.769230769230768,
0.784615384615384,0.799999999999999,0.815384615384614,0.83076923076923,
0.846153846153845,0.86153846153846,0.876923076923076,0.892307692307691,
0.907692307692306,0.923076923076922,0.938461538461537,0.953846153846152,
0.969230769230768,0.984615384615383,1.),.UNSPECIFIED.)
CURVE()
GEOMETRIC_REPRESENTATION_ITEM()
RATIONAL_B_SPLINE_CURVE((1.,1.,1.,1.,1.,1.,1.,1.,1.,1.,1.,1.,1.,1.,1.,1.,
1.,1.,1.,1.,1.,1.,1.,1.,1.,1.,1.,1.,1.,1.,1.,1.,1.,1.,1.,1.,1.,1.,1.,1.,
1.,1.,1.,1.,1.,1.,1.,1.,1.,1.,1.,1.,1.,1.,1.,1.,1.,1.,1.,1.,1.,1.,1.,1.,
1.,1.,1.,1.,1.,1.))
REPRESENTATION_ITEM('')
);
#145=(
BOUNDED_CURVE()
B_SPLINE_CURVE(5,(#19237,#19238,#19239,#19240,#19241,#19242,#19243,#19244,
#19245,#19246,#19247,#19248,#19249,#19250,#19251,#19252,#19253,#19254,#19255,
#19256,#19257,#19258,#19259,#19260,#19261,#19262,#19263,#19264,#19265,#19266,
#19267,#19268,#19269,#19270,#19271,#19272,#19273,#19274,#19275,#19276,#19277,
#19278,#19279,#19280,#19281,#19282,#19283,#19284,#19285,#19286,#19287,#19288,
#19289,#19290,#19291,#19292,#19293,#19294,#19295,#19296,#19297,#19298,#19299,
#19300,#19301,#19302,#19303,#19304,#19305,#19306),.UNSPECIFIED.,.F.,.F.)
B_SPLINE_CURVE_WITH_KNOTS((6,1,1,1,1,1,1,1,1,1,1,1,1,1,1,1,1,1,1,1,1,1,
1,1,1,1,1,1,1,1,1,1,1,1,1,1,1,1,1,1,1,1,1,1,1,1,1,1,1,1,1,1,1,1,1,1,1,1,
1,1,1,1,1,1,1,6),(0.,0.0153846153846154,0.0307692307692308,0.0461538461538462,
0.0615384615384615,0.0769230769230769,0.0923076923076923,0.107692307692308,
0.123076923076923,0.138461538461538,0.153846153846154,0.169230769230769,
0.184615384615385,0.2,0.215384615384615,0.230769230769231,0.246153846153846,
0.261538461538462,0.276923076923077,0.292307692307692,0.307692307692308,
0.323076923076923,0.338461538461538,0.353846153846154,0.369230769230769,
0.384615384615385,0.4,0.415384615384615,0.430769230769231,0.446153846153846,
0.461538461538462,0.476923076923077,0.492307692307692,0.507692307692308,
0.523076923076923,0.538461538461538,0.553846153846154,0.569230769230769,
0.584615384615384,0.6,0.615384615384615,0.63076923076923,0.646153846153846,
0.661538461538461,0.676923076923076,0.692307692307692,0.707692307692307,
0.723076923076922,0.738461538461538,0.753846153846153,0.769230769230768,
0.784615384615384,0.799999999999999,0.815384615384614,0.83076923076923,
0.846153846153845,0.86153846153846,0.876923076923076,0.892307692307691,
0.907692307692306,0.923076923076922,0.938461538461537,0.953846153846152,
0.969230769230768,0.984615384615383,1.),.UNSPECIFIED.)
CURVE()
GEOMETRIC_REPRESENTATION_ITEM()
RATIONAL_B_SPLINE_CURVE((1.,1.,1.,1.,1.,1.,1.,1.,1.,1.,1.,1.,1.,1.,1.,1.,
1.,1.,1.,1.,1.,1.,1.,1.,1.,1.,1.,1.,1.,1.,1.,1.,1.,1.,1.,1.,1.,1.,1.,1.,
1.,1.,1.,1.,1.,1.,1.,1.,1.,1.,1.,1.,1.,1.,1.,1.,1.,1.,1.,1.,1.,1.,1.,1.,
1.,1.,1.,1.,1.,1.))
REPRESENTATION_ITEM('')
);
#146=(
BOUNDED_CURVE()
B_SPLINE_CURVE(5,(#19310,#19311,#19312,#19313,#19314,#19315,#19316,#19317,
#19318,#19319,#19320,#19321,#19322,#19323,#19324,#19325,#19326,#19327,#19328,
#19329,#19330,#19331,#19332,#19333,#19334,#19335,#19336,#19337,#19338,#19339,
#19340,#19341,#19342,#19343,#19344,#19345,#19346,#19347,#19348,#19349,#19350,
#19351,#19352,#19353,#19354,#19355,#19356,#19357,#19358,#19359,#19360,#19361,
#19362,#19363,#19364,#19365,#19366,#19367,#19368,#19369,#19370,#19371,#19372,
#19373,#19374,#19375,#19376,#19377,#19378,#19379),.UNSPECIFIED.,.F.,.F.)
B_SPLINE_CURVE_WITH_KNOTS((6,1,1,1,1,1,1,1,1,1,1,1,1,1,1,1,1,1,1,1,1,1,
1,1,1,1,1,1,1,1,1,1,1,1,1,1,1,1,1,1,1,1,1,1,1,1,1,1,1,1,1,1,1,1,1,1,1,1,
1,1,1,1,1,1,1,6),(0.,0.0153846153846154,0.0307692307692308,0.0461538461538462,
0.0615384615384615,0.0769230769230769,0.0923076923076923,0.107692307692308,
0.123076923076923,0.138461538461538,0.153846153846154,0.169230769230769,
0.184615384615385,0.2,0.215384615384615,0.230769230769231,0.246153846153846,
0.261538461538462,0.276923076923077,0.292307692307692,0.307692307692308,
0.323076923076923,0.338461538461538,0.353846153846154,0.369230769230769,
0.384615384615385,0.4,0.415384615384615,0.430769230769231,0.446153846153846,
0.461538461538462,0.476923076923077,0.492307692307692,0.507692307692308,
0.523076923076923,0.538461538461538,0.553846153846154,0.569230769230769,
0.584615384615384,0.6,0.615384615384615,0.63076923076923,0.646153846153846,
0.661538461538461,0.676923076923076,0.692307692307692,0.707692307692307,
0.723076923076922,0.738461538461538,0.753846153846153,0.769230769230768,
0.784615384615384,0.799999999999999,0.815384615384614,0.83076923076923,
0.846153846153845,0.86153846153846,0.876923076923076,0.892307692307691,
0.907692307692306,0.923076923076922,0.938461538461537,0.953846153846152,
0.969230769230768,0.984615384615383,1.),.UNSPECIFIED.)
CURVE()
GEOMETRIC_REPRESENTATION_ITEM()
RATIONAL_B_SPLINE_CURVE((1.,1.,1.,1.,1.,1.,1.,1.,1.,1.,1.,1.,1.,1.,1.,1.,
1.,1.,1.,1.,1.,1.,1.,1.,1.,1.,1.,1.,1.,1.,1.,1.,1.,1.,1.,1.,1.,1.,1.,1.,
1.,1.,1.,1.,1.,1.,1.,1.,1.,1.,1.,1.,1.,1.,1.,1.,1.,1.,1.,1.,1.,1.,1.,1.,
1.,1.,1.,1.,1.,1.))
REPRESENTATION_ITEM('')
);
#147=(
BOUNDED_CURVE()
B_SPLINE_CURVE(5,(#19383,#19384,#19385,#19386,#19387,#19388,#19389,#19390,
#19391,#19392,#19393,#19394,#19395,#19396,#19397,#19398,#19399,#19400,#19401,
#19402,#19403,#19404,#19405,#19406,#19407,#19408,#19409,#19410,#19411,#19412,
#19413,#19414,#19415,#19416,#19417,#19418,#19419,#19420,#19421,#19422,#19423,
#19424,#19425,#19426,#19427,#19428,#19429,#19430,#19431,#19432,#19433,#19434,
#19435,#19436,#19437,#19438,#19439,#19440,#19441,#19442,#19443,#19444,#19445,
#19446,#19447,#19448,#19449,#19450,#19451,#19452),.UNSPECIFIED.,.F.,.F.)
B_SPLINE_CURVE_WITH_KNOTS((6,1,1,1,1,1,1,1,1,1,1,1,1,1,1,1,1,1,1,1,1,1,
1,1,1,1,1,1,1,1,1,1,1,1,1,1,1,1,1,1,1,1,1,1,1,1,1,1,1,1,1,1,1,1,1,1,1,1,
1,1,1,1,1,1,1,6),(0.,0.0153846153846154,0.0307692307692308,0.0461538461538462,
0.0615384615384615,0.0769230769230769,0.0923076923076923,0.107692307692308,
0.123076923076923,0.138461538461538,0.153846153846154,0.169230769230769,
0.184615384615385,0.2,0.215384615384615,0.230769230769231,0.246153846153846,
0.261538461538462,0.276923076923077,0.292307692307692,0.307692307692308,
0.323076923076923,0.338461538461538,0.353846153846154,0.369230769230769,
0.384615384615385,0.4,0.415384615384615,0.430769230769231,0.446153846153846,
0.461538461538462,0.476923076923077,0.492307692307692,0.507692307692308,
0.523076923076923,0.538461538461538,0.553846153846154,0.569230769230769,
0.584615384615384,0.6,0.615384615384615,0.63076923076923,0.646153846153846,
0.661538461538461,0.676923076923076,0.692307692307692,0.707692307692307,
0.723076923076922,0.738461538461538,0.753846153846153,0.769230769230768,
0.784615384615384,0.799999999999999,0.815384615384614,0.83076923076923,
0.846153846153845,0.86153846153846,0.876923076923076,0.892307692307691,
0.907692307692306,0.923076923076922,0.938461538461537,0.953846153846152,
0.969230769230768,0.984615384615383,1.),.UNSPECIFIED.)
CURVE()
GEOMETRIC_REPRESENTATION_ITEM()
RATIONAL_B_SPLINE_CURVE((1.,1.,1.,1.,1.,1.,1.,1.,1.,1.,1.,1.,1.,1.,1.,1.,
1.,1.,1.,1.,1.,1.,1.,1.,1.,1.,1.,1.,1.,1.,1.,1.,1.,1.,1.,1.,1.,1.,1.,1.,
1.,1.,1.,1.,1.,1.,1.,1.,1.,1.,1.,1.,1.,1.,1.,1.,1.,1.,1.,1.,1.,1.,1.,1.,
1.,1.,1.,1.,1.,1.))
REPRESENTATION_ITEM('')
);
#148=(
BOUNDED_CURVE()
B_SPLINE_CURVE(5,(#19456,#19457,#19458,#19459,#19460,#19461,#19462,#19463,
#19464,#19465,#19466,#19467,#19468,#19469,#19470,#19471,#19472,#19473,#19474,
#19475,#19476,#19477,#19478,#19479,#19480,#19481,#19482,#19483,#19484,#19485,
#19486,#19487,#19488,#19489,#19490,#19491,#19492,#19493,#19494,#19495,#19496,
#19497,#19498,#19499,#19500,#19501,#19502,#19503,#19504,#19505,#19506,#19507,
#19508,#19509,#19510,#19511,#19512,#19513,#19514,#19515,#19516,#19517,#19518,
#19519,#19520,#19521,#19522,#19523,#19524,#19525),.UNSPECIFIED.,.F.,.F.)
B_SPLINE_CURVE_WITH_KNOTS((6,1,1,1,1,1,1,1,1,1,1,1,1,1,1,1,1,1,1,1,1,1,
1,1,1,1,1,1,1,1,1,1,1,1,1,1,1,1,1,1,1,1,1,1,1,1,1,1,1,1,1,1,1,1,1,1,1,1,
1,1,1,1,1,1,1,6),(0.,0.0153846153846154,0.0307692307692308,0.0461538461538462,
0.0615384615384615,0.0769230769230769,0.0923076923076923,0.107692307692308,
0.123076923076923,0.138461538461538,0.153846153846154,0.169230769230769,
0.184615384615385,0.2,0.215384615384615,0.230769230769231,0.246153846153846,
0.261538461538462,0.276923076923077,0.292307692307692,0.307692307692308,
0.323076923076923,0.338461538461538,0.353846153846154,0.369230769230769,
0.384615384615385,0.4,0.415384615384615,0.430769230769231,0.446153846153846,
0.461538461538462,0.476923076923077,0.492307692307692,0.507692307692308,
0.523076923076923,0.538461538461538,0.553846153846154,0.569230769230769,
0.584615384615384,0.6,0.615384615384615,0.63076923076923,0.646153846153846,
0.661538461538461,0.676923076923076,0.692307692307692,0.707692307692307,
0.723076923076922,0.738461538461538,0.753846153846153,0.769230769230768,
0.784615384615384,0.799999999999999,0.815384615384614,0.83076923076923,
0.846153846153845,0.86153846153846,0.876923076923076,0.892307692307691,
0.907692307692306,0.923076923076922,0.938461538461537,0.953846153846152,
0.969230769230768,0.984615384615383,1.),.UNSPECIFIED.)
CURVE()
GEOMETRIC_REPRESENTATION_ITEM()
RATIONAL_B_SPLINE_CURVE((1.,1.,1.,1.,1.,1.,1.,1.,1.,1.,1.,1.,1.,1.,1.,1.,
1.,1.,1.,1.,1.,1.,1.,1.,1.,1.,1.,1.,1.,1.,1.,1.,1.,1.,1.,1.,1.,1.,1.,1.,
1.,1.,1.,1.,1.,1.,1.,1.,1.,1.,1.,1.,1.,1.,1.,1.,1.,1.,1.,1.,1.,1.,1.,1.,
1.,1.,1.,1.,1.,1.))
REPRESENTATION_ITEM('')
);
#149=(
BOUNDED_CURVE()
B_SPLINE_CURVE(5,(#19529,#19530,#19531,#19532,#19533,#19534,#19535,#19536,
#19537,#19538,#19539,#19540,#19541,#19542,#19543,#19544,#19545,#19546,#19547,
#19548,#19549,#19550,#19551,#19552,#19553,#19554,#19555,#19556,#19557,#19558,
#19559,#19560,#19561,#19562,#19563,#19564,#19565,#19566,#19567,#19568,#19569,
#19570,#19571,#19572,#19573,#19574,#19575,#19576,#19577,#19578,#19579,#19580,
#19581,#19582,#19583,#19584,#19585,#19586,#19587,#19588,#19589,#19590,#19591,
#19592,#19593,#19594,#19595,#19596,#19597,#19598),.UNSPECIFIED.,.F.,.F.)
B_SPLINE_CURVE_WITH_KNOTS((6,1,1,1,1,1,1,1,1,1,1,1,1,1,1,1,1,1,1,1,1,1,
1,1,1,1,1,1,1,1,1,1,1,1,1,1,1,1,1,1,1,1,1,1,1,1,1,1,1,1,1,1,1,1,1,1,1,1,
1,1,1,1,1,1,1,6),(0.,0.0153846153846154,0.0307692307692308,0.0461538461538462,
0.0615384615384615,0.0769230769230769,0.0923076923076923,0.107692307692308,
0.123076923076923,0.138461538461538,0.153846153846154,0.169230769230769,
0.184615384615385,0.2,0.215384615384615,0.230769230769231,0.246153846153846,
0.261538461538462,0.276923076923077,0.292307692307692,0.307692307692308,
0.323076923076923,0.338461538461538,0.353846153846154,0.369230769230769,
0.384615384615385,0.4,0.415384615384615,0.430769230769231,0.446153846153846,
0.461538461538462,0.476923076923077,0.492307692307692,0.507692307692308,
0.523076923076923,0.538461538461538,0.553846153846154,0.569230769230769,
0.584615384615384,0.6,0.615384615384615,0.63076923076923,0.646153846153846,
0.661538461538461,0.676923076923076,0.692307692307692,0.707692307692307,
0.723076923076922,0.738461538461538,0.753846153846153,0.769230769230768,
0.784615384615384,0.799999999999999,0.815384615384614,0.83076923076923,
0.846153846153845,0.86153846153846,0.876923076923076,0.892307692307691,
0.907692307692306,0.923076923076922,0.938461538461537,0.953846153846152,
0.969230769230768,0.984615384615383,1.),.UNSPECIFIED.)
CURVE()
GEOMETRIC_REPRESENTATION_ITEM()
RATIONAL_B_SPLINE_CURVE((1.,1.,1.,1.,1.,1.,1.,1.,1.,1.,1.,1.,1.,1.,1.,1.,
1.,1.,1.,1.,1.,1.,1.,1.,1.,1.,1.,1.,1.,1.,1.,1.,1.,1.,1.,1.,1.,1.,1.,1.,
1.,1.,1.,1.,1.,1.,1.,1.,1.,1.,1.,1.,1.,1.,1.,1.,1.,1.,1.,1.,1.,1.,1.,1.,
1.,1.,1.,1.,1.,1.))
REPRESENTATION_ITEM('')
);
#150=(
BOUNDED_CURVE()
B_SPLINE_CURVE(5,(#19602,#19603,#19604,#19605,#19606,#19607,#19608,#19609,
#19610,#19611,#19612,#19613,#19614,#19615,#19616,#19617,#19618,#19619,#19620,
#19621,#19622,#19623,#19624,#19625,#19626,#19627,#19628,#19629,#19630,#19631,
#19632,#19633,#19634,#19635,#19636,#19637,#19638,#19639,#19640,#19641,#19642,
#19643,#19644,#19645,#19646,#19647,#19648,#19649,#19650,#19651,#19652,#19653,
#19654,#19655,#19656,#19657,#19658,#19659,#19660,#19661,#19662,#19663,#19664,
#19665,#19666,#19667,#19668,#19669,#19670,#19671),.UNSPECIFIED.,.F.,.F.)
B_SPLINE_CURVE_WITH_KNOTS((6,1,1,1,1,1,1,1,1,1,1,1,1,1,1,1,1,1,1,1,1,1,
1,1,1,1,1,1,1,1,1,1,1,1,1,1,1,1,1,1,1,1,1,1,1,1,1,1,1,1,1,1,1,1,1,1,1,1,
1,1,1,1,1,1,1,6),(0.,0.0153846153846154,0.0307692307692308,0.0461538461538462,
0.0615384615384615,0.0769230769230769,0.0923076923076923,0.107692307692308,
0.123076923076923,0.138461538461538,0.153846153846154,0.169230769230769,
0.184615384615385,0.2,0.215384615384615,0.230769230769231,0.246153846153846,
0.261538461538462,0.276923076923077,0.292307692307692,0.307692307692308,
0.323076923076923,0.338461538461538,0.353846153846154,0.369230769230769,
0.384615384615385,0.4,0.415384615384615,0.430769230769231,0.446153846153846,
0.461538461538462,0.476923076923077,0.492307692307692,0.507692307692308,
0.523076923076923,0.538461538461538,0.553846153846154,0.569230769230769,
0.584615384615384,0.6,0.615384615384615,0.63076923076923,0.646153846153846,
0.661538461538461,0.676923076923076,0.692307692307692,0.707692307692307,
0.723076923076922,0.738461538461538,0.753846153846153,0.769230769230768,
0.784615384615384,0.799999999999999,0.815384615384614,0.83076923076923,
0.846153846153845,0.86153846153846,0.876923076923076,0.892307692307691,
0.907692307692306,0.923076923076922,0.938461538461537,0.953846153846152,
0.969230769230768,0.984615384615383,1.),.UNSPECIFIED.)
CURVE()
GEOMETRIC_REPRESENTATION_ITEM()
RATIONAL_B_SPLINE_CURVE((1.,1.,1.,1.,1.,1.,1.,1.,1.,1.,1.,1.,1.,1.,1.,1.,
1.,1.,1.,1.,1.,1.,1.,1.,1.,1.,1.,1.,1.,1.,1.,1.,1.,1.,1.,1.,1.,1.,1.,1.,
1.,1.,1.,1.,1.,1.,1.,1.,1.,1.,1.,1.,1.,1.,1.,1.,1.,1.,1.,1.,1.,1.,1.,1.,
1.,1.,1.,1.,1.,1.))
REPRESENTATION_ITEM('')
);
#151=(
BOUNDED_CURVE()
B_SPLINE_CURVE(5,(#19675,#19676,#19677,#19678,#19679,#19680,#19681,#19682,
#19683,#19684,#19685,#19686,#19687,#19688,#19689,#19690,#19691,#19692,#19693,
#19694,#19695,#19696,#19697,#19698,#19699,#19700,#19701,#19702,#19703,#19704,
#19705,#19706,#19707,#19708,#19709,#19710,#19711,#19712,#19713,#19714,#19715,
#19716,#19717,#19718,#19719,#19720,#19721,#19722,#19723,#19724,#19725,#19726,
#19727,#19728,#19729,#19730,#19731,#19732,#19733,#19734,#19735,#19736,#19737,
#19738,#19739,#19740,#19741,#19742,#19743,#19744),.UNSPECIFIED.,.F.,.F.)
B_SPLINE_CURVE_WITH_KNOTS((6,1,1,1,1,1,1,1,1,1,1,1,1,1,1,1,1,1,1,1,1,1,
1,1,1,1,1,1,1,1,1,1,1,1,1,1,1,1,1,1,1,1,1,1,1,1,1,1,1,1,1,1,1,1,1,1,1,1,
1,1,1,1,1,1,1,6),(0.,0.0153846153846154,0.0307692307692308,0.0461538461538462,
0.0615384615384615,0.0769230769230769,0.0923076923076923,0.107692307692308,
0.123076923076923,0.138461538461538,0.153846153846154,0.169230769230769,
0.184615384615385,0.2,0.215384615384615,0.230769230769231,0.246153846153846,
0.261538461538462,0.276923076923077,0.292307692307692,0.307692307692308,
0.323076923076923,0.338461538461538,0.353846153846154,0.369230769230769,
0.384615384615385,0.4,0.415384615384615,0.430769230769231,0.446153846153846,
0.461538461538462,0.476923076923077,0.492307692307692,0.507692307692308,
0.523076923076923,0.538461538461538,0.553846153846154,0.569230769230769,
0.584615384615384,0.6,0.615384615384615,0.63076923076923,0.646153846153846,
0.661538461538461,0.676923076923076,0.692307692307692,0.707692307692307,
0.723076923076922,0.738461538461538,0.753846153846153,0.769230769230768,
0.784615384615384,0.799999999999999,0.815384615384614,0.83076923076923,
0.846153846153845,0.86153846153846,0.876923076923076,0.892307692307691,
0.907692307692306,0.923076923076922,0.938461538461537,0.953846153846152,
0.969230769230768,0.984615384615383,1.),.UNSPECIFIED.)
CURVE()
GEOMETRIC_REPRESENTATION_ITEM()
RATIONAL_B_SPLINE_CURVE((1.,1.,1.,1.,1.,1.,1.,1.,1.,1.,1.,1.,1.,1.,1.,1.,
1.,1.,1.,1.,1.,1.,1.,1.,1.,1.,1.,1.,1.,1.,1.,1.,1.,1.,1.,1.,1.,1.,1.,1.,
1.,1.,1.,1.,1.,1.,1.,1.,1.,1.,1.,1.,1.,1.,1.,1.,1.,1.,1.,1.,1.,1.,1.,1.,
1.,1.,1.,1.,1.,1.))
REPRESENTATION_ITEM('')
);
#152=(
BOUNDED_CURVE()
B_SPLINE_CURVE(5,(#19748,#19749,#19750,#19751,#19752,#19753,#19754,#19755,
#19756,#19757,#19758,#19759,#19760,#19761,#19762,#19763,#19764,#19765,#19766,
#19767,#19768,#19769,#19770,#19771,#19772,#19773,#19774,#19775,#19776,#19777,
#19778,#19779,#19780,#19781,#19782,#19783,#19784,#19785,#19786,#19787,#19788,
#19789,#19790,#19791,#19792,#19793,#19794,#19795,#19796,#19797,#19798,#19799,
#19800,#19801,#19802,#19803,#19804,#19805,#19806,#19807,#19808,#19809,#19810,
#19811,#19812,#19813,#19814,#19815,#19816,#19817),.UNSPECIFIED.,.F.,.F.)
B_SPLINE_CURVE_WITH_KNOTS((6,1,1,1,1,1,1,1,1,1,1,1,1,1,1,1,1,1,1,1,1,1,
1,1,1,1,1,1,1,1,1,1,1,1,1,1,1,1,1,1,1,1,1,1,1,1,1,1,1,1,1,1,1,1,1,1,1,1,
1,1,1,1,1,1,1,6),(0.,0.0153846153846154,0.0307692307692308,0.0461538461538462,
0.0615384615384615,0.0769230769230769,0.0923076923076923,0.107692307692308,
0.123076923076923,0.138461538461538,0.153846153846154,0.169230769230769,
0.184615384615385,0.2,0.215384615384615,0.230769230769231,0.246153846153846,
0.261538461538462,0.276923076923077,0.292307692307692,0.307692307692308,
0.323076923076923,0.338461538461538,0.353846153846154,0.369230769230769,
0.384615384615385,0.4,0.415384615384615,0.430769230769231,0.446153846153846,
0.461538461538462,0.476923076923077,0.492307692307692,0.507692307692308,
0.523076923076923,0.538461538461538,0.553846153846154,0.569230769230769,
0.584615384615384,0.6,0.615384615384615,0.63076923076923,0.646153846153846,
0.661538461538461,0.676923076923076,0.692307692307692,0.707692307692307,
0.723076923076922,0.738461538461538,0.753846153846153,0.769230769230768,
0.784615384615384,0.799999999999999,0.815384615384614,0.83076923076923,
0.846153846153845,0.86153846153846,0.876923076923076,0.892307692307691,
0.907692307692306,0.923076923076922,0.938461538461537,0.953846153846152,
0.969230769230768,0.984615384615383,1.),.UNSPECIFIED.)
CURVE()
GEOMETRIC_REPRESENTATION_ITEM()
RATIONAL_B_SPLINE_CURVE((1.,1.,1.,1.,1.,1.,1.,1.,1.,1.,1.,1.,1.,1.,1.,1.,
1.,1.,1.,1.,1.,1.,1.,1.,1.,1.,1.,1.,1.,1.,1.,1.,1.,1.,1.,1.,1.,1.,1.,1.,
1.,1.,1.,1.,1.,1.,1.,1.,1.,1.,1.,1.,1.,1.,1.,1.,1.,1.,1.,1.,1.,1.,1.,1.,
1.,1.,1.,1.,1.,1.))
REPRESENTATION_ITEM('')
);
#153=(
BOUNDED_CURVE()
B_SPLINE_CURVE(5,(#19821,#19822,#19823,#19824,#19825,#19826,#19827,#19828,
#19829,#19830,#19831,#19832,#19833,#19834,#19835,#19836,#19837,#19838,#19839,
#19840,#19841,#19842,#19843,#19844,#19845,#19846,#19847,#19848,#19849,#19850,
#19851,#19852,#19853,#19854,#19855,#19856,#19857,#19858,#19859,#19860,#19861,
#19862,#19863,#19864,#19865,#19866,#19867,#19868,#19869,#19870,#19871,#19872,
#19873,#19874,#19875,#19876,#19877,#19878,#19879,#19880,#19881,#19882,#19883,
#19884,#19885,#19886,#19887,#19888,#19889,#19890),.UNSPECIFIED.,.F.,.F.)
B_SPLINE_CURVE_WITH_KNOTS((6,1,1,1,1,1,1,1,1,1,1,1,1,1,1,1,1,1,1,1,1,1,
1,1,1,1,1,1,1,1,1,1,1,1,1,1,1,1,1,1,1,1,1,1,1,1,1,1,1,1,1,1,1,1,1,1,1,1,
1,1,1,1,1,1,1,6),(0.,0.0153846153846154,0.0307692307692308,0.0461538461538462,
0.0615384615384615,0.0769230769230769,0.0923076923076923,0.107692307692308,
0.123076923076923,0.138461538461538,0.153846153846154,0.169230769230769,
0.184615384615385,0.2,0.215384615384615,0.230769230769231,0.246153846153846,
0.261538461538462,0.276923076923077,0.292307692307692,0.307692307692308,
0.323076923076923,0.338461538461538,0.353846153846154,0.369230769230769,
0.384615384615385,0.4,0.415384615384615,0.430769230769231,0.446153846153846,
0.461538461538462,0.476923076923077,0.492307692307692,0.507692307692308,
0.523076923076923,0.538461538461538,0.553846153846154,0.569230769230769,
0.584615384615384,0.6,0.615384615384615,0.63076923076923,0.646153846153846,
0.661538461538461,0.676923076923076,0.692307692307692,0.707692307692307,
0.723076923076922,0.738461538461538,0.753846153846153,0.769230769230768,
0.784615384615384,0.799999999999999,0.815384615384614,0.83076923076923,
0.846153846153845,0.86153846153846,0.876923076923076,0.892307692307691,
0.907692307692306,0.923076923076922,0.938461538461537,0.953846153846152,
0.969230769230768,0.984615384615383,1.),.UNSPECIFIED.)
CURVE()
GEOMETRIC_REPRESENTATION_ITEM()
RATIONAL_B_SPLINE_CURVE((1.,1.,1.,1.,1.,1.,1.,1.,1.,1.,1.,1.,1.,1.,1.,1.,
1.,1.,1.,1.,1.,1.,1.,1.,1.,1.,1.,1.,1.,1.,1.,1.,1.,1.,1.,1.,1.,1.,1.,1.,
1.,1.,1.,1.,1.,1.,1.,1.,1.,1.,1.,1.,1.,1.,1.,1.,1.,1.,1.,1.,1.,1.,1.,1.,
1.,1.,1.,1.,1.,1.))
REPRESENTATION_ITEM('')
);
#154=(
BOUNDED_CURVE()
B_SPLINE_CURVE(5,(#19894,#19895,#19896,#19897,#19898,#19899,#19900,#19901,
#19902,#19903,#19904,#19905,#19906,#19907,#19908,#19909,#19910,#19911,#19912,
#19913,#19914,#19915,#19916,#19917,#19918,#19919,#19920,#19921,#19922,#19923,
#19924,#19925,#19926,#19927,#19928,#19929,#19930,#19931,#19932,#19933,#19934,
#19935,#19936,#19937,#19938,#19939,#19940,#19941,#19942,#19943,#19944,#19945,
#19946,#19947,#19948,#19949,#19950,#19951,#19952,#19953,#19954,#19955,#19956,
#19957,#19958,#19959,#19960,#19961,#19962,#19963),.UNSPECIFIED.,.F.,.F.)
B_SPLINE_CURVE_WITH_KNOTS((6,1,1,1,1,1,1,1,1,1,1,1,1,1,1,1,1,1,1,1,1,1,
1,1,1,1,1,1,1,1,1,1,1,1,1,1,1,1,1,1,1,1,1,1,1,1,1,1,1,1,1,1,1,1,1,1,1,1,
1,1,1,1,1,1,1,6),(0.,0.0153846153846154,0.0307692307692308,0.0461538461538462,
0.0615384615384615,0.0769230769230769,0.0923076923076923,0.107692307692308,
0.123076923076923,0.138461538461538,0.153846153846154,0.169230769230769,
0.184615384615385,0.2,0.215384615384615,0.230769230769231,0.246153846153846,
0.261538461538462,0.276923076923077,0.292307692307692,0.307692307692308,
0.323076923076923,0.338461538461538,0.353846153846154,0.369230769230769,
0.384615384615385,0.4,0.415384615384615,0.430769230769231,0.446153846153846,
0.461538461538462,0.476923076923077,0.492307692307692,0.507692307692308,
0.523076923076923,0.538461538461538,0.553846153846154,0.569230769230769,
0.584615384615384,0.6,0.615384615384615,0.63076923076923,0.646153846153846,
0.661538461538461,0.676923076923076,0.692307692307692,0.707692307692307,
0.723076923076922,0.738461538461538,0.753846153846153,0.769230769230768,
0.784615384615384,0.799999999999999,0.815384615384614,0.83076923076923,
0.846153846153845,0.86153846153846,0.876923076923076,0.892307692307691,
0.907692307692306,0.923076923076922,0.938461538461537,0.953846153846152,
0.969230769230768,0.984615384615383,1.),.UNSPECIFIED.)
CURVE()
GEOMETRIC_REPRESENTATION_ITEM()
RATIONAL_B_SPLINE_CURVE((1.,1.,1.,1.,1.,1.,1.,1.,1.,1.,1.,1.,1.,1.,1.,1.,
1.,1.,1.,1.,1.,1.,1.,1.,1.,1.,1.,1.,1.,1.,1.,1.,1.,1.,1.,1.,1.,1.,1.,1.,
1.,1.,1.,1.,1.,1.,1.,1.,1.,1.,1.,1.,1.,1.,1.,1.,1.,1.,1.,1.,1.,1.,1.,1.,
1.,1.,1.,1.,1.,1.))
REPRESENTATION_ITEM('')
);
#155=(
BOUNDED_CURVE()
B_SPLINE_CURVE(5,(#19967,#19968,#19969,#19970,#19971,#19972,#19973,#19974,
#19975,#19976,#19977,#19978,#19979,#19980,#19981,#19982,#19983,#19984,#19985,
#19986,#19987,#19988,#19989,#19990,#19991,#19992,#19993,#19994,#19995,#19996,
#19997,#19998,#19999,#20000,#20001,#20002,#20003,#20004,#20005,#20006,#20007,
#20008,#20009,#20010,#20011,#20012,#20013,#20014,#20015,#20016,#20017,#20018,
#20019,#20020,#20021,#20022,#20023,#20024,#20025,#20026,#20027,#20028,#20029,
#20030,#20031,#20032,#20033,#20034,#20035,#20036),.UNSPECIFIED.,.F.,.F.)
B_SPLINE_CURVE_WITH_KNOTS((6,1,1,1,1,1,1,1,1,1,1,1,1,1,1,1,1,1,1,1,1,1,
1,1,1,1,1,1,1,1,1,1,1,1,1,1,1,1,1,1,1,1,1,1,1,1,1,1,1,1,1,1,1,1,1,1,1,1,
1,1,1,1,1,1,1,6),(0.,0.0153846153846154,0.0307692307692308,0.0461538461538462,
0.0615384615384615,0.0769230769230769,0.0923076923076923,0.107692307692308,
0.123076923076923,0.138461538461538,0.153846153846154,0.169230769230769,
0.184615384615385,0.2,0.215384615384615,0.230769230769231,0.246153846153846,
0.261538461538462,0.276923076923077,0.292307692307692,0.307692307692308,
0.323076923076923,0.338461538461538,0.353846153846154,0.369230769230769,
0.384615384615385,0.4,0.415384615384615,0.430769230769231,0.446153846153846,
0.461538461538462,0.476923076923077,0.492307692307692,0.507692307692308,
0.523076923076923,0.538461538461538,0.553846153846154,0.569230769230769,
0.584615384615384,0.6,0.615384615384615,0.63076923076923,0.646153846153846,
0.661538461538461,0.676923076923076,0.692307692307692,0.707692307692307,
0.723076923076922,0.738461538461538,0.753846153846153,0.769230769230768,
0.784615384615384,0.799999999999999,0.815384615384614,0.83076923076923,
0.846153846153845,0.86153846153846,0.876923076923076,0.892307692307691,
0.907692307692306,0.923076923076922,0.938461538461537,0.953846153846152,
0.969230769230768,0.984615384615383,1.),.UNSPECIFIED.)
CURVE()
GEOMETRIC_REPRESENTATION_ITEM()
RATIONAL_B_SPLINE_CURVE((1.,1.,1.,1.,1.,1.,1.,1.,1.,1.,1.,1.,1.,1.,1.,1.,
1.,1.,1.,1.,1.,1.,1.,1.,1.,1.,1.,1.,1.,1.,1.,1.,1.,1.,1.,1.,1.,1.,1.,1.,
1.,1.,1.,1.,1.,1.,1.,1.,1.,1.,1.,1.,1.,1.,1.,1.,1.,1.,1.,1.,1.,1.,1.,1.,
1.,1.,1.,1.,1.,1.))
REPRESENTATION_ITEM('')
);
#156=(
BOUNDED_CURVE()
B_SPLINE_CURVE(5,(#20040,#20041,#20042,#20043,#20044,#20045,#20046,#20047,
#20048,#20049,#20050,#20051,#20052,#20053,#20054,#20055,#20056,#20057,#20058,
#20059,#20060,#20061,#20062,#20063,#20064,#20065,#20066,#20067,#20068,#20069,
#20070,#20071,#20072,#20073,#20074,#20075,#20076,#20077,#20078,#20079,#20080,
#20081,#20082,#20083,#20084,#20085,#20086,#20087,#20088,#20089,#20090,#20091,
#20092,#20093,#20094,#20095,#20096,#20097,#20098,#20099,#20100,#20101,#20102,
#20103,#20104,#20105,#20106,#20107,#20108,#20109),.UNSPECIFIED.,.F.,.F.)
B_SPLINE_CURVE_WITH_KNOTS((6,1,1,1,1,1,1,1,1,1,1,1,1,1,1,1,1,1,1,1,1,1,
1,1,1,1,1,1,1,1,1,1,1,1,1,1,1,1,1,1,1,1,1,1,1,1,1,1,1,1,1,1,1,1,1,1,1,1,
1,1,1,1,1,1,1,6),(0.,0.0153846153846154,0.0307692307692308,0.0461538461538462,
0.0615384615384615,0.0769230769230769,0.0923076923076923,0.107692307692308,
0.123076923076923,0.138461538461538,0.153846153846154,0.169230769230769,
0.184615384615385,0.2,0.215384615384615,0.230769230769231,0.246153846153846,
0.261538461538462,0.276923076923077,0.292307692307692,0.307692307692308,
0.323076923076923,0.338461538461538,0.353846153846154,0.369230769230769,
0.384615384615385,0.4,0.415384615384615,0.430769230769231,0.446153846153846,
0.461538461538462,0.476923076923077,0.492307692307692,0.507692307692308,
0.523076923076923,0.538461538461538,0.553846153846154,0.569230769230769,
0.584615384615384,0.6,0.615384615384615,0.63076923076923,0.646153846153846,
0.661538461538461,0.676923076923076,0.692307692307692,0.707692307692307,
0.723076923076922,0.738461538461538,0.753846153846153,0.769230769230768,
0.784615384615384,0.799999999999999,0.815384615384614,0.83076923076923,
0.846153846153845,0.86153846153846,0.876923076923076,0.892307692307691,
0.907692307692306,0.923076923076922,0.938461538461537,0.953846153846152,
0.969230769230768,0.984615384615383,1.),.UNSPECIFIED.)
CURVE()
GEOMETRIC_REPRESENTATION_ITEM()
RATIONAL_B_SPLINE_CURVE((1.,1.,1.,1.,1.,1.,1.,1.,1.,1.,1.,1.,1.,1.,1.,1.,
1.,1.,1.,1.,1.,1.,1.,1.,1.,1.,1.,1.,1.,1.,1.,1.,1.,1.,1.,1.,1.,1.,1.,1.,
1.,1.,1.,1.,1.,1.,1.,1.,1.,1.,1.,1.,1.,1.,1.,1.,1.,1.,1.,1.,1.,1.,1.,1.,
1.,1.,1.,1.,1.,1.))
REPRESENTATION_ITEM('')
);
#157=(
BOUNDED_CURVE()
B_SPLINE_CURVE(5,(#20113,#20114,#20115,#20116,#20117,#20118,#20119,#20120,
#20121,#20122,#20123,#20124,#20125,#20126,#20127,#20128,#20129,#20130,#20131,
#20132,#20133,#20134,#20135,#20136,#20137,#20138,#20139,#20140,#20141,#20142,
#20143,#20144,#20145,#20146,#20147,#20148,#20149,#20150,#20151,#20152,#20153,
#20154,#20155,#20156,#20157,#20158,#20159,#20160,#20161,#20162,#20163,#20164,
#20165,#20166,#20167,#20168,#20169,#20170,#20171,#20172,#20173,#20174,#20175,
#20176,#20177,#20178,#20179,#20180,#20181,#20182),.UNSPECIFIED.,.F.,.F.)
B_SPLINE_CURVE_WITH_KNOTS((6,1,1,1,1,1,1,1,1,1,1,1,1,1,1,1,1,1,1,1,1,1,
1,1,1,1,1,1,1,1,1,1,1,1,1,1,1,1,1,1,1,1,1,1,1,1,1,1,1,1,1,1,1,1,1,1,1,1,
1,1,1,1,1,1,1,6),(0.,0.0153846153846154,0.0307692307692308,0.0461538461538462,
0.0615384615384615,0.0769230769230769,0.0923076923076923,0.107692307692308,
0.123076923076923,0.138461538461538,0.153846153846154,0.169230769230769,
0.184615384615385,0.2,0.215384615384615,0.230769230769231,0.246153846153846,
0.261538461538462,0.276923076923077,0.292307692307692,0.307692307692308,
0.323076923076923,0.338461538461538,0.353846153846154,0.369230769230769,
0.384615384615385,0.4,0.415384615384615,0.430769230769231,0.446153846153846,
0.461538461538462,0.476923076923077,0.492307692307692,0.507692307692308,
0.523076923076923,0.538461538461538,0.553846153846154,0.569230769230769,
0.584615384615384,0.6,0.615384615384615,0.63076923076923,0.646153846153846,
0.661538461538461,0.676923076923076,0.692307692307692,0.707692307692307,
0.723076923076922,0.738461538461538,0.753846153846153,0.769230769230768,
0.784615384615384,0.799999999999999,0.815384615384614,0.83076923076923,
0.846153846153845,0.86153846153846,0.876923076923076,0.892307692307691,
0.907692307692306,0.923076923076922,0.938461538461537,0.953846153846152,
0.969230769230768,0.984615384615383,1.),.UNSPECIFIED.)
CURVE()
GEOMETRIC_REPRESENTATION_ITEM()
RATIONAL_B_SPLINE_CURVE((1.,1.,1.,1.,1.,1.,1.,1.,1.,1.,1.,1.,1.,1.,1.,1.,
1.,1.,1.,1.,1.,1.,1.,1.,1.,1.,1.,1.,1.,1.,1.,1.,1.,1.,1.,1.,1.,1.,1.,1.,
1.,1.,1.,1.,1.,1.,1.,1.,1.,1.,1.,1.,1.,1.,1.,1.,1.,1.,1.,1.,1.,1.,1.,1.,
1.,1.,1.,1.,1.,1.))
REPRESENTATION_ITEM('')
);
#158=(
BOUNDED_CURVE()
B_SPLINE_CURVE(5,(#20186,#20187,#20188,#20189,#20190,#20191,#20192,#20193,
#20194,#20195,#20196,#20197,#20198,#20199,#20200,#20201,#20202,#20203,#20204,
#20205,#20206,#20207,#20208,#20209,#20210,#20211,#20212,#20213,#20214,#20215,
#20216,#20217,#20218,#20219,#20220,#20221,#20222,#20223,#20224,#20225,#20226,
#20227,#20228,#20229,#20230,#20231,#20232,#20233,#20234,#20235,#20236,#20237,
#20238,#20239,#20240,#20241,#20242,#20243,#20244,#20245,#20246,#20247,#20248,
#20249,#20250,#20251,#20252,#20253,#20254,#20255),.UNSPECIFIED.,.F.,.F.)
B_SPLINE_CURVE_WITH_KNOTS((6,1,1,1,1,1,1,1,1,1,1,1,1,1,1,1,1,1,1,1,1,1,
1,1,1,1,1,1,1,1,1,1,1,1,1,1,1,1,1,1,1,1,1,1,1,1,1,1,1,1,1,1,1,1,1,1,1,1,
1,1,1,1,1,1,1,6),(0.,0.0153846153846154,0.0307692307692308,0.0461538461538462,
0.0615384615384615,0.0769230769230769,0.0923076923076923,0.107692307692308,
0.123076923076923,0.138461538461538,0.153846153846154,0.169230769230769,
0.184615384615385,0.2,0.215384615384615,0.230769230769231,0.246153846153846,
0.261538461538462,0.276923076923077,0.292307692307692,0.307692307692308,
0.323076923076923,0.338461538461538,0.353846153846154,0.369230769230769,
0.384615384615385,0.4,0.415384615384615,0.430769230769231,0.446153846153846,
0.461538461538462,0.476923076923077,0.492307692307692,0.507692307692308,
0.523076923076923,0.538461538461538,0.553846153846154,0.569230769230769,
0.584615384615384,0.6,0.615384615384615,0.63076923076923,0.646153846153846,
0.661538461538461,0.676923076923076,0.692307692307692,0.707692307692307,
0.723076923076922,0.738461538461538,0.753846153846153,0.769230769230768,
0.784615384615384,0.799999999999999,0.815384615384614,0.83076923076923,
0.846153846153845,0.86153846153846,0.876923076923076,0.892307692307691,
0.907692307692306,0.923076923076922,0.938461538461537,0.953846153846152,
0.969230769230768,0.984615384615383,1.),.UNSPECIFIED.)
CURVE()
GEOMETRIC_REPRESENTATION_ITEM()
RATIONAL_B_SPLINE_CURVE((1.,1.,1.,1.,1.,1.,1.,1.,1.,1.,1.,1.,1.,1.,1.,1.,
1.,1.,1.,1.,1.,1.,1.,1.,1.,1.,1.,1.,1.,1.,1.,1.,1.,1.,1.,1.,1.,1.,1.,1.,
1.,1.,1.,1.,1.,1.,1.,1.,1.,1.,1.,1.,1.,1.,1.,1.,1.,1.,1.,1.,1.,1.,1.,1.,
1.,1.,1.,1.,1.,1.))
REPRESENTATION_ITEM('')
);
#159=(
BOUNDED_CURVE()
B_SPLINE_CURVE(5,(#20259,#20260,#20261,#20262,#20263,#20264,#20265,#20266,
#20267,#20268,#20269,#20270,#20271,#20272,#20273,#20274,#20275,#20276,#20277,
#20278,#20279,#20280,#20281,#20282,#20283,#20284,#20285,#20286,#20287,#20288,
#20289,#20290,#20291,#20292,#20293,#20294,#20295,#20296,#20297,#20298,#20299,
#20300,#20301,#20302,#20303,#20304,#20305,#20306,#20307,#20308,#20309,#20310,
#20311,#20312,#20313,#20314,#20315,#20316,#20317,#20318,#20319,#20320,#20321,
#20322,#20323,#20324,#20325,#20326,#20327,#20328),.UNSPECIFIED.,.F.,.F.)
B_SPLINE_CURVE_WITH_KNOTS((6,1,1,1,1,1,1,1,1,1,1,1,1,1,1,1,1,1,1,1,1,1,
1,1,1,1,1,1,1,1,1,1,1,1,1,1,1,1,1,1,1,1,1,1,1,1,1,1,1,1,1,1,1,1,1,1,1,1,
1,1,1,1,1,1,1,6),(0.,0.0153846153846154,0.0307692307692308,0.0461538461538462,
0.0615384615384615,0.0769230769230769,0.0923076923076923,0.107692307692308,
0.123076923076923,0.138461538461538,0.153846153846154,0.169230769230769,
0.184615384615385,0.2,0.215384615384615,0.230769230769231,0.246153846153846,
0.261538461538462,0.276923076923077,0.292307692307692,0.307692307692308,
0.323076923076923,0.338461538461538,0.353846153846154,0.369230769230769,
0.384615384615385,0.4,0.415384615384615,0.430769230769231,0.446153846153846,
0.461538461538462,0.476923076923077,0.492307692307692,0.507692307692308,
0.523076923076923,0.538461538461538,0.553846153846154,0.569230769230769,
0.584615384615384,0.6,0.615384615384615,0.63076923076923,0.646153846153846,
0.661538461538461,0.676923076923076,0.692307692307692,0.707692307692307,
0.723076923076922,0.738461538461538,0.753846153846153,0.769230769230768,
0.784615384615384,0.799999999999999,0.815384615384614,0.83076923076923,
0.846153846153845,0.86153846153846,0.876923076923076,0.892307692307691,
0.907692307692306,0.923076923076922,0.938461538461537,0.953846153846152,
0.969230769230768,0.984615384615383,1.),.UNSPECIFIED.)
CURVE()
GEOMETRIC_REPRESENTATION_ITEM()
RATIONAL_B_SPLINE_CURVE((1.,1.,1.,1.,1.,1.,1.,1.,1.,1.,1.,1.,1.,1.,1.,1.,
1.,1.,1.,1.,1.,1.,1.,1.,1.,1.,1.,1.,1.,1.,1.,1.,1.,1.,1.,1.,1.,1.,1.,1.,
1.,1.,1.,1.,1.,1.,1.,1.,1.,1.,1.,1.,1.,1.,1.,1.,1.,1.,1.,1.,1.,1.,1.,1.,
1.,1.,1.,1.,1.,1.))
REPRESENTATION_ITEM('')
);
#160=(
BOUNDED_CURVE()
B_SPLINE_CURVE(5,(#20332,#20333,#20334,#20335,#20336,#20337,#20338,#20339,
#20340,#20341,#20342,#20343,#20344,#20345,#20346,#20347,#20348,#20349,#20350,
#20351,#20352,#20353,#20354,#20355,#20356,#20357,#20358,#20359,#20360,#20361,
#20362,#20363,#20364,#20365,#20366,#20367,#20368,#20369,#20370,#20371,#20372,
#20373,#20374,#20375,#20376,#20377,#20378,#20379,#20380,#20381,#20382,#20383,
#20384,#20385,#20386,#20387,#20388,#20389,#20390,#20391,#20392,#20393,#20394,
#20395,#20396,#20397,#20398,#20399,#20400,#20401),.UNSPECIFIED.,.F.,.F.)
B_SPLINE_CURVE_WITH_KNOTS((6,1,1,1,1,1,1,1,1,1,1,1,1,1,1,1,1,1,1,1,1,1,
1,1,1,1,1,1,1,1,1,1,1,1,1,1,1,1,1,1,1,1,1,1,1,1,1,1,1,1,1,1,1,1,1,1,1,1,
1,1,1,1,1,1,1,6),(0.,0.0153846153846154,0.0307692307692308,0.0461538461538462,
0.0615384615384615,0.0769230769230769,0.0923076923076923,0.107692307692308,
0.123076923076923,0.138461538461538,0.153846153846154,0.169230769230769,
0.184615384615385,0.2,0.215384615384615,0.230769230769231,0.246153846153846,
0.261538461538462,0.276923076923077,0.292307692307692,0.307692307692308,
0.323076923076923,0.338461538461538,0.353846153846154,0.369230769230769,
0.384615384615385,0.4,0.415384615384615,0.430769230769231,0.446153846153846,
0.461538461538462,0.476923076923077,0.492307692307692,0.507692307692308,
0.523076923076923,0.538461538461538,0.553846153846154,0.569230769230769,
0.584615384615384,0.6,0.615384615384615,0.63076923076923,0.646153846153846,
0.661538461538461,0.676923076923076,0.692307692307692,0.707692307692307,
0.723076923076922,0.738461538461538,0.753846153846153,0.769230769230768,
0.784615384615384,0.799999999999999,0.815384615384614,0.83076923076923,
0.846153846153845,0.86153846153846,0.876923076923076,0.892307692307691,
0.907692307692306,0.923076923076922,0.938461538461537,0.953846153846152,
0.969230769230768,0.984615384615383,1.),.UNSPECIFIED.)
CURVE()
GEOMETRIC_REPRESENTATION_ITEM()
RATIONAL_B_SPLINE_CURVE((1.,1.,1.,1.,1.,1.,1.,1.,1.,1.,1.,1.,1.,1.,1.,1.,
1.,1.,1.,1.,1.,1.,1.,1.,1.,1.,1.,1.,1.,1.,1.,1.,1.,1.,1.,1.,1.,1.,1.,1.,
1.,1.,1.,1.,1.,1.,1.,1.,1.,1.,1.,1.,1.,1.,1.,1.,1.,1.,1.,1.,1.,1.,1.,1.,
1.,1.,1.,1.,1.,1.))
REPRESENTATION_ITEM('')
);
#161=(
BOUNDED_CURVE()
B_SPLINE_CURVE(5,(#20405,#20406,#20407,#20408,#20409,#20410,#20411,#20412,
#20413,#20414,#20415,#20416,#20417,#20418,#20419,#20420,#20421,#20422,#20423,
#20424,#20425,#20426,#20427,#20428,#20429,#20430,#20431,#20432,#20433,#20434,
#20435,#20436,#20437,#20438,#20439,#20440,#20441,#20442,#20443,#20444,#20445,
#20446,#20447,#20448,#20449,#20450,#20451,#20452,#20453,#20454,#20455,#20456,
#20457,#20458,#20459,#20460,#20461,#20462,#20463,#20464,#20465,#20466,#20467,
#20468,#20469,#20470,#20471,#20472,#20473,#20474),.UNSPECIFIED.,.F.,.F.)
B_SPLINE_CURVE_WITH_KNOTS((6,1,1,1,1,1,1,1,1,1,1,1,1,1,1,1,1,1,1,1,1,1,
1,1,1,1,1,1,1,1,1,1,1,1,1,1,1,1,1,1,1,1,1,1,1,1,1,1,1,1,1,1,1,1,1,1,1,1,
1,1,1,1,1,1,1,6),(0.,0.0153846153846154,0.0307692307692308,0.0461538461538462,
0.0615384615384615,0.0769230769230769,0.0923076923076923,0.107692307692308,
0.123076923076923,0.138461538461538,0.153846153846154,0.169230769230769,
0.184615384615385,0.2,0.215384615384615,0.230769230769231,0.246153846153846,
0.261538461538462,0.276923076923077,0.292307692307692,0.307692307692308,
0.323076923076923,0.338461538461538,0.353846153846154,0.369230769230769,
0.384615384615385,0.4,0.415384615384615,0.430769230769231,0.446153846153846,
0.461538461538462,0.476923076923077,0.492307692307692,0.507692307692308,
0.523076923076923,0.538461538461538,0.553846153846154,0.569230769230769,
0.584615384615384,0.6,0.615384615384615,0.63076923076923,0.646153846153846,
0.661538461538461,0.676923076923076,0.692307692307692,0.707692307692307,
0.723076923076922,0.738461538461538,0.753846153846153,0.769230769230768,
0.784615384615384,0.799999999999999,0.815384615384614,0.83076923076923,
0.846153846153845,0.86153846153846,0.876923076923076,0.892307692307691,
0.907692307692306,0.923076923076922,0.938461538461537,0.953846153846152,
0.969230769230768,0.984615384615383,1.),.UNSPECIFIED.)
CURVE()
GEOMETRIC_REPRESENTATION_ITEM()
RATIONAL_B_SPLINE_CURVE((1.,1.,1.,1.,1.,1.,1.,1.,1.,1.,1.,1.,1.,1.,1.,1.,
1.,1.,1.,1.,1.,1.,1.,1.,1.,1.,1.,1.,1.,1.,1.,1.,1.,1.,1.,1.,1.,1.,1.,1.,
1.,1.,1.,1.,1.,1.,1.,1.,1.,1.,1.,1.,1.,1.,1.,1.,1.,1.,1.,1.,1.,1.,1.,1.,
1.,1.,1.,1.,1.,1.))
REPRESENTATION_ITEM('')
);
#162=(
BOUNDED_CURVE()
B_SPLINE_CURVE(5,(#20478,#20479,#20480,#20481,#20482,#20483,#20484,#20485,
#20486,#20487,#20488,#20489,#20490,#20491,#20492,#20493,#20494,#20495,#20496,
#20497,#20498,#20499,#20500,#20501,#20502,#20503,#20504,#20505,#20506,#20507,
#20508,#20509,#20510,#20511,#20512,#20513,#20514,#20515,#20516,#20517,#20518,
#20519,#20520,#20521,#20522,#20523,#20524,#20525,#20526,#20527,#20528,#20529,
#20530,#20531,#20532,#20533,#20534,#20535,#20536,#20537,#20538,#20539,#20540,
#20541,#20542,#20543,#20544,#20545,#20546,#20547),.UNSPECIFIED.,.F.,.F.)
B_SPLINE_CURVE_WITH_KNOTS((6,1,1,1,1,1,1,1,1,1,1,1,1,1,1,1,1,1,1,1,1,1,
1,1,1,1,1,1,1,1,1,1,1,1,1,1,1,1,1,1,1,1,1,1,1,1,1,1,1,1,1,1,1,1,1,1,1,1,
1,1,1,1,1,1,1,6),(0.,0.0153846153846154,0.0307692307692308,0.0461538461538462,
0.0615384615384615,0.0769230769230769,0.0923076923076923,0.107692307692308,
0.123076923076923,0.138461538461538,0.153846153846154,0.169230769230769,
0.184615384615385,0.2,0.215384615384615,0.230769230769231,0.246153846153846,
0.261538461538462,0.276923076923077,0.292307692307692,0.307692307692308,
0.323076923076923,0.338461538461538,0.353846153846154,0.369230769230769,
0.384615384615385,0.4,0.415384615384615,0.430769230769231,0.446153846153846,
0.461538461538462,0.476923076923077,0.492307692307692,0.507692307692308,
0.523076923076923,0.538461538461538,0.553846153846154,0.569230769230769,
0.584615384615384,0.6,0.615384615384615,0.63076923076923,0.646153846153846,
0.661538461538461,0.676923076923076,0.692307692307692,0.707692307692307,
0.723076923076922,0.738461538461538,0.753846153846153,0.769230769230768,
0.784615384615384,0.799999999999999,0.815384615384614,0.83076923076923,
0.846153846153845,0.86153846153846,0.876923076923076,0.892307692307691,
0.907692307692306,0.923076923076922,0.938461538461537,0.953846153846152,
0.969230769230768,0.984615384615383,1.),.UNSPECIFIED.)
CURVE()
GEOMETRIC_REPRESENTATION_ITEM()
RATIONAL_B_SPLINE_CURVE((1.,1.,1.,1.,1.,1.,1.,1.,1.,1.,1.,1.,1.,1.,1.,1.,
1.,1.,1.,1.,1.,1.,1.,1.,1.,1.,1.,1.,1.,1.,1.,1.,1.,1.,1.,1.,1.,1.,1.,1.,
1.,1.,1.,1.,1.,1.,1.,1.,1.,1.,1.,1.,1.,1.,1.,1.,1.,1.,1.,1.,1.,1.,1.,1.,
1.,1.,1.,1.,1.,1.))
REPRESENTATION_ITEM('')
);
#163=(
BOUNDED_CURVE()
B_SPLINE_CURVE(5,(#20551,#20552,#20553,#20554,#20555,#20556,#20557,#20558,
#20559,#20560,#20561,#20562,#20563,#20564,#20565,#20566,#20567,#20568,#20569,
#20570,#20571,#20572,#20573,#20574,#20575,#20576,#20577,#20578,#20579,#20580,
#20581,#20582,#20583,#20584,#20585,#20586,#20587,#20588,#20589,#20590,#20591,
#20592,#20593,#20594,#20595,#20596,#20597,#20598,#20599,#20600,#20601,#20602,
#20603,#20604,#20605,#20606,#20607,#20608,#20609,#20610,#20611,#20612,#20613,
#20614,#20615,#20616,#20617,#20618,#20619,#20620),.UNSPECIFIED.,.F.,.F.)
B_SPLINE_CURVE_WITH_KNOTS((6,1,1,1,1,1,1,1,1,1,1,1,1,1,1,1,1,1,1,1,1,1,
1,1,1,1,1,1,1,1,1,1,1,1,1,1,1,1,1,1,1,1,1,1,1,1,1,1,1,1,1,1,1,1,1,1,1,1,
1,1,1,1,1,1,1,6),(0.,0.0153846153846154,0.0307692307692308,0.0461538461538462,
0.0615384615384615,0.0769230769230769,0.0923076923076923,0.107692307692308,
0.123076923076923,0.138461538461538,0.153846153846154,0.169230769230769,
0.184615384615385,0.2,0.215384615384615,0.230769230769231,0.246153846153846,
0.261538461538462,0.276923076923077,0.292307692307692,0.307692307692308,
0.323076923076923,0.338461538461538,0.353846153846154,0.369230769230769,
0.384615384615385,0.4,0.415384615384615,0.430769230769231,0.446153846153846,
0.461538461538462,0.476923076923077,0.492307692307692,0.507692307692308,
0.523076923076923,0.538461538461538,0.553846153846154,0.569230769230769,
0.584615384615384,0.6,0.615384615384615,0.63076923076923,0.646153846153846,
0.661538461538461,0.676923076923076,0.692307692307692,0.707692307692307,
0.723076923076922,0.738461538461538,0.753846153846153,0.769230769230768,
0.784615384615384,0.799999999999999,0.815384615384614,0.83076923076923,
0.846153846153845,0.86153846153846,0.876923076923076,0.892307692307691,
0.907692307692306,0.923076923076922,0.938461538461537,0.953846153846152,
0.969230769230768,0.984615384615383,1.),.UNSPECIFIED.)
CURVE()
GEOMETRIC_REPRESENTATION_ITEM()
RATIONAL_B_SPLINE_CURVE((1.,1.,1.,1.,1.,1.,1.,1.,1.,1.,1.,1.,1.,1.,1.,1.,
1.,1.,1.,1.,1.,1.,1.,1.,1.,1.,1.,1.,1.,1.,1.,1.,1.,1.,1.,1.,1.,1.,1.,1.,
1.,1.,1.,1.,1.,1.,1.,1.,1.,1.,1.,1.,1.,1.,1.,1.,1.,1.,1.,1.,1.,1.,1.,1.,
1.,1.,1.,1.,1.,1.))
REPRESENTATION_ITEM('')
);
#164=(
BOUNDED_CURVE()
B_SPLINE_CURVE(5,(#20624,#20625,#20626,#20627,#20628,#20629,#20630,#20631,
#20632,#20633,#20634,#20635,#20636,#20637,#20638,#20639,#20640,#20641,#20642,
#20643,#20644,#20645,#20646,#20647,#20648,#20649,#20650,#20651,#20652,#20653,
#20654,#20655,#20656,#20657,#20658,#20659,#20660,#20661,#20662,#20663,#20664,
#20665,#20666,#20667,#20668,#20669,#20670,#20671,#20672,#20673,#20674,#20675,
#20676,#20677,#20678,#20679,#20680,#20681,#20682,#20683,#20684,#20685,#20686,
#20687,#20688,#20689,#20690,#20691,#20692,#20693),.UNSPECIFIED.,.F.,.F.)
B_SPLINE_CURVE_WITH_KNOTS((6,1,1,1,1,1,1,1,1,1,1,1,1,1,1,1,1,1,1,1,1,1,
1,1,1,1,1,1,1,1,1,1,1,1,1,1,1,1,1,1,1,1,1,1,1,1,1,1,1,1,1,1,1,1,1,1,1,1,
1,1,1,1,1,1,1,6),(0.,0.0153846153846154,0.0307692307692308,0.0461538461538462,
0.0615384615384615,0.0769230769230769,0.0923076923076923,0.107692307692308,
0.123076923076923,0.138461538461538,0.153846153846154,0.169230769230769,
0.184615384615385,0.2,0.215384615384615,0.230769230769231,0.246153846153846,
0.261538461538462,0.276923076923077,0.292307692307692,0.307692307692308,
0.323076923076923,0.338461538461538,0.353846153846154,0.369230769230769,
0.384615384615385,0.4,0.415384615384615,0.430769230769231,0.446153846153846,
0.461538461538462,0.476923076923077,0.492307692307692,0.507692307692308,
0.523076923076923,0.538461538461538,0.553846153846154,0.569230769230769,
0.584615384615384,0.6,0.615384615384615,0.63076923076923,0.646153846153846,
0.661538461538461,0.676923076923076,0.692307692307692,0.707692307692307,
0.723076923076922,0.738461538461538,0.753846153846153,0.769230769230768,
0.784615384615384,0.799999999999999,0.815384615384614,0.83076923076923,
0.846153846153845,0.86153846153846,0.876923076923076,0.892307692307691,
0.907692307692306,0.923076923076922,0.938461538461537,0.953846153846152,
0.969230769230768,0.984615384615383,1.),.UNSPECIFIED.)
CURVE()
GEOMETRIC_REPRESENTATION_ITEM()
RATIONAL_B_SPLINE_CURVE((1.,1.,1.,1.,1.,1.,1.,1.,1.,1.,1.,1.,1.,1.,1.,1.,
1.,1.,1.,1.,1.,1.,1.,1.,1.,1.,1.,1.,1.,1.,1.,1.,1.,1.,1.,1.,1.,1.,1.,1.,
1.,1.,1.,1.,1.,1.,1.,1.,1.,1.,1.,1.,1.,1.,1.,1.,1.,1.,1.,1.,1.,1.,1.,1.,
1.,1.,1.,1.,1.,1.))
REPRESENTATION_ITEM('')
);
#165=(
BOUNDED_CURVE()
B_SPLINE_CURVE(5,(#20697,#20698,#20699,#20700,#20701,#20702,#20703,#20704,
#20705,#20706,#20707,#20708,#20709,#20710,#20711,#20712,#20713,#20714,#20715,
#20716,#20717,#20718,#20719,#20720,#20721,#20722,#20723,#20724,#20725,#20726,
#20727,#20728,#20729,#20730,#20731,#20732,#20733,#20734,#20735,#20736,#20737,
#20738,#20739,#20740,#20741,#20742,#20743,#20744,#20745,#20746,#20747,#20748,
#20749,#20750,#20751,#20752,#20753,#20754,#20755,#20756,#20757,#20758,#20759,
#20760,#20761,#20762,#20763,#20764,#20765,#20766),.UNSPECIFIED.,.F.,.F.)
B_SPLINE_CURVE_WITH_KNOTS((6,1,1,1,1,1,1,1,1,1,1,1,1,1,1,1,1,1,1,1,1,1,
1,1,1,1,1,1,1,1,1,1,1,1,1,1,1,1,1,1,1,1,1,1,1,1,1,1,1,1,1,1,1,1,1,1,1,1,
1,1,1,1,1,1,1,6),(0.,0.0153846153846154,0.0307692307692308,0.0461538461538462,
0.0615384615384615,0.0769230769230769,0.0923076923076923,0.107692307692308,
0.123076923076923,0.138461538461538,0.153846153846154,0.169230769230769,
0.184615384615385,0.2,0.215384615384615,0.230769230769231,0.246153846153846,
0.261538461538462,0.276923076923077,0.292307692307692,0.307692307692308,
0.323076923076923,0.338461538461538,0.353846153846154,0.369230769230769,
0.384615384615385,0.4,0.415384615384615,0.430769230769231,0.446153846153846,
0.461538461538462,0.476923076923077,0.492307692307692,0.507692307692308,
0.523076923076923,0.538461538461538,0.553846153846154,0.569230769230769,
0.584615384615384,0.6,0.615384615384615,0.63076923076923,0.646153846153846,
0.661538461538461,0.676923076923076,0.692307692307692,0.707692307692307,
0.723076923076922,0.738461538461538,0.753846153846153,0.769230769230768,
0.784615384615384,0.799999999999999,0.815384615384614,0.83076923076923,
0.846153846153845,0.86153846153846,0.876923076923076,0.892307692307691,
0.907692307692306,0.923076923076922,0.938461538461537,0.953846153846152,
0.969230769230768,0.984615384615383,1.),.UNSPECIFIED.)
CURVE()
GEOMETRIC_REPRESENTATION_ITEM()
RATIONAL_B_SPLINE_CURVE((1.,1.,1.,1.,1.,1.,1.,1.,1.,1.,1.,1.,1.,1.,1.,1.,
1.,1.,1.,1.,1.,1.,1.,1.,1.,1.,1.,1.,1.,1.,1.,1.,1.,1.,1.,1.,1.,1.,1.,1.,
1.,1.,1.,1.,1.,1.,1.,1.,1.,1.,1.,1.,1.,1.,1.,1.,1.,1.,1.,1.,1.,1.,1.,1.,
1.,1.,1.,1.,1.,1.))
REPRESENTATION_ITEM('')
);
#166=(
BOUNDED_CURVE()
B_SPLINE_CURVE(5,(#20770,#20771,#20772,#20773,#20774,#20775,#20776,#20777,
#20778,#20779,#20780,#20781,#20782,#20783,#20784,#20785,#20786,#20787,#20788,
#20789,#20790,#20791,#20792,#20793,#20794,#20795,#20796,#20797,#20798,#20799,
#20800,#20801,#20802,#20803,#20804,#20805,#20806,#20807,#20808,#20809,#20810,
#20811,#20812,#20813,#20814,#20815,#20816,#20817,#20818,#20819,#20820,#20821,
#20822,#20823,#20824,#20825,#20826,#20827,#20828,#20829,#20830,#20831,#20832,
#20833,#20834,#20835,#20836,#20837,#20838,#20839),.UNSPECIFIED.,.F.,.F.)
B_SPLINE_CURVE_WITH_KNOTS((6,1,1,1,1,1,1,1,1,1,1,1,1,1,1,1,1,1,1,1,1,1,
1,1,1,1,1,1,1,1,1,1,1,1,1,1,1,1,1,1,1,1,1,1,1,1,1,1,1,1,1,1,1,1,1,1,1,1,
1,1,1,1,1,1,1,6),(0.,0.0153846153846154,0.0307692307692308,0.0461538461538462,
0.0615384615384615,0.0769230769230769,0.0923076923076923,0.107692307692308,
0.123076923076923,0.138461538461538,0.153846153846154,0.169230769230769,
0.184615384615385,0.2,0.215384615384615,0.230769230769231,0.246153846153846,
0.261538461538462,0.276923076923077,0.292307692307692,0.307692307692308,
0.323076923076923,0.338461538461538,0.353846153846154,0.369230769230769,
0.384615384615385,0.4,0.415384615384615,0.430769230769231,0.446153846153846,
0.461538461538462,0.476923076923077,0.492307692307692,0.507692307692308,
0.523076923076923,0.538461538461538,0.553846153846154,0.569230769230769,
0.584615384615384,0.6,0.615384615384615,0.63076923076923,0.646153846153846,
0.661538461538461,0.676923076923076,0.692307692307692,0.707692307692307,
0.723076923076922,0.738461538461538,0.753846153846153,0.769230769230768,
0.784615384615384,0.799999999999999,0.815384615384614,0.83076923076923,
0.846153846153845,0.86153846153846,0.876923076923076,0.892307692307691,
0.907692307692306,0.923076923076922,0.938461538461537,0.953846153846152,
0.969230769230768,0.984615384615383,1.),.UNSPECIFIED.)
CURVE()
GEOMETRIC_REPRESENTATION_ITEM()
RATIONAL_B_SPLINE_CURVE((1.,1.,1.,1.,1.,1.,1.,1.,1.,1.,1.,1.,1.,1.,1.,1.,
1.,1.,1.,1.,1.,1.,1.,1.,1.,1.,1.,1.,1.,1.,1.,1.,1.,1.,1.,1.,1.,1.,1.,1.,
1.,1.,1.,1.,1.,1.,1.,1.,1.,1.,1.,1.,1.,1.,1.,1.,1.,1.,1.,1.,1.,1.,1.,1.,
1.,1.,1.,1.,1.,1.))
REPRESENTATION_ITEM('')
);
#167=(
BOUNDED_CURVE()
B_SPLINE_CURVE(5,(#20843,#20844,#20845,#20846,#20847,#20848,#20849,#20850,
#20851,#20852,#20853,#20854,#20855,#20856,#20857,#20858,#20859,#20860,#20861,
#20862,#20863,#20864,#20865,#20866,#20867,#20868,#20869,#20870,#20871,#20872,
#20873,#20874,#20875,#20876,#20877,#20878,#20879,#20880,#20881,#20882,#20883,
#20884,#20885,#20886,#20887,#20888,#20889,#20890,#20891,#20892,#20893,#20894,
#20895,#20896,#20897,#20898,#20899,#20900,#20901,#20902,#20903,#20904,#20905,
#20906,#20907,#20908,#20909,#20910,#20911,#20912),.UNSPECIFIED.,.F.,.F.)
B_SPLINE_CURVE_WITH_KNOTS((6,1,1,1,1,1,1,1,1,1,1,1,1,1,1,1,1,1,1,1,1,1,
1,1,1,1,1,1,1,1,1,1,1,1,1,1,1,1,1,1,1,1,1,1,1,1,1,1,1,1,1,1,1,1,1,1,1,1,
1,1,1,1,1,1,1,6),(0.,0.0153846153846154,0.0307692307692308,0.0461538461538462,
0.0615384615384615,0.0769230769230769,0.0923076923076923,0.107692307692308,
0.123076923076923,0.138461538461538,0.153846153846154,0.169230769230769,
0.184615384615385,0.2,0.215384615384615,0.230769230769231,0.246153846153846,
0.261538461538462,0.276923076923077,0.292307692307692,0.307692307692308,
0.323076923076923,0.338461538461538,0.353846153846154,0.369230769230769,
0.384615384615385,0.4,0.415384615384615,0.430769230769231,0.446153846153846,
0.461538461538462,0.476923076923077,0.492307692307692,0.507692307692308,
0.523076923076923,0.538461538461538,0.553846153846154,0.569230769230769,
0.584615384615384,0.6,0.615384615384615,0.63076923076923,0.646153846153846,
0.661538461538461,0.676923076923076,0.692307692307692,0.707692307692307,
0.723076923076922,0.738461538461538,0.753846153846153,0.769230769230768,
0.784615384615384,0.799999999999999,0.815384615384614,0.83076923076923,
0.846153846153845,0.86153846153846,0.876923076923076,0.892307692307691,
0.907692307692306,0.923076923076922,0.938461538461537,0.953846153846152,
0.969230769230768,0.984615384615383,1.),.UNSPECIFIED.)
CURVE()
GEOMETRIC_REPRESENTATION_ITEM()
RATIONAL_B_SPLINE_CURVE((1.,1.,1.,1.,1.,1.,1.,1.,1.,1.,1.,1.,1.,1.,1.,1.,
1.,1.,1.,1.,1.,1.,1.,1.,1.,1.,1.,1.,1.,1.,1.,1.,1.,1.,1.,1.,1.,1.,1.,1.,
1.,1.,1.,1.,1.,1.,1.,1.,1.,1.,1.,1.,1.,1.,1.,1.,1.,1.,1.,1.,1.,1.,1.,1.,
1.,1.,1.,1.,1.,1.))
REPRESENTATION_ITEM('')
);
#168=(
BOUNDED_CURVE()
B_SPLINE_CURVE(5,(#20916,#20917,#20918,#20919,#20920,#20921,#20922,#20923,
#20924,#20925,#20926,#20927,#20928,#20929,#20930,#20931,#20932,#20933,#20934,
#20935,#20936,#20937,#20938,#20939,#20940,#20941,#20942,#20943,#20944,#20945,
#20946,#20947,#20948,#20949,#20950,#20951,#20952,#20953,#20954,#20955,#20956,
#20957,#20958,#20959,#20960,#20961,#20962,#20963,#20964,#20965,#20966,#20967,
#20968,#20969,#20970,#20971,#20972,#20973,#20974,#20975,#20976,#20977,#20978,
#20979,#20980,#20981,#20982,#20983,#20984,#20985),.UNSPECIFIED.,.F.,.F.)
B_SPLINE_CURVE_WITH_KNOTS((6,1,1,1,1,1,1,1,1,1,1,1,1,1,1,1,1,1,1,1,1,1,
1,1,1,1,1,1,1,1,1,1,1,1,1,1,1,1,1,1,1,1,1,1,1,1,1,1,1,1,1,1,1,1,1,1,1,1,
1,1,1,1,1,1,1,6),(0.,0.0153846153846154,0.0307692307692308,0.0461538461538462,
0.0615384615384615,0.0769230769230769,0.0923076923076923,0.107692307692308,
0.123076923076923,0.138461538461538,0.153846153846154,0.169230769230769,
0.184615384615385,0.2,0.215384615384615,0.230769230769231,0.246153846153846,
0.261538461538462,0.276923076923077,0.292307692307692,0.307692307692308,
0.323076923076923,0.338461538461538,0.353846153846154,0.369230769230769,
0.384615384615385,0.4,0.415384615384615,0.430769230769231,0.446153846153846,
0.461538461538462,0.476923076923077,0.492307692307692,0.507692307692308,
0.523076923076923,0.538461538461538,0.553846153846154,0.569230769230769,
0.584615384615384,0.6,0.615384615384615,0.63076923076923,0.646153846153846,
0.661538461538461,0.676923076923076,0.692307692307692,0.707692307692307,
0.723076923076922,0.738461538461538,0.753846153846153,0.769230769230768,
0.784615384615384,0.799999999999999,0.815384615384614,0.83076923076923,
0.846153846153845,0.86153846153846,0.876923076923076,0.892307692307691,
0.907692307692306,0.923076923076922,0.938461538461537,0.953846153846152,
0.969230769230768,0.984615384615383,1.),.UNSPECIFIED.)
CURVE()
GEOMETRIC_REPRESENTATION_ITEM()
RATIONAL_B_SPLINE_CURVE((1.,1.,1.,1.,1.,1.,1.,1.,1.,1.,1.,1.,1.,1.,1.,1.,
1.,1.,1.,1.,1.,1.,1.,1.,1.,1.,1.,1.,1.,1.,1.,1.,1.,1.,1.,1.,1.,1.,1.,1.,
1.,1.,1.,1.,1.,1.,1.,1.,1.,1.,1.,1.,1.,1.,1.,1.,1.,1.,1.,1.,1.,1.,1.,1.,
1.,1.,1.,1.,1.,1.))
REPRESENTATION_ITEM('')
);
#169=(
BOUNDED_CURVE()
B_SPLINE_CURVE(5,(#20989,#20990,#20991,#20992,#20993,#20994,#20995,#20996,
#20997,#20998,#20999,#21000,#21001,#21002,#21003,#21004,#21005,#21006,#21007,
#21008,#21009,#21010,#21011,#21012,#21013,#21014,#21015,#21016,#21017,#21018,
#21019,#21020,#21021,#21022,#21023,#21024,#21025,#21026,#21027,#21028,#21029,
#21030,#21031,#21032,#21033,#21034,#21035,#21036,#21037,#21038,#21039,#21040,
#21041,#21042,#21043,#21044,#21045,#21046,#21047,#21048,#21049,#21050,#21051,
#21052,#21053,#21054,#21055,#21056,#21057,#21058),.UNSPECIFIED.,.F.,.F.)
B_SPLINE_CURVE_WITH_KNOTS((6,1,1,1,1,1,1,1,1,1,1,1,1,1,1,1,1,1,1,1,1,1,
1,1,1,1,1,1,1,1,1,1,1,1,1,1,1,1,1,1,1,1,1,1,1,1,1,1,1,1,1,1,1,1,1,1,1,1,
1,1,1,1,1,1,1,6),(0.,0.0153846153846154,0.0307692307692308,0.0461538461538462,
0.0615384615384615,0.0769230769230769,0.0923076923076923,0.107692307692308,
0.123076923076923,0.138461538461538,0.153846153846154,0.169230769230769,
0.184615384615385,0.2,0.215384615384615,0.230769230769231,0.246153846153846,
0.261538461538462,0.276923076923077,0.292307692307692,0.307692307692308,
0.323076923076923,0.338461538461538,0.353846153846154,0.369230769230769,
0.384615384615385,0.4,0.415384615384615,0.430769230769231,0.446153846153846,
0.461538461538462,0.476923076923077,0.492307692307692,0.507692307692308,
0.523076923076923,0.538461538461538,0.553846153846154,0.569230769230769,
0.584615384615384,0.6,0.615384615384615,0.63076923076923,0.646153846153846,
0.661538461538461,0.676923076923076,0.692307692307692,0.707692307692307,
0.723076923076922,0.738461538461538,0.753846153846153,0.769230769230768,
0.784615384615384,0.799999999999999,0.815384615384614,0.83076923076923,
0.846153846153845,0.86153846153846,0.876923076923076,0.892307692307691,
0.907692307692306,0.923076923076922,0.938461538461537,0.953846153846152,
0.969230769230768,0.984615384615383,1.),.UNSPECIFIED.)
CURVE()
GEOMETRIC_REPRESENTATION_ITEM()
RATIONAL_B_SPLINE_CURVE((1.,1.,1.,1.,1.,1.,1.,1.,1.,1.,1.,1.,1.,1.,1.,1.,
1.,1.,1.,1.,1.,1.,1.,1.,1.,1.,1.,1.,1.,1.,1.,1.,1.,1.,1.,1.,1.,1.,1.,1.,
1.,1.,1.,1.,1.,1.,1.,1.,1.,1.,1.,1.,1.,1.,1.,1.,1.,1.,1.,1.,1.,1.,1.,1.,
1.,1.,1.,1.,1.,1.))
REPRESENTATION_ITEM('')
);
#170=(
BOUNDED_CURVE()
B_SPLINE_CURVE(5,(#21061,#21062,#21063,#21064,#21065,#21066,#21067,#21068,
#21069,#21070,#21071,#21072,#21073,#21074,#21075,#21076,#21077,#21078,#21079,
#21080,#21081,#21082,#21083,#21084,#21085,#21086,#21087,#21088,#21089,#21090,
#21091,#21092,#21093,#21094,#21095,#21096,#21097,#21098,#21099,#21100,#21101,
#21102,#21103,#21104,#21105,#21106,#21107,#21108,#21109,#21110,#21111,#21112,
#21113,#21114,#21115,#21116,#21117,#21118,#21119,#21120,#21121,#21122,#21123,
#21124,#21125,#21126,#21127,#21128,#21129,#21130),.UNSPECIFIED.,.F.,.F.)
B_SPLINE_CURVE_WITH_KNOTS((6,1,1,1,1,1,1,1,1,1,1,1,1,1,1,1,1,1,1,1,1,1,
1,1,1,1,1,1,1,1,1,1,1,1,1,1,1,1,1,1,1,1,1,1,1,1,1,1,1,1,1,1,1,1,1,1,1,1,
1,1,1,1,1,1,1,6),(0.,0.0153846153846154,0.0307692307692308,0.0461538461538462,
0.0615384615384615,0.0769230769230769,0.0923076923076923,0.107692307692308,
0.123076923076923,0.138461538461538,0.153846153846154,0.169230769230769,
0.184615384615385,0.2,0.215384615384615,0.230769230769231,0.246153846153846,
0.261538461538462,0.276923076923077,0.292307692307692,0.307692307692308,
0.323076923076923,0.338461538461538,0.353846153846154,0.369230769230769,
0.384615384615385,0.4,0.415384615384615,0.430769230769231,0.446153846153846,
0.461538461538462,0.476923076923077,0.492307692307692,0.507692307692308,
0.523076923076923,0.538461538461538,0.553846153846154,0.569230769230769,
0.584615384615384,0.6,0.615384615384615,0.63076923076923,0.646153846153846,
0.661538461538461,0.676923076923076,0.692307692307692,0.707692307692307,
0.723076923076922,0.738461538461538,0.753846153846153,0.769230769230768,
0.784615384615384,0.799999999999999,0.815384615384614,0.83076923076923,
0.846153846153845,0.86153846153846,0.876923076923076,0.892307692307691,
0.907692307692306,0.923076923076922,0.938461538461537,0.953846153846152,
0.969230769230768,0.984615384615383,1.),.UNSPECIFIED.)
CURVE()
GEOMETRIC_REPRESENTATION_ITEM()
RATIONAL_B_SPLINE_CURVE((1.,1.,1.,1.,1.,1.,1.,1.,1.,1.,1.,1.,1.,1.,1.,1.,
1.,1.,1.,1.,1.,1.,1.,1.,1.,1.,1.,1.,1.,1.,1.,1.,1.,1.,1.,1.,1.,1.,1.,1.,
1.,1.,1.,1.,1.,1.,1.,1.,1.,1.,1.,1.,1.,1.,1.,1.,1.,1.,1.,1.,1.,1.,1.,1.,
1.,1.,1.,1.,1.,1.))
REPRESENTATION_ITEM('')
);
#171=(
BOUNDED_CURVE()
B_SPLINE_CURVE(5,(#21284,#21285,#21286,#21287,#21288,#21289,#21290,#21291,
#21292,#21293,#21294,#21295,#21296,#21297,#21298,#21299,#21300,#21301,#21302,
#21303,#21304,#21305,#21306,#21307,#21308,#21309,#21310,#21311,#21312,#21313,
#21314,#21315,#21316,#21317,#21318,#21319,#21320,#21321,#21322,#21323,#21324,
#21325,#21326,#21327,#21328,#21329,#21330,#21331,#21332,#21333,#21334,#21335,
#21336,#21337,#21338,#21339,#21340,#21341,#21342,#21343,#21344,#21345,#21346,
#21347,#21348,#21349,#21350,#21351,#21352,#21353),.UNSPECIFIED.,.F.,.F.)
B_SPLINE_CURVE_WITH_KNOTS((6,1,1,1,1,1,1,1,1,1,1,1,1,1,1,1,1,1,1,1,1,1,
1,1,1,1,1,1,1,1,1,1,1,1,1,1,1,1,1,1,1,1,1,1,1,1,1,1,1,1,1,1,1,1,1,1,1,1,
1,1,1,1,1,1,1,6),(-1.,-0.984615384615383,-0.969230769230768,-0.953846153846152,
-0.938461538461537,-0.923076923076922,-0.907692307692306,-0.892307692307691,
-0.876923076923076,-0.86153846153846,-0.846153846153845,-0.83076923076923,
-0.815384615384614,-0.799999999999999,-0.784615384615384,-0.769230769230768,
-0.753846153846153,-0.738461538461538,-0.723076923076922,-0.707692307692307,
-0.692307692307692,-0.676923076923076,-0.661538461538461,-0.646153846153846,
-0.63076923076923,-0.615384615384615,-0.6,-0.584615384615384,-0.569230769230769,
-0.553846153846154,-0.538461538461538,-0.523076923076923,-0.507692307692308,
-0.492307692307692,-0.476923076923077,-0.461538461538462,-0.446153846153846,
-0.430769230769231,-0.415384615384615,-0.4,-0.384615384615385,-0.369230769230769,
-0.353846153846154,-0.338461538461538,-0.323076923076923,-0.307692307692308,
-0.292307692307692,-0.276923076923077,-0.261538461538462,-0.246153846153846,
-0.230769230769231,-0.215384615384615,-0.2,-0.184615384615385,-0.169230769230769,
-0.153846153846154,-0.138461538461538,-0.123076923076923,-0.107692307692308,
-0.0923076923076923,-0.0769230769230769,-0.0615384615384615,-0.0461538461538462,
-0.0307692307692308,-0.0153846153846154,0.),.UNSPECIFIED.)
CURVE()
GEOMETRIC_REPRESENTATION_ITEM()
RATIONAL_B_SPLINE_CURVE((1.,1.,1.,1.,1.,1.,1.,1.,1.,1.,1.,1.,1.,1.,1.,1.,
1.,1.,1.,1.,1.,1.,1.,1.,1.,1.,1.,1.,1.,1.,1.,1.,1.,1.,1.,1.,1.,1.,1.,1.,
1.,1.,1.,1.,1.,1.,1.,1.,1.,1.,1.,1.,1.,1.,1.,1.,1.,1.,1.,1.,1.,1.,1.,1.,
1.,1.,1.,1.,1.,1.))
REPRESENTATION_ITEM('')
);
#172=(
BOUNDED_CURVE()
B_SPLINE_CURVE(5,(#21500,#21501,#21502,#21503,#21504,#21505,#21506,#21507,
#21508,#21509,#21510,#21511,#21512,#21513,#21514,#21515,#21516,#21517,#21518,
#21519,#21520,#21521,#21522,#21523,#21524,#21525,#21526,#21527,#21528,#21529,
#21530,#21531,#21532,#21533,#21534,#21535,#21536,#21537,#21538,#21539,#21540,
#21541,#21542,#21543,#21544,#21545,#21546,#21547,#21548,#21549,#21550,#21551,
#21552,#21553,#21554,#21555,#21556,#21557,#21558,#21559,#21560,#21561,#21562,
#21563,#21564,#21565,#21566,#21567,#21568,#21569),.UNSPECIFIED.,.F.,.F.)
B_SPLINE_CURVE_WITH_KNOTS((6,1,1,1,1,1,1,1,1,1,1,1,1,1,1,1,1,1,1,1,1,1,
1,1,1,1,1,1,1,1,1,1,1,1,1,1,1,1,1,1,1,1,1,1,1,1,1,1,1,1,1,1,1,1,1,1,1,1,
1,1,1,1,1,1,1,6),(-1.,-0.984615384615383,-0.969230769230768,-0.953846153846152,
-0.938461538461537,-0.923076923076922,-0.907692307692306,-0.892307692307691,
-0.876923076923076,-0.86153846153846,-0.846153846153845,-0.83076923076923,
-0.815384615384614,-0.799999999999999,-0.784615384615384,-0.769230769230768,
-0.753846153846153,-0.738461538461538,-0.723076923076922,-0.707692307692307,
-0.692307692307692,-0.676923076923076,-0.661538461538461,-0.646153846153846,
-0.63076923076923,-0.615384615384615,-0.6,-0.584615384615384,-0.569230769230769,
-0.553846153846154,-0.538461538461538,-0.523076923076923,-0.507692307692308,
-0.492307692307692,-0.476923076923077,-0.461538461538462,-0.446153846153846,
-0.430769230769231,-0.415384615384615,-0.4,-0.384615384615385,-0.369230769230769,
-0.353846153846154,-0.338461538461538,-0.323076923076923,-0.307692307692308,
-0.292307692307692,-0.276923076923077,-0.261538461538462,-0.246153846153846,
-0.230769230769231,-0.215384615384615,-0.2,-0.184615384615385,-0.169230769230769,
-0.153846153846154,-0.138461538461538,-0.123076923076923,-0.107692307692308,
-0.0923076923076923,-0.0769230769230769,-0.0615384615384615,-0.0461538461538462,
-0.0307692307692308,-0.0153846153846154,0.),.UNSPECIFIED.)
CURVE()
GEOMETRIC_REPRESENTATION_ITEM()
RATIONAL_B_SPLINE_CURVE((1.,1.,1.,1.,1.,1.,1.,1.,1.,1.,1.,1.,1.,1.,1.,1.,
1.,1.,1.,1.,1.,1.,1.,1.,1.,1.,1.,1.,1.,1.,1.,1.,1.,1.,1.,1.,1.,1.,1.,1.,
1.,1.,1.,1.,1.,1.,1.,1.,1.,1.,1.,1.,1.,1.,1.,1.,1.,1.,1.,1.,1.,1.,1.,1.,
1.,1.,1.,1.,1.,1.))
REPRESENTATION_ITEM('')
);
#173=(
BOUNDED_CURVE()
B_SPLINE_CURVE(5,(#21716,#21717,#21718,#21719,#21720,#21721,#21722,#21723,
#21724,#21725,#21726,#21727,#21728,#21729,#21730,#21731,#21732,#21733,#21734,
#21735,#21736,#21737,#21738,#21739,#21740,#21741,#21742,#21743,#21744,#21745,
#21746,#21747,#21748,#21749,#21750,#21751,#21752,#21753,#21754,#21755,#21756,
#21757,#21758,#21759,#21760,#21761,#21762,#21763,#21764,#21765,#21766,#21767,
#21768,#21769,#21770,#21771,#21772,#21773,#21774,#21775,#21776,#21777,#21778,
#21779,#21780,#21781,#21782,#21783,#21784,#21785),.UNSPECIFIED.,.F.,.F.)
B_SPLINE_CURVE_WITH_KNOTS((6,1,1,1,1,1,1,1,1,1,1,1,1,1,1,1,1,1,1,1,1,1,
1,1,1,1,1,1,1,1,1,1,1,1,1,1,1,1,1,1,1,1,1,1,1,1,1,1,1,1,1,1,1,1,1,1,1,1,
1,1,1,1,1,1,1,6),(-1.,-0.984615384615383,-0.969230769230768,-0.953846153846152,
-0.938461538461537,-0.923076923076922,-0.907692307692306,-0.892307692307691,
-0.876923076923076,-0.86153846153846,-0.846153846153845,-0.83076923076923,
-0.815384615384614,-0.799999999999999,-0.784615384615384,-0.769230769230768,
-0.753846153846153,-0.738461538461538,-0.723076923076922,-0.707692307692307,
-0.692307692307692,-0.676923076923076,-0.661538461538461,-0.646153846153846,
-0.63076923076923,-0.615384615384615,-0.6,-0.584615384615384,-0.569230769230769,
-0.553846153846154,-0.538461538461538,-0.523076923076923,-0.507692307692308,
-0.492307692307692,-0.476923076923077,-0.461538461538462,-0.446153846153846,
-0.430769230769231,-0.415384615384615,-0.4,-0.384615384615385,-0.369230769230769,
-0.353846153846154,-0.338461538461538,-0.323076923076923,-0.307692307692308,
-0.292307692307692,-0.276923076923077,-0.261538461538462,-0.246153846153846,
-0.230769230769231,-0.215384615384615,-0.2,-0.184615384615385,-0.169230769230769,
-0.153846153846154,-0.138461538461538,-0.123076923076923,-0.107692307692308,
-0.0923076923076923,-0.0769230769230769,-0.0615384615384615,-0.0461538461538462,
-0.0307692307692308,-0.0153846153846154,0.),.UNSPECIFIED.)
CURVE()
GEOMETRIC_REPRESENTATION_ITEM()
RATIONAL_B_SPLINE_CURVE((1.,1.,1.,1.,1.,1.,1.,1.,1.,1.,1.,1.,1.,1.,1.,1.,
1.,1.,1.,1.,1.,1.,1.,1.,1.,1.,1.,1.,1.,1.,1.,1.,1.,1.,1.,1.,1.,1.,1.,1.,
1.,1.,1.,1.,1.,1.,1.,1.,1.,1.,1.,1.,1.,1.,1.,1.,1.,1.,1.,1.,1.,1.,1.,1.,
1.,1.,1.,1.,1.,1.))
REPRESENTATION_ITEM('')
);
#174=(
BOUNDED_CURVE()
B_SPLINE_CURVE(5,(#21932,#21933,#21934,#21935,#21936,#21937,#21938,#21939,
#21940,#21941,#21942,#21943,#21944,#21945,#21946,#21947,#21948,#21949,#21950,
#21951,#21952,#21953,#21954,#21955,#21956,#21957,#21958,#21959,#21960,#21961,
#21962,#21963,#21964,#21965,#21966,#21967,#21968,#21969,#21970,#21971,#21972,
#21973,#21974,#21975,#21976,#21977,#21978,#21979,#21980,#21981,#21982,#21983,
#21984,#21985,#21986,#21987,#21988,#21989,#21990,#21991,#21992,#21993,#21994,
#21995,#21996,#21997,#21998,#21999,#22000,#22001),.UNSPECIFIED.,.F.,.F.)
B_SPLINE_CURVE_WITH_KNOTS((6,1,1,1,1,1,1,1,1,1,1,1,1,1,1,1,1,1,1,1,1,1,
1,1,1,1,1,1,1,1,1,1,1,1,1,1,1,1,1,1,1,1,1,1,1,1,1,1,1,1,1,1,1,1,1,1,1,1,
1,1,1,1,1,1,1,6),(-1.,-0.984615384615383,-0.969230769230768,-0.953846153846152,
-0.938461538461537,-0.923076923076922,-0.907692307692306,-0.892307692307691,
-0.876923076923076,-0.86153846153846,-0.846153846153845,-0.83076923076923,
-0.815384615384614,-0.799999999999999,-0.784615384615384,-0.769230769230768,
-0.753846153846153,-0.738461538461538,-0.723076923076922,-0.707692307692307,
-0.692307692307692,-0.676923076923076,-0.661538461538461,-0.646153846153846,
-0.63076923076923,-0.615384615384615,-0.6,-0.584615384615384,-0.569230769230769,
-0.553846153846154,-0.538461538461538,-0.523076923076923,-0.507692307692308,
-0.492307692307692,-0.476923076923077,-0.461538461538462,-0.446153846153846,
-0.430769230769231,-0.415384615384615,-0.4,-0.384615384615385,-0.369230769230769,
-0.353846153846154,-0.338461538461538,-0.323076923076923,-0.307692307692308,
-0.292307692307692,-0.276923076923077,-0.261538461538462,-0.246153846153846,
-0.230769230769231,-0.215384615384615,-0.2,-0.184615384615385,-0.169230769230769,
-0.153846153846154,-0.138461538461538,-0.123076923076923,-0.107692307692308,
-0.0923076923076923,-0.0769230769230769,-0.0615384615384615,-0.0461538461538462,
-0.0307692307692308,-0.0153846153846154,0.),.UNSPECIFIED.)
CURVE()
GEOMETRIC_REPRESENTATION_ITEM()
RATIONAL_B_SPLINE_CURVE((1.,1.,1.,1.,1.,1.,1.,1.,1.,1.,1.,1.,1.,1.,1.,1.,
1.,1.,1.,1.,1.,1.,1.,1.,1.,1.,1.,1.,1.,1.,1.,1.,1.,1.,1.,1.,1.,1.,1.,1.,
1.,1.,1.,1.,1.,1.,1.,1.,1.,1.,1.,1.,1.,1.,1.,1.,1.,1.,1.,1.,1.,1.,1.,1.,
1.,1.,1.,1.,1.,1.))
REPRESENTATION_ITEM('')
);
#175=(
BOUNDED_CURVE()
B_SPLINE_CURVE(5,(#22148,#22149,#22150,#22151,#22152,#22153,#22154,#22155,
#22156,#22157,#22158,#22159,#22160,#22161,#22162,#22163,#22164,#22165,#22166,
#22167,#22168,#22169,#22170,#22171,#22172,#22173,#22174,#22175,#22176,#22177,
#22178,#22179,#22180,#22181,#22182,#22183,#22184,#22185,#22186,#22187,#22188,
#22189,#22190,#22191,#22192,#22193,#22194,#22195,#22196,#22197,#22198,#22199,
#22200,#22201,#22202,#22203,#22204,#22205,#22206,#22207,#22208,#22209,#22210,
#22211,#22212,#22213,#22214,#22215,#22216,#22217),.UNSPECIFIED.,.F.,.F.)
B_SPLINE_CURVE_WITH_KNOTS((6,1,1,1,1,1,1,1,1,1,1,1,1,1,1,1,1,1,1,1,1,1,
1,1,1,1,1,1,1,1,1,1,1,1,1,1,1,1,1,1,1,1,1,1,1,1,1,1,1,1,1,1,1,1,1,1,1,1,
1,1,1,1,1,1,1,6),(-1.,-0.984615384615383,-0.969230769230768,-0.953846153846152,
-0.938461538461537,-0.923076923076922,-0.907692307692306,-0.892307692307691,
-0.876923076923076,-0.86153846153846,-0.846153846153845,-0.83076923076923,
-0.815384615384614,-0.799999999999999,-0.784615384615384,-0.769230769230768,
-0.753846153846153,-0.738461538461538,-0.723076923076922,-0.707692307692307,
-0.692307692307692,-0.676923076923076,-0.661538461538461,-0.646153846153846,
-0.63076923076923,-0.615384615384615,-0.6,-0.584615384615384,-0.569230769230769,
-0.553846153846154,-0.538461538461538,-0.523076923076923,-0.507692307692308,
-0.492307692307692,-0.476923076923077,-0.461538461538462,-0.446153846153846,
-0.430769230769231,-0.415384615384615,-0.4,-0.384615384615385,-0.369230769230769,
-0.353846153846154,-0.338461538461538,-0.323076923076923,-0.307692307692308,
-0.292307692307692,-0.276923076923077,-0.261538461538462,-0.246153846153846,
-0.230769230769231,-0.215384615384615,-0.2,-0.184615384615385,-0.169230769230769,
-0.153846153846154,-0.138461538461538,-0.123076923076923,-0.107692307692308,
-0.0923076923076923,-0.0769230769230769,-0.0615384615384615,-0.0461538461538462,
-0.0307692307692308,-0.0153846153846154,0.),.UNSPECIFIED.)
CURVE()
GEOMETRIC_REPRESENTATION_ITEM()
RATIONAL_B_SPLINE_CURVE((1.,1.,1.,1.,1.,1.,1.,1.,1.,1.,1.,1.,1.,1.,1.,1.,
1.,1.,1.,1.,1.,1.,1.,1.,1.,1.,1.,1.,1.,1.,1.,1.,1.,1.,1.,1.,1.,1.,1.,1.,
1.,1.,1.,1.,1.,1.,1.,1.,1.,1.,1.,1.,1.,1.,1.,1.,1.,1.,1.,1.,1.,1.,1.,1.,
1.,1.,1.,1.,1.,1.))
REPRESENTATION_ITEM('')
);
#176=(
BOUNDED_CURVE()
B_SPLINE_CURVE(5,(#22364,#22365,#22366,#22367,#22368,#22369,#22370,#22371,
#22372,#22373,#22374,#22375,#22376,#22377,#22378,#22379,#22380,#22381,#22382,
#22383,#22384,#22385,#22386,#22387,#22388,#22389,#22390,#22391,#22392,#22393,
#22394,#22395,#22396,#22397,#22398,#22399,#22400,#22401,#22402,#22403,#22404,
#22405,#22406,#22407,#22408,#22409,#22410,#22411,#22412,#22413,#22414,#22415,
#22416,#22417,#22418,#22419,#22420,#22421,#22422,#22423,#22424,#22425,#22426,
#22427,#22428,#22429,#22430,#22431,#22432,#22433),.UNSPECIFIED.,.F.,.F.)
B_SPLINE_CURVE_WITH_KNOTS((6,1,1,1,1,1,1,1,1,1,1,1,1,1,1,1,1,1,1,1,1,1,
1,1,1,1,1,1,1,1,1,1,1,1,1,1,1,1,1,1,1,1,1,1,1,1,1,1,1,1,1,1,1,1,1,1,1,1,
1,1,1,1,1,1,1,6),(-1.,-0.984615384615383,-0.969230769230768,-0.953846153846152,
-0.938461538461537,-0.923076923076922,-0.907692307692306,-0.892307692307691,
-0.876923076923076,-0.86153846153846,-0.846153846153845,-0.83076923076923,
-0.815384615384614,-0.799999999999999,-0.784615384615384,-0.769230769230768,
-0.753846153846153,-0.738461538461538,-0.723076923076922,-0.707692307692307,
-0.692307692307692,-0.676923076923076,-0.661538461538461,-0.646153846153846,
-0.63076923076923,-0.615384615384615,-0.6,-0.584615384615384,-0.569230769230769,
-0.553846153846154,-0.538461538461538,-0.523076923076923,-0.507692307692308,
-0.492307692307692,-0.476923076923077,-0.461538461538462,-0.446153846153846,
-0.430769230769231,-0.415384615384615,-0.4,-0.384615384615385,-0.369230769230769,
-0.353846153846154,-0.338461538461538,-0.323076923076923,-0.307692307692308,
-0.292307692307692,-0.276923076923077,-0.261538461538462,-0.246153846153846,
-0.230769230769231,-0.215384615384615,-0.2,-0.184615384615385,-0.169230769230769,
-0.153846153846154,-0.138461538461538,-0.123076923076923,-0.107692307692308,
-0.0923076923076923,-0.0769230769230769,-0.0615384615384615,-0.0461538461538462,
-0.0307692307692308,-0.0153846153846154,0.),.UNSPECIFIED.)
CURVE()
GEOMETRIC_REPRESENTATION_ITEM()
RATIONAL_B_SPLINE_CURVE((1.,1.,1.,1.,1.,1.,1.,1.,1.,1.,1.,1.,1.,1.,1.,1.,
1.,1.,1.,1.,1.,1.,1.,1.,1.,1.,1.,1.,1.,1.,1.,1.,1.,1.,1.,1.,1.,1.,1.,1.,
1.,1.,1.,1.,1.,1.,1.,1.,1.,1.,1.,1.,1.,1.,1.,1.,1.,1.,1.,1.,1.,1.,1.,1.,
1.,1.,1.,1.,1.,1.))
REPRESENTATION_ITEM('')
);
#177=(
BOUNDED_CURVE()
B_SPLINE_CURVE(5,(#22580,#22581,#22582,#22583,#22584,#22585,#22586,#22587,
#22588,#22589,#22590,#22591,#22592,#22593,#22594,#22595,#22596,#22597,#22598,
#22599,#22600,#22601,#22602,#22603,#22604,#22605,#22606,#22607,#22608,#22609,
#22610,#22611,#22612,#22613,#22614,#22615,#22616,#22617,#22618,#22619,#22620,
#22621,#22622,#22623,#22624,#22625,#22626,#22627,#22628,#22629,#22630,#22631,
#22632,#22633,#22634,#22635,#22636,#22637,#22638,#22639,#22640,#22641,#22642,
#22643,#22644,#22645,#22646,#22647,#22648,#22649),.UNSPECIFIED.,.F.,.F.)
B_SPLINE_CURVE_WITH_KNOTS((6,1,1,1,1,1,1,1,1,1,1,1,1,1,1,1,1,1,1,1,1,1,
1,1,1,1,1,1,1,1,1,1,1,1,1,1,1,1,1,1,1,1,1,1,1,1,1,1,1,1,1,1,1,1,1,1,1,1,
1,1,1,1,1,1,1,6),(-1.,-0.984615384615383,-0.969230769230768,-0.953846153846152,
-0.938461538461537,-0.923076923076922,-0.907692307692306,-0.892307692307691,
-0.876923076923076,-0.86153846153846,-0.846153846153845,-0.83076923076923,
-0.815384615384614,-0.799999999999999,-0.784615384615384,-0.769230769230768,
-0.753846153846153,-0.738461538461538,-0.723076923076922,-0.707692307692307,
-0.692307692307692,-0.676923076923076,-0.661538461538461,-0.646153846153846,
-0.63076923076923,-0.615384615384615,-0.6,-0.584615384615384,-0.569230769230769,
-0.553846153846154,-0.538461538461538,-0.523076923076923,-0.507692307692308,
-0.492307692307692,-0.476923076923077,-0.461538461538462,-0.446153846153846,
-0.430769230769231,-0.415384615384615,-0.4,-0.384615384615385,-0.369230769230769,
-0.353846153846154,-0.338461538461538,-0.323076923076923,-0.307692307692308,
-0.292307692307692,-0.276923076923077,-0.261538461538462,-0.246153846153846,
-0.230769230769231,-0.215384615384615,-0.2,-0.184615384615385,-0.169230769230769,
-0.153846153846154,-0.138461538461538,-0.123076923076923,-0.107692307692308,
-0.0923076923076923,-0.0769230769230769,-0.0615384615384615,-0.0461538461538462,
-0.0307692307692308,-0.0153846153846154,0.),.UNSPECIFIED.)
CURVE()
GEOMETRIC_REPRESENTATION_ITEM()
RATIONAL_B_SPLINE_CURVE((1.,1.,1.,1.,1.,1.,1.,1.,1.,1.,1.,1.,1.,1.,1.,1.,
1.,1.,1.,1.,1.,1.,1.,1.,1.,1.,1.,1.,1.,1.,1.,1.,1.,1.,1.,1.,1.,1.,1.,1.,
1.,1.,1.,1.,1.,1.,1.,1.,1.,1.,1.,1.,1.,1.,1.,1.,1.,1.,1.,1.,1.,1.,1.,1.,
1.,1.,1.,1.,1.,1.))
REPRESENTATION_ITEM('')
);
#178=(
BOUNDED_CURVE()
B_SPLINE_CURVE(5,(#22796,#22797,#22798,#22799,#22800,#22801,#22802,#22803,
#22804,#22805,#22806,#22807,#22808,#22809,#22810,#22811,#22812,#22813,#22814,
#22815,#22816,#22817,#22818,#22819,#22820,#22821,#22822,#22823,#22824,#22825,
#22826,#22827,#22828,#22829,#22830,#22831,#22832,#22833,#22834,#22835,#22836,
#22837,#22838,#22839,#22840,#22841,#22842,#22843,#22844,#22845,#22846,#22847,
#22848,#22849,#22850,#22851,#22852,#22853,#22854,#22855,#22856,#22857,#22858,
#22859,#22860,#22861,#22862,#22863,#22864,#22865),.UNSPECIFIED.,.F.,.F.)
B_SPLINE_CURVE_WITH_KNOTS((6,1,1,1,1,1,1,1,1,1,1,1,1,1,1,1,1,1,1,1,1,1,
1,1,1,1,1,1,1,1,1,1,1,1,1,1,1,1,1,1,1,1,1,1,1,1,1,1,1,1,1,1,1,1,1,1,1,1,
1,1,1,1,1,1,1,6),(-1.,-0.984615384615383,-0.969230769230768,-0.953846153846152,
-0.938461538461537,-0.923076923076922,-0.907692307692306,-0.892307692307691,
-0.876923076923076,-0.86153846153846,-0.846153846153845,-0.83076923076923,
-0.815384615384614,-0.799999999999999,-0.784615384615384,-0.769230769230768,
-0.753846153846153,-0.738461538461538,-0.723076923076922,-0.707692307692307,
-0.692307692307692,-0.676923076923076,-0.661538461538461,-0.646153846153846,
-0.63076923076923,-0.615384615384615,-0.6,-0.584615384615384,-0.569230769230769,
-0.553846153846154,-0.538461538461538,-0.523076923076923,-0.507692307692308,
-0.492307692307692,-0.476923076923077,-0.461538461538462,-0.446153846153846,
-0.430769230769231,-0.415384615384615,-0.4,-0.384615384615385,-0.369230769230769,
-0.353846153846154,-0.338461538461538,-0.323076923076923,-0.307692307692308,
-0.292307692307692,-0.276923076923077,-0.261538461538462,-0.246153846153846,
-0.230769230769231,-0.215384615384615,-0.2,-0.184615384615385,-0.169230769230769,
-0.153846153846154,-0.138461538461538,-0.123076923076923,-0.107692307692308,
-0.0923076923076923,-0.0769230769230769,-0.0615384615384615,-0.0461538461538462,
-0.0307692307692308,-0.0153846153846154,0.),.UNSPECIFIED.)
CURVE()
GEOMETRIC_REPRESENTATION_ITEM()
RATIONAL_B_SPLINE_CURVE((1.,1.,1.,1.,1.,1.,1.,1.,1.,1.,1.,1.,1.,1.,1.,1.,
1.,1.,1.,1.,1.,1.,1.,1.,1.,1.,1.,1.,1.,1.,1.,1.,1.,1.,1.,1.,1.,1.,1.,1.,
1.,1.,1.,1.,1.,1.,1.,1.,1.,1.,1.,1.,1.,1.,1.,1.,1.,1.,1.,1.,1.,1.,1.,1.,
1.,1.,1.,1.,1.,1.))
REPRESENTATION_ITEM('')
);
#179=(
BOUNDED_CURVE()
B_SPLINE_CURVE(5,(#23012,#23013,#23014,#23015,#23016,#23017,#23018,#23019,
#23020,#23021,#23022,#23023,#23024,#23025,#23026,#23027,#23028,#23029,#23030,
#23031,#23032,#23033,#23034,#23035,#23036,#23037,#23038,#23039,#23040,#23041,
#23042,#23043,#23044,#23045,#23046,#23047,#23048,#23049,#23050,#23051,#23052,
#23053,#23054,#23055,#23056,#23057,#23058,#23059,#23060,#23061,#23062,#23063,
#23064,#23065,#23066,#23067,#23068,#23069,#23070,#23071,#23072,#23073,#23074,
#23075,#23076,#23077,#23078,#23079,#23080,#23081),.UNSPECIFIED.,.F.,.F.)
B_SPLINE_CURVE_WITH_KNOTS((6,1,1,1,1,1,1,1,1,1,1,1,1,1,1,1,1,1,1,1,1,1,
1,1,1,1,1,1,1,1,1,1,1,1,1,1,1,1,1,1,1,1,1,1,1,1,1,1,1,1,1,1,1,1,1,1,1,1,
1,1,1,1,1,1,1,6),(-1.,-0.984615384615383,-0.969230769230768,-0.953846153846152,
-0.938461538461537,-0.923076923076922,-0.907692307692306,-0.892307692307691,
-0.876923076923076,-0.86153846153846,-0.846153846153845,-0.83076923076923,
-0.815384615384614,-0.799999999999999,-0.784615384615384,-0.769230769230768,
-0.753846153846153,-0.738461538461538,-0.723076923076922,-0.707692307692307,
-0.692307692307692,-0.676923076923076,-0.661538461538461,-0.646153846153846,
-0.63076923076923,-0.615384615384615,-0.6,-0.584615384615384,-0.569230769230769,
-0.553846153846154,-0.538461538461538,-0.523076923076923,-0.507692307692308,
-0.492307692307692,-0.476923076923077,-0.461538461538462,-0.446153846153846,
-0.430769230769231,-0.415384615384615,-0.4,-0.384615384615385,-0.369230769230769,
-0.353846153846154,-0.338461538461538,-0.323076923076923,-0.307692307692308,
-0.292307692307692,-0.276923076923077,-0.261538461538462,-0.246153846153846,
-0.230769230769231,-0.215384615384615,-0.2,-0.184615384615385,-0.169230769230769,
-0.153846153846154,-0.138461538461538,-0.123076923076923,-0.107692307692308,
-0.0923076923076923,-0.0769230769230769,-0.0615384615384615,-0.0461538461538462,
-0.0307692307692308,-0.0153846153846154,0.),.UNSPECIFIED.)
CURVE()
GEOMETRIC_REPRESENTATION_ITEM()
RATIONAL_B_SPLINE_CURVE((1.,1.,1.,1.,1.,1.,1.,1.,1.,1.,1.,1.,1.,1.,1.,1.,
1.,1.,1.,1.,1.,1.,1.,1.,1.,1.,1.,1.,1.,1.,1.,1.,1.,1.,1.,1.,1.,1.,1.,1.,
1.,1.,1.,1.,1.,1.,1.,1.,1.,1.,1.,1.,1.,1.,1.,1.,1.,1.,1.,1.,1.,1.,1.,1.,
1.,1.,1.,1.,1.,1.))
REPRESENTATION_ITEM('')
);
#180=(
BOUNDED_CURVE()
B_SPLINE_CURVE(5,(#23228,#23229,#23230,#23231,#23232,#23233,#23234,#23235,
#23236,#23237,#23238,#23239,#23240,#23241,#23242,#23243,#23244,#23245,#23246,
#23247,#23248,#23249,#23250,#23251,#23252,#23253,#23254,#23255,#23256,#23257,
#23258,#23259,#23260,#23261,#23262,#23263,#23264,#23265,#23266,#23267,#23268,
#23269,#23270,#23271,#23272,#23273,#23274,#23275,#23276,#23277,#23278,#23279,
#23280,#23281,#23282,#23283,#23284,#23285,#23286,#23287,#23288,#23289,#23290,
#23291,#23292,#23293,#23294,#23295,#23296,#23297),.UNSPECIFIED.,.F.,.F.)
B_SPLINE_CURVE_WITH_KNOTS((6,1,1,1,1,1,1,1,1,1,1,1,1,1,1,1,1,1,1,1,1,1,
1,1,1,1,1,1,1,1,1,1,1,1,1,1,1,1,1,1,1,1,1,1,1,1,1,1,1,1,1,1,1,1,1,1,1,1,
1,1,1,1,1,1,1,6),(-1.,-0.984615384615383,-0.969230769230768,-0.953846153846152,
-0.938461538461537,-0.923076923076922,-0.907692307692306,-0.892307692307691,
-0.876923076923076,-0.86153846153846,-0.846153846153845,-0.83076923076923,
-0.815384615384614,-0.799999999999999,-0.784615384615384,-0.769230769230768,
-0.753846153846153,-0.738461538461538,-0.723076923076922,-0.707692307692307,
-0.692307692307692,-0.676923076923076,-0.661538461538461,-0.646153846153846,
-0.63076923076923,-0.615384615384615,-0.6,-0.584615384615384,-0.569230769230769,
-0.553846153846154,-0.538461538461538,-0.523076923076923,-0.507692307692308,
-0.492307692307692,-0.476923076923077,-0.461538461538462,-0.446153846153846,
-0.430769230769231,-0.415384615384615,-0.4,-0.384615384615385,-0.369230769230769,
-0.353846153846154,-0.338461538461538,-0.323076923076923,-0.307692307692308,
-0.292307692307692,-0.276923076923077,-0.261538461538462,-0.246153846153846,
-0.230769230769231,-0.215384615384615,-0.2,-0.184615384615385,-0.169230769230769,
-0.153846153846154,-0.138461538461538,-0.123076923076923,-0.107692307692308,
-0.0923076923076923,-0.0769230769230769,-0.0615384615384615,-0.0461538461538462,
-0.0307692307692308,-0.0153846153846154,0.),.UNSPECIFIED.)
CURVE()
GEOMETRIC_REPRESENTATION_ITEM()
RATIONAL_B_SPLINE_CURVE((1.,1.,1.,1.,1.,1.,1.,1.,1.,1.,1.,1.,1.,1.,1.,1.,
1.,1.,1.,1.,1.,1.,1.,1.,1.,1.,1.,1.,1.,1.,1.,1.,1.,1.,1.,1.,1.,1.,1.,1.,
1.,1.,1.,1.,1.,1.,1.,1.,1.,1.,1.,1.,1.,1.,1.,1.,1.,1.,1.,1.,1.,1.,1.,1.,
1.,1.,1.,1.,1.,1.))
REPRESENTATION_ITEM('')
);
#181=(
BOUNDED_CURVE()
B_SPLINE_CURVE(5,(#23444,#23445,#23446,#23447,#23448,#23449,#23450,#23451,
#23452,#23453,#23454,#23455,#23456,#23457,#23458,#23459,#23460,#23461,#23462,
#23463,#23464,#23465,#23466,#23467,#23468,#23469,#23470,#23471,#23472,#23473,
#23474,#23475,#23476,#23477,#23478,#23479,#23480,#23481,#23482,#23483,#23484,
#23485,#23486,#23487,#23488,#23489,#23490,#23491,#23492,#23493,#23494,#23495,
#23496,#23497,#23498,#23499,#23500,#23501,#23502,#23503,#23504,#23505,#23506,
#23507,#23508,#23509,#23510,#23511,#23512,#23513),.UNSPECIFIED.,.F.,.F.)
B_SPLINE_CURVE_WITH_KNOTS((6,1,1,1,1,1,1,1,1,1,1,1,1,1,1,1,1,1,1,1,1,1,
1,1,1,1,1,1,1,1,1,1,1,1,1,1,1,1,1,1,1,1,1,1,1,1,1,1,1,1,1,1,1,1,1,1,1,1,
1,1,1,1,1,1,1,6),(-1.,-0.984615384615383,-0.969230769230768,-0.953846153846152,
-0.938461538461537,-0.923076923076922,-0.907692307692306,-0.892307692307691,
-0.876923076923076,-0.86153846153846,-0.846153846153845,-0.83076923076923,
-0.815384615384614,-0.799999999999999,-0.784615384615384,-0.769230769230768,
-0.753846153846153,-0.738461538461538,-0.723076923076922,-0.707692307692307,
-0.692307692307692,-0.676923076923076,-0.661538461538461,-0.646153846153846,
-0.63076923076923,-0.615384615384615,-0.6,-0.584615384615384,-0.569230769230769,
-0.553846153846154,-0.538461538461538,-0.523076923076923,-0.507692307692308,
-0.492307692307692,-0.476923076923077,-0.461538461538462,-0.446153846153846,
-0.430769230769231,-0.415384615384615,-0.4,-0.384615384615385,-0.369230769230769,
-0.353846153846154,-0.338461538461538,-0.323076923076923,-0.307692307692308,
-0.292307692307692,-0.276923076923077,-0.261538461538462,-0.246153846153846,
-0.230769230769231,-0.215384615384615,-0.2,-0.184615384615385,-0.169230769230769,
-0.153846153846154,-0.138461538461538,-0.123076923076923,-0.107692307692308,
-0.0923076923076923,-0.0769230769230769,-0.0615384615384615,-0.0461538461538462,
-0.0307692307692308,-0.0153846153846154,0.),.UNSPECIFIED.)
CURVE()
GEOMETRIC_REPRESENTATION_ITEM()
RATIONAL_B_SPLINE_CURVE((1.,1.,1.,1.,1.,1.,1.,1.,1.,1.,1.,1.,1.,1.,1.,1.,
1.,1.,1.,1.,1.,1.,1.,1.,1.,1.,1.,1.,1.,1.,1.,1.,1.,1.,1.,1.,1.,1.,1.,1.,
1.,1.,1.,1.,1.,1.,1.,1.,1.,1.,1.,1.,1.,1.,1.,1.,1.,1.,1.,1.,1.,1.,1.,1.,
1.,1.,1.,1.,1.,1.))
REPRESENTATION_ITEM('')
);
#182=(
BOUNDED_CURVE()
B_SPLINE_CURVE(5,(#23660,#23661,#23662,#23663,#23664,#23665,#23666,#23667,
#23668,#23669,#23670,#23671,#23672,#23673,#23674,#23675,#23676,#23677,#23678,
#23679,#23680,#23681,#23682,#23683,#23684,#23685,#23686,#23687,#23688,#23689,
#23690,#23691,#23692,#23693,#23694,#23695,#23696,#23697,#23698,#23699,#23700,
#23701,#23702,#23703,#23704,#23705,#23706,#23707,#23708,#23709,#23710,#23711,
#23712,#23713,#23714,#23715,#23716,#23717,#23718,#23719,#23720,#23721,#23722,
#23723,#23724,#23725,#23726,#23727,#23728,#23729),.UNSPECIFIED.,.F.,.F.)
B_SPLINE_CURVE_WITH_KNOTS((6,1,1,1,1,1,1,1,1,1,1,1,1,1,1,1,1,1,1,1,1,1,
1,1,1,1,1,1,1,1,1,1,1,1,1,1,1,1,1,1,1,1,1,1,1,1,1,1,1,1,1,1,1,1,1,1,1,1,
1,1,1,1,1,1,1,6),(-1.,-0.984615384615383,-0.969230769230768,-0.953846153846152,
-0.938461538461537,-0.923076923076922,-0.907692307692306,-0.892307692307691,
-0.876923076923076,-0.86153846153846,-0.846153846153845,-0.83076923076923,
-0.815384615384614,-0.799999999999999,-0.784615384615384,-0.769230769230768,
-0.753846153846153,-0.738461538461538,-0.723076923076922,-0.707692307692307,
-0.692307692307692,-0.676923076923076,-0.661538461538461,-0.646153846153846,
-0.63076923076923,-0.615384615384615,-0.6,-0.584615384615384,-0.569230769230769,
-0.553846153846154,-0.538461538461538,-0.523076923076923,-0.507692307692308,
-0.492307692307692,-0.476923076923077,-0.461538461538462,-0.446153846153846,
-0.430769230769231,-0.415384615384615,-0.4,-0.384615384615385,-0.369230769230769,
-0.353846153846154,-0.338461538461538,-0.323076923076923,-0.307692307692308,
-0.292307692307692,-0.276923076923077,-0.261538461538462,-0.246153846153846,
-0.230769230769231,-0.215384615384615,-0.2,-0.184615384615385,-0.169230769230769,
-0.153846153846154,-0.138461538461538,-0.123076923076923,-0.107692307692308,
-0.0923076923076923,-0.0769230769230769,-0.0615384615384615,-0.0461538461538462,
-0.0307692307692308,-0.0153846153846154,0.),.UNSPECIFIED.)
CURVE()
GEOMETRIC_REPRESENTATION_ITEM()
RATIONAL_B_SPLINE_CURVE((1.,1.,1.,1.,1.,1.,1.,1.,1.,1.,1.,1.,1.,1.,1.,1.,
1.,1.,1.,1.,1.,1.,1.,1.,1.,1.,1.,1.,1.,1.,1.,1.,1.,1.,1.,1.,1.,1.,1.,1.,
1.,1.,1.,1.,1.,1.,1.,1.,1.,1.,1.,1.,1.,1.,1.,1.,1.,1.,1.,1.,1.,1.,1.,1.,
1.,1.,1.,1.,1.,1.))
REPRESENTATION_ITEM('')
);
#183=(
BOUNDED_CURVE()
B_SPLINE_CURVE(5,(#23876,#23877,#23878,#23879,#23880,#23881,#23882,#23883,
#23884,#23885,#23886,#23887,#23888,#23889,#23890,#23891,#23892,#23893,#23894,
#23895,#23896,#23897,#23898,#23899,#23900,#23901,#23902,#23903,#23904,#23905,
#23906,#23907,#23908,#23909,#23910,#23911,#23912,#23913,#23914,#23915,#23916,
#23917,#23918,#23919,#23920,#23921,#23922,#23923,#23924,#23925,#23926,#23927,
#23928,#23929,#23930,#23931,#23932,#23933,#23934,#23935,#23936,#23937,#23938,
#23939,#23940,#23941,#23942,#23943,#23944,#23945),.UNSPECIFIED.,.F.,.F.)
B_SPLINE_CURVE_WITH_KNOTS((6,1,1,1,1,1,1,1,1,1,1,1,1,1,1,1,1,1,1,1,1,1,
1,1,1,1,1,1,1,1,1,1,1,1,1,1,1,1,1,1,1,1,1,1,1,1,1,1,1,1,1,1,1,1,1,1,1,1,
1,1,1,1,1,1,1,6),(-1.,-0.984615384615383,-0.969230769230768,-0.953846153846152,
-0.938461538461537,-0.923076923076922,-0.907692307692306,-0.892307692307691,
-0.876923076923076,-0.86153846153846,-0.846153846153845,-0.83076923076923,
-0.815384615384614,-0.799999999999999,-0.784615384615384,-0.769230769230768,
-0.753846153846153,-0.738461538461538,-0.723076923076922,-0.707692307692307,
-0.692307692307692,-0.676923076923076,-0.661538461538461,-0.646153846153846,
-0.63076923076923,-0.615384615384615,-0.6,-0.584615384615384,-0.569230769230769,
-0.553846153846154,-0.538461538461538,-0.523076923076923,-0.507692307692308,
-0.492307692307692,-0.476923076923077,-0.461538461538462,-0.446153846153846,
-0.430769230769231,-0.415384615384615,-0.4,-0.384615384615385,-0.369230769230769,
-0.353846153846154,-0.338461538461538,-0.323076923076923,-0.307692307692308,
-0.292307692307692,-0.276923076923077,-0.261538461538462,-0.246153846153846,
-0.230769230769231,-0.215384615384615,-0.2,-0.184615384615385,-0.169230769230769,
-0.153846153846154,-0.138461538461538,-0.123076923076923,-0.107692307692308,
-0.0923076923076923,-0.0769230769230769,-0.0615384615384615,-0.0461538461538462,
-0.0307692307692308,-0.0153846153846154,0.),.UNSPECIFIED.)
CURVE()
GEOMETRIC_REPRESENTATION_ITEM()
RATIONAL_B_SPLINE_CURVE((1.,1.,1.,1.,1.,1.,1.,1.,1.,1.,1.,1.,1.,1.,1.,1.,
1.,1.,1.,1.,1.,1.,1.,1.,1.,1.,1.,1.,1.,1.,1.,1.,1.,1.,1.,1.,1.,1.,1.,1.,
1.,1.,1.,1.,1.,1.,1.,1.,1.,1.,1.,1.,1.,1.,1.,1.,1.,1.,1.,1.,1.,1.,1.,1.,
1.,1.,1.,1.,1.,1.))
REPRESENTATION_ITEM('')
);
#184=(
BOUNDED_CURVE()
B_SPLINE_CURVE(5,(#24092,#24093,#24094,#24095,#24096,#24097,#24098,#24099,
#24100,#24101,#24102,#24103,#24104,#24105,#24106,#24107,#24108,#24109,#24110,
#24111,#24112,#24113,#24114,#24115,#24116,#24117,#24118,#24119,#24120,#24121,
#24122,#24123,#24124,#24125,#24126,#24127,#24128,#24129,#24130,#24131,#24132,
#24133,#24134,#24135,#24136,#24137,#24138,#24139,#24140,#24141,#24142,#24143,
#24144,#24145,#24146,#24147,#24148,#24149,#24150,#24151,#24152,#24153,#24154,
#24155,#24156,#24157,#24158,#24159,#24160,#24161),.UNSPECIFIED.,.F.,.F.)
B_SPLINE_CURVE_WITH_KNOTS((6,1,1,1,1,1,1,1,1,1,1,1,1,1,1,1,1,1,1,1,1,1,
1,1,1,1,1,1,1,1,1,1,1,1,1,1,1,1,1,1,1,1,1,1,1,1,1,1,1,1,1,1,1,1,1,1,1,1,
1,1,1,1,1,1,1,6),(-1.,-0.984615384615383,-0.969230769230768,-0.953846153846152,
-0.938461538461537,-0.923076923076922,-0.907692307692306,-0.892307692307691,
-0.876923076923076,-0.86153846153846,-0.846153846153845,-0.83076923076923,
-0.815384615384614,-0.799999999999999,-0.784615384615384,-0.769230769230768,
-0.753846153846153,-0.738461538461538,-0.723076923076922,-0.707692307692307,
-0.692307692307692,-0.676923076923076,-0.661538461538461,-0.646153846153846,
-0.63076923076923,-0.615384615384615,-0.6,-0.584615384615384,-0.569230769230769,
-0.553846153846154,-0.538461538461538,-0.523076923076923,-0.507692307692308,
-0.492307692307692,-0.476923076923077,-0.461538461538462,-0.446153846153846,
-0.430769230769231,-0.415384615384615,-0.4,-0.384615384615385,-0.369230769230769,
-0.353846153846154,-0.338461538461538,-0.323076923076923,-0.307692307692308,
-0.292307692307692,-0.276923076923077,-0.261538461538462,-0.246153846153846,
-0.230769230769231,-0.215384615384615,-0.2,-0.184615384615385,-0.169230769230769,
-0.153846153846154,-0.138461538461538,-0.123076923076923,-0.107692307692308,
-0.0923076923076923,-0.0769230769230769,-0.0615384615384615,-0.0461538461538462,
-0.0307692307692308,-0.0153846153846154,0.),.UNSPECIFIED.)
CURVE()
GEOMETRIC_REPRESENTATION_ITEM()
RATIONAL_B_SPLINE_CURVE((1.,1.,1.,1.,1.,1.,1.,1.,1.,1.,1.,1.,1.,1.,1.,1.,
1.,1.,1.,1.,1.,1.,1.,1.,1.,1.,1.,1.,1.,1.,1.,1.,1.,1.,1.,1.,1.,1.,1.,1.,
1.,1.,1.,1.,1.,1.,1.,1.,1.,1.,1.,1.,1.,1.,1.,1.,1.,1.,1.,1.,1.,1.,1.,1.,
1.,1.,1.,1.,1.,1.))
REPRESENTATION_ITEM('')
);
#185=(
BOUNDED_CURVE()
B_SPLINE_CURVE(5,(#24308,#24309,#24310,#24311,#24312,#24313,#24314,#24315,
#24316,#24317,#24318,#24319,#24320,#24321,#24322,#24323,#24324,#24325,#24326,
#24327,#24328,#24329,#24330,#24331,#24332,#24333,#24334,#24335,#24336,#24337,
#24338,#24339,#24340,#24341,#24342,#24343,#24344,#24345,#24346,#24347,#24348,
#24349,#24350,#24351,#24352,#24353,#24354,#24355,#24356,#24357,#24358,#24359,
#24360,#24361,#24362,#24363,#24364,#24365,#24366,#24367,#24368,#24369,#24370,
#24371,#24372,#24373,#24374,#24375,#24376,#24377),.UNSPECIFIED.,.F.,.F.)
B_SPLINE_CURVE_WITH_KNOTS((6,1,1,1,1,1,1,1,1,1,1,1,1,1,1,1,1,1,1,1,1,1,
1,1,1,1,1,1,1,1,1,1,1,1,1,1,1,1,1,1,1,1,1,1,1,1,1,1,1,1,1,1,1,1,1,1,1,1,
1,1,1,1,1,1,1,6),(-1.,-0.984615384615383,-0.969230769230768,-0.953846153846152,
-0.938461538461537,-0.923076923076922,-0.907692307692306,-0.892307692307691,
-0.876923076923076,-0.86153846153846,-0.846153846153845,-0.83076923076923,
-0.815384615384614,-0.799999999999999,-0.784615384615384,-0.769230769230768,
-0.753846153846153,-0.738461538461538,-0.723076923076922,-0.707692307692307,
-0.692307692307692,-0.676923076923076,-0.661538461538461,-0.646153846153846,
-0.63076923076923,-0.615384615384615,-0.6,-0.584615384615384,-0.569230769230769,
-0.553846153846154,-0.538461538461538,-0.523076923076923,-0.507692307692308,
-0.492307692307692,-0.476923076923077,-0.461538461538462,-0.446153846153846,
-0.430769230769231,-0.415384615384615,-0.4,-0.384615384615385,-0.369230769230769,
-0.353846153846154,-0.338461538461538,-0.323076923076923,-0.307692307692308,
-0.292307692307692,-0.276923076923077,-0.261538461538462,-0.246153846153846,
-0.230769230769231,-0.215384615384615,-0.2,-0.184615384615385,-0.169230769230769,
-0.153846153846154,-0.138461538461538,-0.123076923076923,-0.107692307692308,
-0.0923076923076923,-0.0769230769230769,-0.0615384615384615,-0.0461538461538462,
-0.0307692307692308,-0.0153846153846154,0.),.UNSPECIFIED.)
CURVE()
GEOMETRIC_REPRESENTATION_ITEM()
RATIONAL_B_SPLINE_CURVE((1.,1.,1.,1.,1.,1.,1.,1.,1.,1.,1.,1.,1.,1.,1.,1.,
1.,1.,1.,1.,1.,1.,1.,1.,1.,1.,1.,1.,1.,1.,1.,1.,1.,1.,1.,1.,1.,1.,1.,1.,
1.,1.,1.,1.,1.,1.,1.,1.,1.,1.,1.,1.,1.,1.,1.,1.,1.,1.,1.,1.,1.,1.,1.,1.,
1.,1.,1.,1.,1.,1.))
REPRESENTATION_ITEM('')
);
#186=(
BOUNDED_CURVE()
B_SPLINE_CURVE(5,(#24524,#24525,#24526,#24527,#24528,#24529,#24530,#24531,
#24532,#24533,#24534,#24535,#24536,#24537,#24538,#24539,#24540,#24541,#24542,
#24543,#24544,#24545,#24546,#24547,#24548,#24549,#24550,#24551,#24552,#24553,
#24554,#24555,#24556,#24557,#24558,#24559,#24560,#24561,#24562,#24563,#24564,
#24565,#24566,#24567,#24568,#24569,#24570,#24571,#24572,#24573,#24574,#24575,
#24576,#24577,#24578,#24579,#24580,#24581,#24582,#24583,#24584,#24585,#24586,
#24587,#24588,#24589,#24590,#24591,#24592,#24593),.UNSPECIFIED.,.F.,.F.)
B_SPLINE_CURVE_WITH_KNOTS((6,1,1,1,1,1,1,1,1,1,1,1,1,1,1,1,1,1,1,1,1,1,
1,1,1,1,1,1,1,1,1,1,1,1,1,1,1,1,1,1,1,1,1,1,1,1,1,1,1,1,1,1,1,1,1,1,1,1,
1,1,1,1,1,1,1,6),(-1.,-0.984615384615383,-0.969230769230768,-0.953846153846152,
-0.938461538461537,-0.923076923076922,-0.907692307692306,-0.892307692307691,
-0.876923076923076,-0.86153846153846,-0.846153846153845,-0.83076923076923,
-0.815384615384614,-0.799999999999999,-0.784615384615384,-0.769230769230768,
-0.753846153846153,-0.738461538461538,-0.723076923076922,-0.707692307692307,
-0.692307692307692,-0.676923076923076,-0.661538461538461,-0.646153846153846,
-0.63076923076923,-0.615384615384615,-0.6,-0.584615384615384,-0.569230769230769,
-0.553846153846154,-0.538461538461538,-0.523076923076923,-0.507692307692308,
-0.492307692307692,-0.476923076923077,-0.461538461538462,-0.446153846153846,
-0.430769230769231,-0.415384615384615,-0.4,-0.384615384615385,-0.369230769230769,
-0.353846153846154,-0.338461538461538,-0.323076923076923,-0.307692307692308,
-0.292307692307692,-0.276923076923077,-0.261538461538462,-0.246153846153846,
-0.230769230769231,-0.215384615384615,-0.2,-0.184615384615385,-0.169230769230769,
-0.153846153846154,-0.138461538461538,-0.123076923076923,-0.107692307692308,
-0.0923076923076923,-0.0769230769230769,-0.0615384615384615,-0.0461538461538462,
-0.0307692307692308,-0.0153846153846154,0.),.UNSPECIFIED.)
CURVE()
GEOMETRIC_REPRESENTATION_ITEM()
RATIONAL_B_SPLINE_CURVE((1.,1.,1.,1.,1.,1.,1.,1.,1.,1.,1.,1.,1.,1.,1.,1.,
1.,1.,1.,1.,1.,1.,1.,1.,1.,1.,1.,1.,1.,1.,1.,1.,1.,1.,1.,1.,1.,1.,1.,1.,
1.,1.,1.,1.,1.,1.,1.,1.,1.,1.,1.,1.,1.,1.,1.,1.,1.,1.,1.,1.,1.,1.,1.,1.,
1.,1.,1.,1.,1.,1.))
REPRESENTATION_ITEM('')
);
#187=(
BOUNDED_CURVE()
B_SPLINE_CURVE(5,(#24740,#24741,#24742,#24743,#24744,#24745,#24746,#24747,
#24748,#24749,#24750,#24751,#24752,#24753,#24754,#24755,#24756,#24757,#24758,
#24759,#24760,#24761,#24762,#24763,#24764,#24765,#24766,#24767,#24768,#24769,
#24770,#24771,#24772,#24773,#24774,#24775,#24776,#24777,#24778,#24779,#24780,
#24781,#24782,#24783,#24784,#24785,#24786,#24787,#24788,#24789,#24790,#24791,
#24792,#24793,#24794,#24795,#24796,#24797,#24798,#24799,#24800,#24801,#24802,
#24803,#24804,#24805,#24806,#24807,#24808,#24809),.UNSPECIFIED.,.F.,.F.)
B_SPLINE_CURVE_WITH_KNOTS((6,1,1,1,1,1,1,1,1,1,1,1,1,1,1,1,1,1,1,1,1,1,
1,1,1,1,1,1,1,1,1,1,1,1,1,1,1,1,1,1,1,1,1,1,1,1,1,1,1,1,1,1,1,1,1,1,1,1,
1,1,1,1,1,1,1,6),(-1.,-0.984615384615383,-0.969230769230768,-0.953846153846152,
-0.938461538461537,-0.923076923076922,-0.907692307692306,-0.892307692307691,
-0.876923076923076,-0.86153846153846,-0.846153846153845,-0.83076923076923,
-0.815384615384614,-0.799999999999999,-0.784615384615384,-0.769230769230768,
-0.753846153846153,-0.738461538461538,-0.723076923076922,-0.707692307692307,
-0.692307692307692,-0.676923076923076,-0.661538461538461,-0.646153846153846,
-0.63076923076923,-0.615384615384615,-0.6,-0.584615384615384,-0.569230769230769,
-0.553846153846154,-0.538461538461538,-0.523076923076923,-0.507692307692308,
-0.492307692307692,-0.476923076923077,-0.461538461538462,-0.446153846153846,
-0.430769230769231,-0.415384615384615,-0.4,-0.384615384615385,-0.369230769230769,
-0.353846153846154,-0.338461538461538,-0.323076923076923,-0.307692307692308,
-0.292307692307692,-0.276923076923077,-0.261538461538462,-0.246153846153846,
-0.230769230769231,-0.215384615384615,-0.2,-0.184615384615385,-0.169230769230769,
-0.153846153846154,-0.138461538461538,-0.123076923076923,-0.107692307692308,
-0.0923076923076923,-0.0769230769230769,-0.0615384615384615,-0.0461538461538462,
-0.0307692307692308,-0.0153846153846154,0.),.UNSPECIFIED.)
CURVE()
GEOMETRIC_REPRESENTATION_ITEM()
RATIONAL_B_SPLINE_CURVE((1.,1.,1.,1.,1.,1.,1.,1.,1.,1.,1.,1.,1.,1.,1.,1.,
1.,1.,1.,1.,1.,1.,1.,1.,1.,1.,1.,1.,1.,1.,1.,1.,1.,1.,1.,1.,1.,1.,1.,1.,
1.,1.,1.,1.,1.,1.,1.,1.,1.,1.,1.,1.,1.,1.,1.,1.,1.,1.,1.,1.,1.,1.,1.,1.,
1.,1.,1.,1.,1.,1.))
REPRESENTATION_ITEM('')
);
#188=(
BOUNDED_CURVE()
B_SPLINE_CURVE(5,(#24956,#24957,#24958,#24959,#24960,#24961,#24962,#24963,
#24964,#24965,#24966,#24967,#24968,#24969,#24970,#24971,#24972,#24973,#24974,
#24975,#24976,#24977,#24978,#24979,#24980,#24981,#24982,#24983,#24984,#24985,
#24986,#24987,#24988,#24989,#24990,#24991,#24992,#24993,#24994,#24995,#24996,
#24997,#24998,#24999,#25000,#25001,#25002,#25003,#25004,#25005,#25006,#25007,
#25008,#25009,#25010,#25011,#25012,#25013,#25014,#25015,#25016,#25017,#25018,
#25019,#25020,#25021,#25022,#25023,#25024,#25025),.UNSPECIFIED.,.F.,.F.)
B_SPLINE_CURVE_WITH_KNOTS((6,1,1,1,1,1,1,1,1,1,1,1,1,1,1,1,1,1,1,1,1,1,
1,1,1,1,1,1,1,1,1,1,1,1,1,1,1,1,1,1,1,1,1,1,1,1,1,1,1,1,1,1,1,1,1,1,1,1,
1,1,1,1,1,1,1,6),(-1.,-0.984615384615383,-0.969230769230768,-0.953846153846152,
-0.938461538461537,-0.923076923076922,-0.907692307692306,-0.892307692307691,
-0.876923076923076,-0.86153846153846,-0.846153846153845,-0.83076923076923,
-0.815384615384614,-0.799999999999999,-0.784615384615384,-0.769230769230768,
-0.753846153846153,-0.738461538461538,-0.723076923076922,-0.707692307692307,
-0.692307692307692,-0.676923076923076,-0.661538461538461,-0.646153846153846,
-0.63076923076923,-0.615384615384615,-0.6,-0.584615384615384,-0.569230769230769,
-0.553846153846154,-0.538461538461538,-0.523076923076923,-0.507692307692308,
-0.492307692307692,-0.476923076923077,-0.461538461538462,-0.446153846153846,
-0.430769230769231,-0.415384615384615,-0.4,-0.384615384615385,-0.369230769230769,
-0.353846153846154,-0.338461538461538,-0.323076923076923,-0.307692307692308,
-0.292307692307692,-0.276923076923077,-0.261538461538462,-0.246153846153846,
-0.230769230769231,-0.215384615384615,-0.2,-0.184615384615385,-0.169230769230769,
-0.153846153846154,-0.138461538461538,-0.123076923076923,-0.107692307692308,
-0.0923076923076923,-0.0769230769230769,-0.0615384615384615,-0.0461538461538462,
-0.0307692307692308,-0.0153846153846154,0.),.UNSPECIFIED.)
CURVE()
GEOMETRIC_REPRESENTATION_ITEM()
RATIONAL_B_SPLINE_CURVE((1.,1.,1.,1.,1.,1.,1.,1.,1.,1.,1.,1.,1.,1.,1.,1.,
1.,1.,1.,1.,1.,1.,1.,1.,1.,1.,1.,1.,1.,1.,1.,1.,1.,1.,1.,1.,1.,1.,1.,1.,
1.,1.,1.,1.,1.,1.,1.,1.,1.,1.,1.,1.,1.,1.,1.,1.,1.,1.,1.,1.,1.,1.,1.,1.,
1.,1.,1.,1.,1.,1.))
REPRESENTATION_ITEM('')
);
#189=(
BOUNDED_CURVE()
B_SPLINE_CURVE(5,(#25172,#25173,#25174,#25175,#25176,#25177,#25178,#25179,
#25180,#25181,#25182,#25183,#25184,#25185,#25186,#25187,#25188,#25189,#25190,
#25191,#25192,#25193,#25194,#25195,#25196,#25197,#25198,#25199,#25200,#25201,
#25202,#25203,#25204,#25205,#25206,#25207,#25208,#25209,#25210,#25211,#25212,
#25213,#25214,#25215,#25216,#25217,#25218,#25219,#25220,#25221,#25222,#25223,
#25224,#25225,#25226,#25227,#25228,#25229,#25230,#25231,#25232,#25233,#25234,
#25235,#25236,#25237,#25238,#25239,#25240,#25241),.UNSPECIFIED.,.F.,.F.)
B_SPLINE_CURVE_WITH_KNOTS((6,1,1,1,1,1,1,1,1,1,1,1,1,1,1,1,1,1,1,1,1,1,
1,1,1,1,1,1,1,1,1,1,1,1,1,1,1,1,1,1,1,1,1,1,1,1,1,1,1,1,1,1,1,1,1,1,1,1,
1,1,1,1,1,1,1,6),(-1.,-0.984615384615383,-0.969230769230768,-0.953846153846152,
-0.938461538461537,-0.923076923076922,-0.907692307692306,-0.892307692307691,
-0.876923076923076,-0.86153846153846,-0.846153846153845,-0.83076923076923,
-0.815384615384614,-0.799999999999999,-0.784615384615384,-0.769230769230768,
-0.753846153846153,-0.738461538461538,-0.723076923076922,-0.707692307692307,
-0.692307692307692,-0.676923076923076,-0.661538461538461,-0.646153846153846,
-0.63076923076923,-0.615384615384615,-0.6,-0.584615384615384,-0.569230769230769,
-0.553846153846154,-0.538461538461538,-0.523076923076923,-0.507692307692308,
-0.492307692307692,-0.476923076923077,-0.461538461538462,-0.446153846153846,
-0.430769230769231,-0.415384615384615,-0.4,-0.384615384615385,-0.369230769230769,
-0.353846153846154,-0.338461538461538,-0.323076923076923,-0.307692307692308,
-0.292307692307692,-0.276923076923077,-0.261538461538462,-0.246153846153846,
-0.230769230769231,-0.215384615384615,-0.2,-0.184615384615385,-0.169230769230769,
-0.153846153846154,-0.138461538461538,-0.123076923076923,-0.107692307692308,
-0.0923076923076923,-0.0769230769230769,-0.0615384615384615,-0.0461538461538462,
-0.0307692307692308,-0.0153846153846154,0.),.UNSPECIFIED.)
CURVE()
GEOMETRIC_REPRESENTATION_ITEM()
RATIONAL_B_SPLINE_CURVE((1.,1.,1.,1.,1.,1.,1.,1.,1.,1.,1.,1.,1.,1.,1.,1.,
1.,1.,1.,1.,1.,1.,1.,1.,1.,1.,1.,1.,1.,1.,1.,1.,1.,1.,1.,1.,1.,1.,1.,1.,
1.,1.,1.,1.,1.,1.,1.,1.,1.,1.,1.,1.,1.,1.,1.,1.,1.,1.,1.,1.,1.,1.,1.,1.,
1.,1.,1.,1.,1.,1.))
REPRESENTATION_ITEM('')
);
#190=(
BOUNDED_CURVE()
B_SPLINE_CURVE(5,(#25388,#25389,#25390,#25391,#25392,#25393,#25394,#25395,
#25396,#25397,#25398,#25399,#25400,#25401,#25402,#25403,#25404,#25405,#25406,
#25407,#25408,#25409,#25410,#25411,#25412,#25413,#25414,#25415,#25416,#25417,
#25418,#25419,#25420,#25421,#25422,#25423,#25424,#25425,#25426,#25427,#25428,
#25429,#25430,#25431,#25432,#25433,#25434,#25435,#25436,#25437,#25438,#25439,
#25440,#25441,#25442,#25443,#25444,#25445,#25446,#25447,#25448,#25449,#25450,
#25451,#25452,#25453,#25454,#25455,#25456,#25457),.UNSPECIFIED.,.F.,.F.)
B_SPLINE_CURVE_WITH_KNOTS((6,1,1,1,1,1,1,1,1,1,1,1,1,1,1,1,1,1,1,1,1,1,
1,1,1,1,1,1,1,1,1,1,1,1,1,1,1,1,1,1,1,1,1,1,1,1,1,1,1,1,1,1,1,1,1,1,1,1,
1,1,1,1,1,1,1,6),(-1.,-0.984615384615383,-0.969230769230768,-0.953846153846152,
-0.938461538461537,-0.923076923076922,-0.907692307692306,-0.892307692307691,
-0.876923076923076,-0.86153846153846,-0.846153846153845,-0.83076923076923,
-0.815384615384614,-0.799999999999999,-0.784615384615384,-0.769230769230768,
-0.753846153846153,-0.738461538461538,-0.723076923076922,-0.707692307692307,
-0.692307692307692,-0.676923076923076,-0.661538461538461,-0.646153846153846,
-0.63076923076923,-0.615384615384615,-0.6,-0.584615384615384,-0.569230769230769,
-0.553846153846154,-0.538461538461538,-0.523076923076923,-0.507692307692308,
-0.492307692307692,-0.476923076923077,-0.461538461538462,-0.446153846153846,
-0.430769230769231,-0.415384615384615,-0.4,-0.384615384615385,-0.369230769230769,
-0.353846153846154,-0.338461538461538,-0.323076923076923,-0.307692307692308,
-0.292307692307692,-0.276923076923077,-0.261538461538462,-0.246153846153846,
-0.230769230769231,-0.215384615384615,-0.2,-0.184615384615385,-0.169230769230769,
-0.153846153846154,-0.138461538461538,-0.123076923076923,-0.107692307692308,
-0.0923076923076923,-0.0769230769230769,-0.0615384615384615,-0.0461538461538462,
-0.0307692307692308,-0.0153846153846154,0.),.UNSPECIFIED.)
CURVE()
GEOMETRIC_REPRESENTATION_ITEM()
RATIONAL_B_SPLINE_CURVE((1.,1.,1.,1.,1.,1.,1.,1.,1.,1.,1.,1.,1.,1.,1.,1.,
1.,1.,1.,1.,1.,1.,1.,1.,1.,1.,1.,1.,1.,1.,1.,1.,1.,1.,1.,1.,1.,1.,1.,1.,
1.,1.,1.,1.,1.,1.,1.,1.,1.,1.,1.,1.,1.,1.,1.,1.,1.,1.,1.,1.,1.,1.,1.,1.,
1.,1.,1.,1.,1.,1.))
REPRESENTATION_ITEM('')
);
#191=(
BOUNDED_CURVE()
B_SPLINE_CURVE(5,(#25604,#25605,#25606,#25607,#25608,#25609,#25610,#25611,
#25612,#25613,#25614,#25615,#25616,#25617,#25618,#25619,#25620,#25621,#25622,
#25623,#25624,#25625,#25626,#25627,#25628,#25629,#25630,#25631,#25632,#25633,
#25634,#25635,#25636,#25637,#25638,#25639,#25640,#25641,#25642,#25643,#25644,
#25645,#25646,#25647,#25648,#25649,#25650,#25651,#25652,#25653,#25654,#25655,
#25656,#25657,#25658,#25659,#25660,#25661,#25662,#25663,#25664,#25665,#25666,
#25667,#25668,#25669,#25670,#25671,#25672,#25673),.UNSPECIFIED.,.F.,.F.)
B_SPLINE_CURVE_WITH_KNOTS((6,1,1,1,1,1,1,1,1,1,1,1,1,1,1,1,1,1,1,1,1,1,
1,1,1,1,1,1,1,1,1,1,1,1,1,1,1,1,1,1,1,1,1,1,1,1,1,1,1,1,1,1,1,1,1,1,1,1,
1,1,1,1,1,1,1,6),(-1.,-0.984615384615383,-0.969230769230768,-0.953846153846152,
-0.938461538461537,-0.923076923076922,-0.907692307692306,-0.892307692307691,
-0.876923076923076,-0.86153846153846,-0.846153846153845,-0.83076923076923,
-0.815384615384614,-0.799999999999999,-0.784615384615384,-0.769230769230768,
-0.753846153846153,-0.738461538461538,-0.723076923076922,-0.707692307692307,
-0.692307692307692,-0.676923076923076,-0.661538461538461,-0.646153846153846,
-0.63076923076923,-0.615384615384615,-0.6,-0.584615384615384,-0.569230769230769,
-0.553846153846154,-0.538461538461538,-0.523076923076923,-0.507692307692308,
-0.492307692307692,-0.476923076923077,-0.461538461538462,-0.446153846153846,
-0.430769230769231,-0.415384615384615,-0.4,-0.384615384615385,-0.369230769230769,
-0.353846153846154,-0.338461538461538,-0.323076923076923,-0.307692307692308,
-0.292307692307692,-0.276923076923077,-0.261538461538462,-0.246153846153846,
-0.230769230769231,-0.215384615384615,-0.2,-0.184615384615385,-0.169230769230769,
-0.153846153846154,-0.138461538461538,-0.123076923076923,-0.107692307692308,
-0.0923076923076923,-0.0769230769230769,-0.0615384615384615,-0.0461538461538462,
-0.0307692307692308,-0.0153846153846154,0.),.UNSPECIFIED.)
CURVE()
GEOMETRIC_REPRESENTATION_ITEM()
RATIONAL_B_SPLINE_CURVE((1.,1.,1.,1.,1.,1.,1.,1.,1.,1.,1.,1.,1.,1.,1.,1.,
1.,1.,1.,1.,1.,1.,1.,1.,1.,1.,1.,1.,1.,1.,1.,1.,1.,1.,1.,1.,1.,1.,1.,1.,
1.,1.,1.,1.,1.,1.,1.,1.,1.,1.,1.,1.,1.,1.,1.,1.,1.,1.,1.,1.,1.,1.,1.,1.,
1.,1.,1.,1.,1.,1.))
REPRESENTATION_ITEM('')
);
#192=(
BOUNDED_CURVE()
B_SPLINE_CURVE(5,(#25820,#25821,#25822,#25823,#25824,#25825,#25826,#25827,
#25828,#25829,#25830,#25831,#25832,#25833,#25834,#25835,#25836,#25837,#25838,
#25839,#25840,#25841,#25842,#25843,#25844,#25845,#25846,#25847,#25848,#25849,
#25850,#25851,#25852,#25853,#25854,#25855,#25856,#25857,#25858,#25859,#25860,
#25861,#25862,#25863,#25864,#25865,#25866,#25867,#25868,#25869,#25870,#25871,
#25872,#25873,#25874,#25875,#25876,#25877,#25878,#25879,#25880,#25881,#25882,
#25883,#25884,#25885,#25886,#25887,#25888,#25889),.UNSPECIFIED.,.F.,.F.)
B_SPLINE_CURVE_WITH_KNOTS((6,1,1,1,1,1,1,1,1,1,1,1,1,1,1,1,1,1,1,1,1,1,
1,1,1,1,1,1,1,1,1,1,1,1,1,1,1,1,1,1,1,1,1,1,1,1,1,1,1,1,1,1,1,1,1,1,1,1,
1,1,1,1,1,1,1,6),(-1.,-0.984615384615383,-0.969230769230768,-0.953846153846152,
-0.938461538461537,-0.923076923076922,-0.907692307692306,-0.892307692307691,
-0.876923076923076,-0.86153846153846,-0.846153846153845,-0.83076923076923,
-0.815384615384614,-0.799999999999999,-0.784615384615384,-0.769230769230768,
-0.753846153846153,-0.738461538461538,-0.723076923076922,-0.707692307692307,
-0.692307692307692,-0.676923076923076,-0.661538461538461,-0.646153846153846,
-0.63076923076923,-0.615384615384615,-0.6,-0.584615384615384,-0.569230769230769,
-0.553846153846154,-0.538461538461538,-0.523076923076923,-0.507692307692308,
-0.492307692307692,-0.476923076923077,-0.461538461538462,-0.446153846153846,
-0.430769230769231,-0.415384615384615,-0.4,-0.384615384615385,-0.369230769230769,
-0.353846153846154,-0.338461538461538,-0.323076923076923,-0.307692307692308,
-0.292307692307692,-0.276923076923077,-0.261538461538462,-0.246153846153846,
-0.230769230769231,-0.215384615384615,-0.2,-0.184615384615385,-0.169230769230769,
-0.153846153846154,-0.138461538461538,-0.123076923076923,-0.107692307692308,
-0.0923076923076923,-0.0769230769230769,-0.0615384615384615,-0.0461538461538462,
-0.0307692307692308,-0.0153846153846154,0.),.UNSPECIFIED.)
CURVE()
GEOMETRIC_REPRESENTATION_ITEM()
RATIONAL_B_SPLINE_CURVE((1.,1.,1.,1.,1.,1.,1.,1.,1.,1.,1.,1.,1.,1.,1.,1.,
1.,1.,1.,1.,1.,1.,1.,1.,1.,1.,1.,1.,1.,1.,1.,1.,1.,1.,1.,1.,1.,1.,1.,1.,
1.,1.,1.,1.,1.,1.,1.,1.,1.,1.,1.,1.,1.,1.,1.,1.,1.,1.,1.,1.,1.,1.,1.,1.,
1.,1.,1.,1.,1.,1.))
REPRESENTATION_ITEM('')
);
#193=(
BOUNDED_CURVE()
B_SPLINE_CURVE(5,(#26036,#26037,#26038,#26039,#26040,#26041,#26042,#26043,
#26044,#26045,#26046,#26047,#26048,#26049,#26050,#26051,#26052,#26053,#26054,
#26055,#26056,#26057,#26058,#26059,#26060,#26061,#26062,#26063,#26064,#26065,
#26066,#26067,#26068,#26069,#26070,#26071,#26072,#26073,#26074,#26075,#26076,
#26077,#26078,#26079,#26080,#26081,#26082,#26083,#26084,#26085,#26086,#26087,
#26088,#26089,#26090,#26091,#26092,#26093,#26094,#26095,#26096,#26097,#26098,
#26099,#26100,#26101,#26102,#26103,#26104,#26105),.UNSPECIFIED.,.F.,.F.)
B_SPLINE_CURVE_WITH_KNOTS((6,1,1,1,1,1,1,1,1,1,1,1,1,1,1,1,1,1,1,1,1,1,
1,1,1,1,1,1,1,1,1,1,1,1,1,1,1,1,1,1,1,1,1,1,1,1,1,1,1,1,1,1,1,1,1,1,1,1,
1,1,1,1,1,1,1,6),(-1.,-0.984615384615383,-0.969230769230768,-0.953846153846152,
-0.938461538461537,-0.923076923076922,-0.907692307692306,-0.892307692307691,
-0.876923076923076,-0.86153846153846,-0.846153846153845,-0.83076923076923,
-0.815384615384614,-0.799999999999999,-0.784615384615384,-0.769230769230768,
-0.753846153846153,-0.738461538461538,-0.723076923076922,-0.707692307692307,
-0.692307692307692,-0.676923076923076,-0.661538461538461,-0.646153846153846,
-0.63076923076923,-0.615384615384615,-0.6,-0.584615384615384,-0.569230769230769,
-0.553846153846154,-0.538461538461538,-0.523076923076923,-0.507692307692308,
-0.492307692307692,-0.476923076923077,-0.461538461538462,-0.446153846153846,
-0.430769230769231,-0.415384615384615,-0.4,-0.384615384615385,-0.369230769230769,
-0.353846153846154,-0.338461538461538,-0.323076923076923,-0.307692307692308,
-0.292307692307692,-0.276923076923077,-0.261538461538462,-0.246153846153846,
-0.230769230769231,-0.215384615384615,-0.2,-0.184615384615385,-0.169230769230769,
-0.153846153846154,-0.138461538461538,-0.123076923076923,-0.107692307692308,
-0.0923076923076923,-0.0769230769230769,-0.0615384615384615,-0.0461538461538462,
-0.0307692307692308,-0.0153846153846154,0.),.UNSPECIFIED.)
CURVE()
GEOMETRIC_REPRESENTATION_ITEM()
RATIONAL_B_SPLINE_CURVE((1.,1.,1.,1.,1.,1.,1.,1.,1.,1.,1.,1.,1.,1.,1.,1.,
1.,1.,1.,1.,1.,1.,1.,1.,1.,1.,1.,1.,1.,1.,1.,1.,1.,1.,1.,1.,1.,1.,1.,1.,
1.,1.,1.,1.,1.,1.,1.,1.,1.,1.,1.,1.,1.,1.,1.,1.,1.,1.,1.,1.,1.,1.,1.,1.,
1.,1.,1.,1.,1.,1.))
REPRESENTATION_ITEM('')
);
#194=(
BOUNDED_CURVE()
B_SPLINE_CURVE(5,(#26252,#26253,#26254,#26255,#26256,#26257,#26258,#26259,
#26260,#26261,#26262,#26263,#26264,#26265,#26266,#26267,#26268,#26269,#26270,
#26271,#26272,#26273,#26274,#26275,#26276,#26277,#26278,#26279,#26280,#26281,
#26282,#26283,#26284,#26285,#26286,#26287,#26288,#26289,#26290,#26291,#26292,
#26293,#26294,#26295,#26296,#26297,#26298,#26299,#26300,#26301,#26302,#26303,
#26304,#26305,#26306,#26307,#26308,#26309,#26310,#26311,#26312,#26313,#26314,
#26315,#26316,#26317,#26318,#26319,#26320,#26321),.UNSPECIFIED.,.F.,.F.)
B_SPLINE_CURVE_WITH_KNOTS((6,1,1,1,1,1,1,1,1,1,1,1,1,1,1,1,1,1,1,1,1,1,
1,1,1,1,1,1,1,1,1,1,1,1,1,1,1,1,1,1,1,1,1,1,1,1,1,1,1,1,1,1,1,1,1,1,1,1,
1,1,1,1,1,1,1,6),(-1.,-0.984615384615383,-0.969230769230768,-0.953846153846152,
-0.938461538461537,-0.923076923076922,-0.907692307692306,-0.892307692307691,
-0.876923076923076,-0.86153846153846,-0.846153846153845,-0.83076923076923,
-0.815384615384614,-0.799999999999999,-0.784615384615384,-0.769230769230768,
-0.753846153846153,-0.738461538461538,-0.723076923076922,-0.707692307692307,
-0.692307692307692,-0.676923076923076,-0.661538461538461,-0.646153846153846,
-0.63076923076923,-0.615384615384615,-0.6,-0.584615384615384,-0.569230769230769,
-0.553846153846154,-0.538461538461538,-0.523076923076923,-0.507692307692308,
-0.492307692307692,-0.476923076923077,-0.461538461538462,-0.446153846153846,
-0.430769230769231,-0.415384615384615,-0.4,-0.384615384615385,-0.369230769230769,
-0.353846153846154,-0.338461538461538,-0.323076923076923,-0.307692307692308,
-0.292307692307692,-0.276923076923077,-0.261538461538462,-0.246153846153846,
-0.230769230769231,-0.215384615384615,-0.2,-0.184615384615385,-0.169230769230769,
-0.153846153846154,-0.138461538461538,-0.123076923076923,-0.107692307692308,
-0.0923076923076923,-0.0769230769230769,-0.0615384615384615,-0.0461538461538462,
-0.0307692307692308,-0.0153846153846154,0.),.UNSPECIFIED.)
CURVE()
GEOMETRIC_REPRESENTATION_ITEM()
RATIONAL_B_SPLINE_CURVE((1.,1.,1.,1.,1.,1.,1.,1.,1.,1.,1.,1.,1.,1.,1.,1.,
1.,1.,1.,1.,1.,1.,1.,1.,1.,1.,1.,1.,1.,1.,1.,1.,1.,1.,1.,1.,1.,1.,1.,1.,
1.,1.,1.,1.,1.,1.,1.,1.,1.,1.,1.,1.,1.,1.,1.,1.,1.,1.,1.,1.,1.,1.,1.,1.,
1.,1.,1.,1.,1.,1.))
REPRESENTATION_ITEM('')
);
#195=(
BOUNDED_CURVE()
B_SPLINE_CURVE(5,(#26468,#26469,#26470,#26471,#26472,#26473,#26474,#26475,
#26476,#26477,#26478,#26479,#26480,#26481,#26482,#26483,#26484,#26485,#26486,
#26487,#26488,#26489,#26490,#26491,#26492,#26493,#26494,#26495,#26496,#26497,
#26498,#26499,#26500,#26501,#26502,#26503,#26504,#26505,#26506,#26507,#26508,
#26509,#26510,#26511,#26512,#26513,#26514,#26515,#26516,#26517,#26518,#26519,
#26520,#26521,#26522,#26523,#26524,#26525,#26526,#26527,#26528,#26529,#26530,
#26531,#26532,#26533,#26534,#26535,#26536,#26537),.UNSPECIFIED.,.F.,.F.)
B_SPLINE_CURVE_WITH_KNOTS((6,1,1,1,1,1,1,1,1,1,1,1,1,1,1,1,1,1,1,1,1,1,
1,1,1,1,1,1,1,1,1,1,1,1,1,1,1,1,1,1,1,1,1,1,1,1,1,1,1,1,1,1,1,1,1,1,1,1,
1,1,1,1,1,1,1,6),(-1.,-0.984615384615383,-0.969230769230768,-0.953846153846152,
-0.938461538461537,-0.923076923076922,-0.907692307692306,-0.892307692307691,
-0.876923076923076,-0.86153846153846,-0.846153846153845,-0.83076923076923,
-0.815384615384614,-0.799999999999999,-0.784615384615384,-0.769230769230768,
-0.753846153846153,-0.738461538461538,-0.723076923076922,-0.707692307692307,
-0.692307692307692,-0.676923076923076,-0.661538461538461,-0.646153846153846,
-0.63076923076923,-0.615384615384615,-0.6,-0.584615384615384,-0.569230769230769,
-0.553846153846154,-0.538461538461538,-0.523076923076923,-0.507692307692308,
-0.492307692307692,-0.476923076923077,-0.461538461538462,-0.446153846153846,
-0.430769230769231,-0.415384615384615,-0.4,-0.384615384615385,-0.369230769230769,
-0.353846153846154,-0.338461538461538,-0.323076923076923,-0.307692307692308,
-0.292307692307692,-0.276923076923077,-0.261538461538462,-0.246153846153846,
-0.230769230769231,-0.215384615384615,-0.2,-0.184615384615385,-0.169230769230769,
-0.153846153846154,-0.138461538461538,-0.123076923076923,-0.107692307692308,
-0.0923076923076923,-0.0769230769230769,-0.0615384615384615,-0.0461538461538462,
-0.0307692307692308,-0.0153846153846154,0.),.UNSPECIFIED.)
CURVE()
GEOMETRIC_REPRESENTATION_ITEM()
RATIONAL_B_SPLINE_CURVE((1.,1.,1.,1.,1.,1.,1.,1.,1.,1.,1.,1.,1.,1.,1.,1.,
1.,1.,1.,1.,1.,1.,1.,1.,1.,1.,1.,1.,1.,1.,1.,1.,1.,1.,1.,1.,1.,1.,1.,1.,
1.,1.,1.,1.,1.,1.,1.,1.,1.,1.,1.,1.,1.,1.,1.,1.,1.,1.,1.,1.,1.,1.,1.,1.,
1.,1.,1.,1.,1.,1.))
REPRESENTATION_ITEM('')
);
#196=(
BOUNDED_CURVE()
B_SPLINE_CURVE(5,(#26684,#26685,#26686,#26687,#26688,#26689,#26690,#26691,
#26692,#26693,#26694,#26695,#26696,#26697,#26698,#26699,#26700,#26701,#26702,
#26703,#26704,#26705,#26706,#26707,#26708,#26709,#26710,#26711,#26712,#26713,
#26714,#26715,#26716,#26717,#26718,#26719,#26720,#26721,#26722,#26723,#26724,
#26725,#26726,#26727,#26728,#26729,#26730,#26731,#26732,#26733,#26734,#26735,
#26736,#26737,#26738,#26739,#26740,#26741,#26742,#26743,#26744,#26745,#26746,
#26747,#26748,#26749,#26750,#26751,#26752,#26753),.UNSPECIFIED.,.F.,.F.)
B_SPLINE_CURVE_WITH_KNOTS((6,1,1,1,1,1,1,1,1,1,1,1,1,1,1,1,1,1,1,1,1,1,
1,1,1,1,1,1,1,1,1,1,1,1,1,1,1,1,1,1,1,1,1,1,1,1,1,1,1,1,1,1,1,1,1,1,1,1,
1,1,1,1,1,1,1,6),(-1.,-0.984615384615383,-0.969230769230768,-0.953846153846152,
-0.938461538461537,-0.923076923076922,-0.907692307692306,-0.892307692307691,
-0.876923076923076,-0.86153846153846,-0.846153846153845,-0.83076923076923,
-0.815384615384614,-0.799999999999999,-0.784615384615384,-0.769230769230768,
-0.753846153846153,-0.738461538461538,-0.723076923076922,-0.707692307692307,
-0.692307692307692,-0.676923076923076,-0.661538461538461,-0.646153846153846,
-0.63076923076923,-0.615384615384615,-0.6,-0.584615384615384,-0.569230769230769,
-0.553846153846154,-0.538461538461538,-0.523076923076923,-0.507692307692308,
-0.492307692307692,-0.476923076923077,-0.461538461538462,-0.446153846153846,
-0.430769230769231,-0.415384615384615,-0.4,-0.384615384615385,-0.369230769230769,
-0.353846153846154,-0.338461538461538,-0.323076923076923,-0.307692307692308,
-0.292307692307692,-0.276923076923077,-0.261538461538462,-0.246153846153846,
-0.230769230769231,-0.215384615384615,-0.2,-0.184615384615385,-0.169230769230769,
-0.153846153846154,-0.138461538461538,-0.123076923076923,-0.107692307692308,
-0.0923076923076923,-0.0769230769230769,-0.0615384615384615,-0.0461538461538462,
-0.0307692307692308,-0.0153846153846154,0.),.UNSPECIFIED.)
CURVE()
GEOMETRIC_REPRESENTATION_ITEM()
RATIONAL_B_SPLINE_CURVE((1.,1.,1.,1.,1.,1.,1.,1.,1.,1.,1.,1.,1.,1.,1.,1.,
1.,1.,1.,1.,1.,1.,1.,1.,1.,1.,1.,1.,1.,1.,1.,1.,1.,1.,1.,1.,1.,1.,1.,1.,
1.,1.,1.,1.,1.,1.,1.,1.,1.,1.,1.,1.,1.,1.,1.,1.,1.,1.,1.,1.,1.,1.,1.,1.,
1.,1.,1.,1.,1.,1.))
REPRESENTATION_ITEM('')
);
#197=(
BOUNDED_CURVE()
B_SPLINE_CURVE(5,(#26900,#26901,#26902,#26903,#26904,#26905,#26906,#26907,
#26908,#26909,#26910,#26911,#26912,#26913,#26914,#26915,#26916,#26917,#26918,
#26919,#26920,#26921,#26922,#26923,#26924,#26925,#26926,#26927,#26928,#26929,
#26930,#26931,#26932,#26933,#26934,#26935,#26936,#26937,#26938,#26939,#26940,
#26941,#26942,#26943,#26944,#26945,#26946,#26947,#26948,#26949,#26950,#26951,
#26952,#26953,#26954,#26955,#26956,#26957,#26958,#26959,#26960,#26961,#26962,
#26963,#26964,#26965,#26966,#26967,#26968,#26969),.UNSPECIFIED.,.F.,.F.)
B_SPLINE_CURVE_WITH_KNOTS((6,1,1,1,1,1,1,1,1,1,1,1,1,1,1,1,1,1,1,1,1,1,
1,1,1,1,1,1,1,1,1,1,1,1,1,1,1,1,1,1,1,1,1,1,1,1,1,1,1,1,1,1,1,1,1,1,1,1,
1,1,1,1,1,1,1,6),(-1.,-0.984615384615383,-0.969230769230768,-0.953846153846152,
-0.938461538461537,-0.923076923076922,-0.907692307692306,-0.892307692307691,
-0.876923076923076,-0.86153846153846,-0.846153846153845,-0.83076923076923,
-0.815384615384614,-0.799999999999999,-0.784615384615384,-0.769230769230768,
-0.753846153846153,-0.738461538461538,-0.723076923076922,-0.707692307692307,
-0.692307692307692,-0.676923076923076,-0.661538461538461,-0.646153846153846,
-0.63076923076923,-0.615384615384615,-0.6,-0.584615384615384,-0.569230769230769,
-0.553846153846154,-0.538461538461538,-0.523076923076923,-0.507692307692308,
-0.492307692307692,-0.476923076923077,-0.461538461538462,-0.446153846153846,
-0.430769230769231,-0.415384615384615,-0.4,-0.384615384615385,-0.369230769230769,
-0.353846153846154,-0.338461538461538,-0.323076923076923,-0.307692307692308,
-0.292307692307692,-0.276923076923077,-0.261538461538462,-0.246153846153846,
-0.230769230769231,-0.215384615384615,-0.2,-0.184615384615385,-0.169230769230769,
-0.153846153846154,-0.138461538461538,-0.123076923076923,-0.107692307692308,
-0.0923076923076923,-0.0769230769230769,-0.0615384615384615,-0.0461538461538462,
-0.0307692307692308,-0.0153846153846154,0.),.UNSPECIFIED.)
CURVE()
GEOMETRIC_REPRESENTATION_ITEM()
RATIONAL_B_SPLINE_CURVE((1.,1.,1.,1.,1.,1.,1.,1.,1.,1.,1.,1.,1.,1.,1.,1.,
1.,1.,1.,1.,1.,1.,1.,1.,1.,1.,1.,1.,1.,1.,1.,1.,1.,1.,1.,1.,1.,1.,1.,1.,
1.,1.,1.,1.,1.,1.,1.,1.,1.,1.,1.,1.,1.,1.,1.,1.,1.,1.,1.,1.,1.,1.,1.,1.,
1.,1.,1.,1.,1.,1.))
REPRESENTATION_ITEM('')
);
#198=(
BOUNDED_CURVE()
B_SPLINE_CURVE(5,(#27116,#27117,#27118,#27119,#27120,#27121,#27122,#27123,
#27124,#27125,#27126,#27127,#27128,#27129,#27130,#27131,#27132,#27133,#27134,
#27135,#27136,#27137,#27138,#27139,#27140,#27141,#27142,#27143,#27144,#27145,
#27146,#27147,#27148,#27149,#27150,#27151,#27152,#27153,#27154,#27155,#27156,
#27157,#27158,#27159,#27160,#27161,#27162,#27163,#27164,#27165,#27166,#27167,
#27168,#27169,#27170,#27171,#27172,#27173,#27174,#27175,#27176,#27177,#27178,
#27179,#27180,#27181,#27182,#27183,#27184,#27185),.UNSPECIFIED.,.F.,.F.)
B_SPLINE_CURVE_WITH_KNOTS((6,1,1,1,1,1,1,1,1,1,1,1,1,1,1,1,1,1,1,1,1,1,
1,1,1,1,1,1,1,1,1,1,1,1,1,1,1,1,1,1,1,1,1,1,1,1,1,1,1,1,1,1,1,1,1,1,1,1,
1,1,1,1,1,1,1,6),(-1.,-0.984615384615383,-0.969230769230768,-0.953846153846152,
-0.938461538461537,-0.923076923076922,-0.907692307692306,-0.892307692307691,
-0.876923076923076,-0.86153846153846,-0.846153846153845,-0.83076923076923,
-0.815384615384614,-0.799999999999999,-0.784615384615384,-0.769230769230768,
-0.753846153846153,-0.738461538461538,-0.723076923076922,-0.707692307692307,
-0.692307692307692,-0.676923076923076,-0.661538461538461,-0.646153846153846,
-0.63076923076923,-0.615384615384615,-0.6,-0.584615384615384,-0.569230769230769,
-0.553846153846154,-0.538461538461538,-0.523076923076923,-0.507692307692308,
-0.492307692307692,-0.476923076923077,-0.461538461538462,-0.446153846153846,
-0.430769230769231,-0.415384615384615,-0.4,-0.384615384615385,-0.369230769230769,
-0.353846153846154,-0.338461538461538,-0.323076923076923,-0.307692307692308,
-0.292307692307692,-0.276923076923077,-0.261538461538462,-0.246153846153846,
-0.230769230769231,-0.215384615384615,-0.2,-0.184615384615385,-0.169230769230769,
-0.153846153846154,-0.138461538461538,-0.123076923076923,-0.107692307692308,
-0.0923076923076923,-0.0769230769230769,-0.0615384615384615,-0.0461538461538462,
-0.0307692307692308,-0.0153846153846154,0.),.UNSPECIFIED.)
CURVE()
GEOMETRIC_REPRESENTATION_ITEM()
RATIONAL_B_SPLINE_CURVE((1.,1.,1.,1.,1.,1.,1.,1.,1.,1.,1.,1.,1.,1.,1.,1.,
1.,1.,1.,1.,1.,1.,1.,1.,1.,1.,1.,1.,1.,1.,1.,1.,1.,1.,1.,1.,1.,1.,1.,1.,
1.,1.,1.,1.,1.,1.,1.,1.,1.,1.,1.,1.,1.,1.,1.,1.,1.,1.,1.,1.,1.,1.,1.,1.,
1.,1.,1.,1.,1.,1.))
REPRESENTATION_ITEM('')
);
#199=(
BOUNDED_CURVE()
B_SPLINE_CURVE(5,(#27332,#27333,#27334,#27335,#27336,#27337,#27338,#27339,
#27340,#27341,#27342,#27343,#27344,#27345,#27346,#27347,#27348,#27349,#27350,
#27351,#27352,#27353,#27354,#27355,#27356,#27357,#27358,#27359,#27360,#27361,
#27362,#27363,#27364,#27365,#27366,#27367,#27368,#27369,#27370,#27371,#27372,
#27373,#27374,#27375,#27376,#27377,#27378,#27379,#27380,#27381,#27382,#27383,
#27384,#27385,#27386,#27387,#27388,#27389,#27390,#27391,#27392,#27393,#27394,
#27395,#27396,#27397,#27398,#27399,#27400,#27401),.UNSPECIFIED.,.F.,.F.)
B_SPLINE_CURVE_WITH_KNOTS((6,1,1,1,1,1,1,1,1,1,1,1,1,1,1,1,1,1,1,1,1,1,
1,1,1,1,1,1,1,1,1,1,1,1,1,1,1,1,1,1,1,1,1,1,1,1,1,1,1,1,1,1,1,1,1,1,1,1,
1,1,1,1,1,1,1,6),(-1.,-0.984615384615383,-0.969230769230768,-0.953846153846152,
-0.938461538461537,-0.923076923076922,-0.907692307692306,-0.892307692307691,
-0.876923076923076,-0.86153846153846,-0.846153846153845,-0.83076923076923,
-0.815384615384614,-0.799999999999999,-0.784615384615384,-0.769230769230768,
-0.753846153846153,-0.738461538461538,-0.723076923076922,-0.707692307692307,
-0.692307692307692,-0.676923076923076,-0.661538461538461,-0.646153846153846,
-0.63076923076923,-0.615384615384615,-0.6,-0.584615384615384,-0.569230769230769,
-0.553846153846154,-0.538461538461538,-0.523076923076923,-0.507692307692308,
-0.492307692307692,-0.476923076923077,-0.461538461538462,-0.446153846153846,
-0.430769230769231,-0.415384615384615,-0.4,-0.384615384615385,-0.369230769230769,
-0.353846153846154,-0.338461538461538,-0.323076923076923,-0.307692307692308,
-0.292307692307692,-0.276923076923077,-0.261538461538462,-0.246153846153846,
-0.230769230769231,-0.215384615384615,-0.2,-0.184615384615385,-0.169230769230769,
-0.153846153846154,-0.138461538461538,-0.123076923076923,-0.107692307692308,
-0.0923076923076923,-0.0769230769230769,-0.0615384615384615,-0.0461538461538462,
-0.0307692307692308,-0.0153846153846154,0.),.UNSPECIFIED.)
CURVE()
GEOMETRIC_REPRESENTATION_ITEM()
RATIONAL_B_SPLINE_CURVE((1.,1.,1.,1.,1.,1.,1.,1.,1.,1.,1.,1.,1.,1.,1.,1.,
1.,1.,1.,1.,1.,1.,1.,1.,1.,1.,1.,1.,1.,1.,1.,1.,1.,1.,1.,1.,1.,1.,1.,1.,
1.,1.,1.,1.,1.,1.,1.,1.,1.,1.,1.,1.,1.,1.,1.,1.,1.,1.,1.,1.,1.,1.,1.,1.,
1.,1.,1.,1.,1.,1.))
REPRESENTATION_ITEM('')
);
#200=(
BOUNDED_CURVE()
B_SPLINE_CURVE(5,(#27548,#27549,#27550,#27551,#27552,#27553,#27554,#27555,
#27556,#27557,#27558,#27559,#27560,#27561,#27562,#27563,#27564,#27565,#27566,
#27567,#27568,#27569,#27570,#27571,#27572,#27573,#27574,#27575,#27576,#27577,
#27578,#27579,#27580,#27581,#27582,#27583,#27584,#27585,#27586,#27587,#27588,
#27589,#27590,#27591,#27592,#27593,#27594,#27595,#27596,#27597,#27598,#27599,
#27600,#27601,#27602,#27603,#27604,#27605,#27606,#27607,#27608,#27609,#27610,
#27611,#27612,#27613,#27614,#27615,#27616,#27617),.UNSPECIFIED.,.F.,.F.)
B_SPLINE_CURVE_WITH_KNOTS((6,1,1,1,1,1,1,1,1,1,1,1,1,1,1,1,1,1,1,1,1,1,
1,1,1,1,1,1,1,1,1,1,1,1,1,1,1,1,1,1,1,1,1,1,1,1,1,1,1,1,1,1,1,1,1,1,1,1,
1,1,1,1,1,1,1,6),(-1.,-0.984615384615383,-0.969230769230768,-0.953846153846152,
-0.938461538461537,-0.923076923076922,-0.907692307692306,-0.892307692307691,
-0.876923076923076,-0.86153846153846,-0.846153846153845,-0.83076923076923,
-0.815384615384614,-0.799999999999999,-0.784615384615384,-0.769230769230768,
-0.753846153846153,-0.738461538461538,-0.723076923076922,-0.707692307692307,
-0.692307692307692,-0.676923076923076,-0.661538461538461,-0.646153846153846,
-0.63076923076923,-0.615384615384615,-0.6,-0.584615384615384,-0.569230769230769,
-0.553846153846154,-0.538461538461538,-0.523076923076923,-0.507692307692308,
-0.492307692307692,-0.476923076923077,-0.461538461538462,-0.446153846153846,
-0.430769230769231,-0.415384615384615,-0.4,-0.384615384615385,-0.369230769230769,
-0.353846153846154,-0.338461538461538,-0.323076923076923,-0.307692307692308,
-0.292307692307692,-0.276923076923077,-0.261538461538462,-0.246153846153846,
-0.230769230769231,-0.215384615384615,-0.2,-0.184615384615385,-0.169230769230769,
-0.153846153846154,-0.138461538461538,-0.123076923076923,-0.107692307692308,
-0.0923076923076923,-0.0769230769230769,-0.0615384615384615,-0.0461538461538462,
-0.0307692307692308,-0.0153846153846154,0.),.UNSPECIFIED.)
CURVE()
GEOMETRIC_REPRESENTATION_ITEM()
RATIONAL_B_SPLINE_CURVE((1.,1.,1.,1.,1.,1.,1.,1.,1.,1.,1.,1.,1.,1.,1.,1.,
1.,1.,1.,1.,1.,1.,1.,1.,1.,1.,1.,1.,1.,1.,1.,1.,1.,1.,1.,1.,1.,1.,1.,1.,
1.,1.,1.,1.,1.,1.,1.,1.,1.,1.,1.,1.,1.,1.,1.,1.,1.,1.,1.,1.,1.,1.,1.,1.,
1.,1.,1.,1.,1.,1.))
REPRESENTATION_ITEM('')
);
#201=(
BOUNDED_CURVE()
B_SPLINE_CURVE(5,(#27764,#27765,#27766,#27767,#27768,#27769,#27770,#27771,
#27772,#27773,#27774,#27775,#27776,#27777,#27778,#27779,#27780,#27781,#27782,
#27783,#27784,#27785,#27786,#27787,#27788,#27789,#27790,#27791,#27792,#27793,
#27794,#27795,#27796,#27797,#27798,#27799,#27800,#27801,#27802,#27803,#27804,
#27805,#27806,#27807,#27808,#27809,#27810,#27811,#27812,#27813,#27814,#27815,
#27816,#27817,#27818,#27819,#27820,#27821,#27822,#27823,#27824,#27825,#27826,
#27827,#27828,#27829,#27830,#27831,#27832,#27833),.UNSPECIFIED.,.F.,.F.)
B_SPLINE_CURVE_WITH_KNOTS((6,1,1,1,1,1,1,1,1,1,1,1,1,1,1,1,1,1,1,1,1,1,
1,1,1,1,1,1,1,1,1,1,1,1,1,1,1,1,1,1,1,1,1,1,1,1,1,1,1,1,1,1,1,1,1,1,1,1,
1,1,1,1,1,1,1,6),(-1.,-0.984615384615383,-0.969230769230768,-0.953846153846152,
-0.938461538461537,-0.923076923076922,-0.907692307692306,-0.892307692307691,
-0.876923076923076,-0.86153846153846,-0.846153846153845,-0.83076923076923,
-0.815384615384614,-0.799999999999999,-0.784615384615384,-0.769230769230768,
-0.753846153846153,-0.738461538461538,-0.723076923076922,-0.707692307692307,
-0.692307692307692,-0.676923076923076,-0.661538461538461,-0.646153846153846,
-0.63076923076923,-0.615384615384615,-0.6,-0.584615384615384,-0.569230769230769,
-0.553846153846154,-0.538461538461538,-0.523076923076923,-0.507692307692308,
-0.492307692307692,-0.476923076923077,-0.461538461538462,-0.446153846153846,
-0.430769230769231,-0.415384615384615,-0.4,-0.384615384615385,-0.369230769230769,
-0.353846153846154,-0.338461538461538,-0.323076923076923,-0.307692307692308,
-0.292307692307692,-0.276923076923077,-0.261538461538462,-0.246153846153846,
-0.230769230769231,-0.215384615384615,-0.2,-0.184615384615385,-0.169230769230769,
-0.153846153846154,-0.138461538461538,-0.123076923076923,-0.107692307692308,
-0.0923076923076923,-0.0769230769230769,-0.0615384615384615,-0.0461538461538462,
-0.0307692307692308,-0.0153846153846154,0.),.UNSPECIFIED.)
CURVE()
GEOMETRIC_REPRESENTATION_ITEM()
RATIONAL_B_SPLINE_CURVE((1.,1.,1.,1.,1.,1.,1.,1.,1.,1.,1.,1.,1.,1.,1.,1.,
1.,1.,1.,1.,1.,1.,1.,1.,1.,1.,1.,1.,1.,1.,1.,1.,1.,1.,1.,1.,1.,1.,1.,1.,
1.,1.,1.,1.,1.,1.,1.,1.,1.,1.,1.,1.,1.,1.,1.,1.,1.,1.,1.,1.,1.,1.,1.,1.,
1.,1.,1.,1.,1.,1.))
REPRESENTATION_ITEM('')
);
#202=(
BOUNDED_CURVE()
B_SPLINE_CURVE(5,(#27980,#27981,#27982,#27983,#27984,#27985,#27986,#27987,
#27988,#27989,#27990,#27991,#27992,#27993,#27994,#27995,#27996,#27997,#27998,
#27999,#28000,#28001,#28002,#28003,#28004,#28005,#28006,#28007,#28008,#28009,
#28010,#28011,#28012,#28013,#28014,#28015,#28016,#28017,#28018,#28019,#28020,
#28021,#28022,#28023,#28024,#28025,#28026,#28027,#28028,#28029,#28030,#28031,
#28032,#28033,#28034,#28035,#28036,#28037,#28038,#28039,#28040,#28041,#28042,
#28043,#28044,#28045,#28046,#28047,#28048,#28049),.UNSPECIFIED.,.F.,.F.)
B_SPLINE_CURVE_WITH_KNOTS((6,1,1,1,1,1,1,1,1,1,1,1,1,1,1,1,1,1,1,1,1,1,
1,1,1,1,1,1,1,1,1,1,1,1,1,1,1,1,1,1,1,1,1,1,1,1,1,1,1,1,1,1,1,1,1,1,1,1,
1,1,1,1,1,1,1,6),(-1.,-0.984615384615383,-0.969230769230768,-0.953846153846152,
-0.938461538461537,-0.923076923076922,-0.907692307692306,-0.892307692307691,
-0.876923076923076,-0.86153846153846,-0.846153846153845,-0.83076923076923,
-0.815384615384614,-0.799999999999999,-0.784615384615384,-0.769230769230768,
-0.753846153846153,-0.738461538461538,-0.723076923076922,-0.707692307692307,
-0.692307692307692,-0.676923076923076,-0.661538461538461,-0.646153846153846,
-0.63076923076923,-0.615384615384615,-0.6,-0.584615384615384,-0.569230769230769,
-0.553846153846154,-0.538461538461538,-0.523076923076923,-0.507692307692308,
-0.492307692307692,-0.476923076923077,-0.461538461538462,-0.446153846153846,
-0.430769230769231,-0.415384615384615,-0.4,-0.384615384615385,-0.369230769230769,
-0.353846153846154,-0.338461538461538,-0.323076923076923,-0.307692307692308,
-0.292307692307692,-0.276923076923077,-0.261538461538462,-0.246153846153846,
-0.230769230769231,-0.215384615384615,-0.2,-0.184615384615385,-0.169230769230769,
-0.153846153846154,-0.138461538461538,-0.123076923076923,-0.107692307692308,
-0.0923076923076923,-0.0769230769230769,-0.0615384615384615,-0.0461538461538462,
-0.0307692307692308,-0.0153846153846154,0.),.UNSPECIFIED.)
CURVE()
GEOMETRIC_REPRESENTATION_ITEM()
RATIONAL_B_SPLINE_CURVE((1.,1.,1.,1.,1.,1.,1.,1.,1.,1.,1.,1.,1.,1.,1.,1.,
1.,1.,1.,1.,1.,1.,1.,1.,1.,1.,1.,1.,1.,1.,1.,1.,1.,1.,1.,1.,1.,1.,1.,1.,
1.,1.,1.,1.,1.,1.,1.,1.,1.,1.,1.,1.,1.,1.,1.,1.,1.,1.,1.,1.,1.,1.,1.,1.,
1.,1.,1.,1.,1.,1.))
REPRESENTATION_ITEM('')
);
#203=(
BOUNDED_CURVE()
B_SPLINE_CURVE(5,(#28196,#28197,#28198,#28199,#28200,#28201,#28202,#28203,
#28204,#28205,#28206,#28207,#28208,#28209,#28210,#28211,#28212,#28213,#28214,
#28215,#28216,#28217,#28218,#28219,#28220,#28221,#28222,#28223,#28224,#28225,
#28226,#28227,#28228,#28229,#28230,#28231,#28232,#28233,#28234,#28235,#28236,
#28237,#28238,#28239,#28240,#28241,#28242,#28243,#28244,#28245,#28246,#28247,
#28248,#28249,#28250,#28251,#28252,#28253,#28254,#28255,#28256,#28257,#28258,
#28259,#28260,#28261,#28262,#28263,#28264,#28265),.UNSPECIFIED.,.F.,.F.)
B_SPLINE_CURVE_WITH_KNOTS((6,1,1,1,1,1,1,1,1,1,1,1,1,1,1,1,1,1,1,1,1,1,
1,1,1,1,1,1,1,1,1,1,1,1,1,1,1,1,1,1,1,1,1,1,1,1,1,1,1,1,1,1,1,1,1,1,1,1,
1,1,1,1,1,1,1,6),(-1.,-0.984615384615383,-0.969230769230768,-0.953846153846152,
-0.938461538461537,-0.923076923076922,-0.907692307692306,-0.892307692307691,
-0.876923076923076,-0.86153846153846,-0.846153846153845,-0.83076923076923,
-0.815384615384614,-0.799999999999999,-0.784615384615384,-0.769230769230768,
-0.753846153846153,-0.738461538461538,-0.723076923076922,-0.707692307692307,
-0.692307692307692,-0.676923076923076,-0.661538461538461,-0.646153846153846,
-0.63076923076923,-0.615384615384615,-0.6,-0.584615384615384,-0.569230769230769,
-0.553846153846154,-0.538461538461538,-0.523076923076923,-0.507692307692308,
-0.492307692307692,-0.476923076923077,-0.461538461538462,-0.446153846153846,
-0.430769230769231,-0.415384615384615,-0.4,-0.384615384615385,-0.369230769230769,
-0.353846153846154,-0.338461538461538,-0.323076923076923,-0.307692307692308,
-0.292307692307692,-0.276923076923077,-0.261538461538462,-0.246153846153846,
-0.230769230769231,-0.215384615384615,-0.2,-0.184615384615385,-0.169230769230769,
-0.153846153846154,-0.138461538461538,-0.123076923076923,-0.107692307692308,
-0.0923076923076923,-0.0769230769230769,-0.0615384615384615,-0.0461538461538462,
-0.0307692307692308,-0.0153846153846154,0.),.UNSPECIFIED.)
CURVE()
GEOMETRIC_REPRESENTATION_ITEM()
RATIONAL_B_SPLINE_CURVE((1.,1.,1.,1.,1.,1.,1.,1.,1.,1.,1.,1.,1.,1.,1.,1.,
1.,1.,1.,1.,1.,1.,1.,1.,1.,1.,1.,1.,1.,1.,1.,1.,1.,1.,1.,1.,1.,1.,1.,1.,
1.,1.,1.,1.,1.,1.,1.,1.,1.,1.,1.,1.,1.,1.,1.,1.,1.,1.,1.,1.,1.,1.,1.,1.,
1.,1.,1.,1.,1.,1.))
REPRESENTATION_ITEM('')
);
#204=(
BOUNDED_CURVE()
B_SPLINE_CURVE(5,(#28412,#28413,#28414,#28415,#28416,#28417,#28418,#28419,
#28420,#28421,#28422,#28423,#28424,#28425,#28426,#28427,#28428,#28429,#28430,
#28431,#28432,#28433,#28434,#28435,#28436,#28437,#28438,#28439,#28440,#28441,
#28442,#28443,#28444,#28445,#28446,#28447,#28448,#28449,#28450,#28451,#28452,
#28453,#28454,#28455,#28456,#28457,#28458,#28459,#28460,#28461,#28462,#28463,
#28464,#28465,#28466,#28467,#28468,#28469,#28470,#28471,#28472,#28473,#28474,
#28475,#28476,#28477,#28478,#28479,#28480,#28481),.UNSPECIFIED.,.F.,.F.)
B_SPLINE_CURVE_WITH_KNOTS((6,1,1,1,1,1,1,1,1,1,1,1,1,1,1,1,1,1,1,1,1,1,
1,1,1,1,1,1,1,1,1,1,1,1,1,1,1,1,1,1,1,1,1,1,1,1,1,1,1,1,1,1,1,1,1,1,1,1,
1,1,1,1,1,1,1,6),(-1.,-0.984615384615383,-0.969230769230768,-0.953846153846152,
-0.938461538461537,-0.923076923076922,-0.907692307692306,-0.892307692307691,
-0.876923076923076,-0.86153846153846,-0.846153846153845,-0.83076923076923,
-0.815384615384614,-0.799999999999999,-0.784615384615384,-0.769230769230768,
-0.753846153846153,-0.738461538461538,-0.723076923076922,-0.707692307692307,
-0.692307692307692,-0.676923076923076,-0.661538461538461,-0.646153846153846,
-0.63076923076923,-0.615384615384615,-0.6,-0.584615384615384,-0.569230769230769,
-0.553846153846154,-0.538461538461538,-0.523076923076923,-0.507692307692308,
-0.492307692307692,-0.476923076923077,-0.461538461538462,-0.446153846153846,
-0.430769230769231,-0.415384615384615,-0.4,-0.384615384615385,-0.369230769230769,
-0.353846153846154,-0.338461538461538,-0.323076923076923,-0.307692307692308,
-0.292307692307692,-0.276923076923077,-0.261538461538462,-0.246153846153846,
-0.230769230769231,-0.215384615384615,-0.2,-0.184615384615385,-0.169230769230769,
-0.153846153846154,-0.138461538461538,-0.123076923076923,-0.107692307692308,
-0.0923076923076923,-0.0769230769230769,-0.0615384615384615,-0.0461538461538462,
-0.0307692307692308,-0.0153846153846154,0.),.UNSPECIFIED.)
CURVE()
GEOMETRIC_REPRESENTATION_ITEM()
RATIONAL_B_SPLINE_CURVE((1.,1.,1.,1.,1.,1.,1.,1.,1.,1.,1.,1.,1.,1.,1.,1.,
1.,1.,1.,1.,1.,1.,1.,1.,1.,1.,1.,1.,1.,1.,1.,1.,1.,1.,1.,1.,1.,1.,1.,1.,
1.,1.,1.,1.,1.,1.,1.,1.,1.,1.,1.,1.,1.,1.,1.,1.,1.,1.,1.,1.,1.,1.,1.,1.,
1.,1.,1.,1.,1.,1.))
REPRESENTATION_ITEM('')
);
#205=(
BOUNDED_CURVE()
B_SPLINE_CURVE(5,(#28628,#28629,#28630,#28631,#28632,#28633,#28634,#28635,
#28636,#28637,#28638,#28639,#28640,#28641,#28642,#28643,#28644,#28645,#28646,
#28647,#28648,#28649,#28650,#28651,#28652,#28653,#28654,#28655,#28656,#28657,
#28658,#28659,#28660,#28661,#28662,#28663,#28664,#28665,#28666,#28667,#28668,
#28669,#28670,#28671,#28672,#28673,#28674,#28675,#28676,#28677,#28678,#28679,
#28680,#28681,#28682,#28683,#28684,#28685,#28686,#28687,#28688,#28689,#28690,
#28691,#28692,#28693,#28694,#28695,#28696,#28697),.UNSPECIFIED.,.F.,.F.)
B_SPLINE_CURVE_WITH_KNOTS((6,1,1,1,1,1,1,1,1,1,1,1,1,1,1,1,1,1,1,1,1,1,
1,1,1,1,1,1,1,1,1,1,1,1,1,1,1,1,1,1,1,1,1,1,1,1,1,1,1,1,1,1,1,1,1,1,1,1,
1,1,1,1,1,1,1,6),(-1.,-0.984615384615383,-0.969230769230768,-0.953846153846152,
-0.938461538461537,-0.923076923076922,-0.907692307692306,-0.892307692307691,
-0.876923076923076,-0.86153846153846,-0.846153846153845,-0.83076923076923,
-0.815384615384614,-0.799999999999999,-0.784615384615384,-0.769230769230768,
-0.753846153846153,-0.738461538461538,-0.723076923076922,-0.707692307692307,
-0.692307692307692,-0.676923076923076,-0.661538461538461,-0.646153846153846,
-0.63076923076923,-0.615384615384615,-0.6,-0.584615384615384,-0.569230769230769,
-0.553846153846154,-0.538461538461538,-0.523076923076923,-0.507692307692308,
-0.492307692307692,-0.476923076923077,-0.461538461538462,-0.446153846153846,
-0.430769230769231,-0.415384615384615,-0.4,-0.384615384615385,-0.369230769230769,
-0.353846153846154,-0.338461538461538,-0.323076923076923,-0.307692307692308,
-0.292307692307692,-0.276923076923077,-0.261538461538462,-0.246153846153846,
-0.230769230769231,-0.215384615384615,-0.2,-0.184615384615385,-0.169230769230769,
-0.153846153846154,-0.138461538461538,-0.123076923076923,-0.107692307692308,
-0.0923076923076923,-0.0769230769230769,-0.0615384615384615,-0.0461538461538462,
-0.0307692307692308,-0.0153846153846154,0.),.UNSPECIFIED.)
CURVE()
GEOMETRIC_REPRESENTATION_ITEM()
RATIONAL_B_SPLINE_CURVE((1.,1.,1.,1.,1.,1.,1.,1.,1.,1.,1.,1.,1.,1.,1.,1.,
1.,1.,1.,1.,1.,1.,1.,1.,1.,1.,1.,1.,1.,1.,1.,1.,1.,1.,1.,1.,1.,1.,1.,1.,
1.,1.,1.,1.,1.,1.,1.,1.,1.,1.,1.,1.,1.,1.,1.,1.,1.,1.,1.,1.,1.,1.,1.,1.,
1.,1.,1.,1.,1.,1.))
REPRESENTATION_ITEM('')
);
#206=(
BOUNDED_CURVE()
B_SPLINE_CURVE(5,(#28844,#28845,#28846,#28847,#28848,#28849,#28850,#28851,
#28852,#28853,#28854,#28855,#28856,#28857,#28858,#28859,#28860,#28861,#28862,
#28863,#28864,#28865,#28866,#28867,#28868,#28869,#28870,#28871,#28872,#28873,
#28874,#28875,#28876,#28877,#28878,#28879,#28880,#28881,#28882,#28883,#28884,
#28885,#28886,#28887,#28888,#28889,#28890,#28891,#28892,#28893,#28894,#28895,
#28896,#28897,#28898,#28899,#28900,#28901,#28902,#28903,#28904,#28905,#28906,
#28907,#28908,#28909,#28910,#28911,#28912,#28913),.UNSPECIFIED.,.F.,.F.)
B_SPLINE_CURVE_WITH_KNOTS((6,1,1,1,1,1,1,1,1,1,1,1,1,1,1,1,1,1,1,1,1,1,
1,1,1,1,1,1,1,1,1,1,1,1,1,1,1,1,1,1,1,1,1,1,1,1,1,1,1,1,1,1,1,1,1,1,1,1,
1,1,1,1,1,1,1,6),(-1.,-0.984615384615383,-0.969230769230768,-0.953846153846152,
-0.938461538461537,-0.923076923076922,-0.907692307692306,-0.892307692307691,
-0.876923076923076,-0.86153846153846,-0.846153846153845,-0.83076923076923,
-0.815384615384614,-0.799999999999999,-0.784615384615384,-0.769230769230768,
-0.753846153846153,-0.738461538461538,-0.723076923076922,-0.707692307692307,
-0.692307692307692,-0.676923076923076,-0.661538461538461,-0.646153846153846,
-0.63076923076923,-0.615384615384615,-0.6,-0.584615384615384,-0.569230769230769,
-0.553846153846154,-0.538461538461538,-0.523076923076923,-0.507692307692308,
-0.492307692307692,-0.476923076923077,-0.461538461538462,-0.446153846153846,
-0.430769230769231,-0.415384615384615,-0.4,-0.384615384615385,-0.369230769230769,
-0.353846153846154,-0.338461538461538,-0.323076923076923,-0.307692307692308,
-0.292307692307692,-0.276923076923077,-0.261538461538462,-0.246153846153846,
-0.230769230769231,-0.215384615384615,-0.2,-0.184615384615385,-0.169230769230769,
-0.153846153846154,-0.138461538461538,-0.123076923076923,-0.107692307692308,
-0.0923076923076923,-0.0769230769230769,-0.0615384615384615,-0.0461538461538462,
-0.0307692307692308,-0.0153846153846154,0.),.UNSPECIFIED.)
CURVE()
GEOMETRIC_REPRESENTATION_ITEM()
RATIONAL_B_SPLINE_CURVE((1.,1.,1.,1.,1.,1.,1.,1.,1.,1.,1.,1.,1.,1.,1.,1.,
1.,1.,1.,1.,1.,1.,1.,1.,1.,1.,1.,1.,1.,1.,1.,1.,1.,1.,1.,1.,1.,1.,1.,1.,
1.,1.,1.,1.,1.,1.,1.,1.,1.,1.,1.,1.,1.,1.,1.,1.,1.,1.,1.,1.,1.,1.,1.,1.,
1.,1.,1.,1.,1.,1.))
REPRESENTATION_ITEM('')
);
#207=(
BOUNDED_CURVE()
B_SPLINE_CURVE(5,(#29060,#29061,#29062,#29063,#29064,#29065,#29066,#29067,
#29068,#29069,#29070,#29071,#29072,#29073,#29074,#29075,#29076,#29077,#29078,
#29079,#29080,#29081,#29082,#29083,#29084,#29085,#29086,#29087,#29088,#29089,
#29090,#29091,#29092,#29093,#29094,#29095,#29096,#29097,#29098,#29099,#29100,
#29101,#29102,#29103,#29104,#29105,#29106,#29107,#29108,#29109,#29110,#29111,
#29112,#29113,#29114,#29115,#29116,#29117,#29118,#29119,#29120,#29121,#29122,
#29123,#29124,#29125,#29126,#29127,#29128,#29129),.UNSPECIFIED.,.F.,.F.)
B_SPLINE_CURVE_WITH_KNOTS((6,1,1,1,1,1,1,1,1,1,1,1,1,1,1,1,1,1,1,1,1,1,
1,1,1,1,1,1,1,1,1,1,1,1,1,1,1,1,1,1,1,1,1,1,1,1,1,1,1,1,1,1,1,1,1,1,1,1,
1,1,1,1,1,1,1,6),(-1.,-0.984615384615383,-0.969230769230768,-0.953846153846152,
-0.938461538461537,-0.923076923076922,-0.907692307692306,-0.892307692307691,
-0.876923076923076,-0.86153846153846,-0.846153846153845,-0.83076923076923,
-0.815384615384614,-0.799999999999999,-0.784615384615384,-0.769230769230768,
-0.753846153846153,-0.738461538461538,-0.723076923076922,-0.707692307692307,
-0.692307692307692,-0.676923076923076,-0.661538461538461,-0.646153846153846,
-0.63076923076923,-0.615384615384615,-0.6,-0.584615384615384,-0.569230769230769,
-0.553846153846154,-0.538461538461538,-0.523076923076923,-0.507692307692308,
-0.492307692307692,-0.476923076923077,-0.461538461538462,-0.446153846153846,
-0.430769230769231,-0.415384615384615,-0.4,-0.384615384615385,-0.369230769230769,
-0.353846153846154,-0.338461538461538,-0.323076923076923,-0.307692307692308,
-0.292307692307692,-0.276923076923077,-0.261538461538462,-0.246153846153846,
-0.230769230769231,-0.215384615384615,-0.2,-0.184615384615385,-0.169230769230769,
-0.153846153846154,-0.138461538461538,-0.123076923076923,-0.107692307692308,
-0.0923076923076923,-0.0769230769230769,-0.0615384615384615,-0.0461538461538462,
-0.0307692307692308,-0.0153846153846154,0.),.UNSPECIFIED.)
CURVE()
GEOMETRIC_REPRESENTATION_ITEM()
RATIONAL_B_SPLINE_CURVE((1.,1.,1.,1.,1.,1.,1.,1.,1.,1.,1.,1.,1.,1.,1.,1.,
1.,1.,1.,1.,1.,1.,1.,1.,1.,1.,1.,1.,1.,1.,1.,1.,1.,1.,1.,1.,1.,1.,1.,1.,
1.,1.,1.,1.,1.,1.,1.,1.,1.,1.,1.,1.,1.,1.,1.,1.,1.,1.,1.,1.,1.,1.,1.,1.,
1.,1.,1.,1.,1.,1.))
REPRESENTATION_ITEM('')
);
#208=(
BOUNDED_CURVE()
B_SPLINE_CURVE(5,(#29276,#29277,#29278,#29279,#29280,#29281,#29282,#29283,
#29284,#29285,#29286,#29287,#29288,#29289,#29290,#29291,#29292,#29293,#29294,
#29295,#29296,#29297,#29298,#29299,#29300,#29301,#29302,#29303,#29304,#29305,
#29306,#29307,#29308,#29309,#29310,#29311,#29312,#29313,#29314,#29315,#29316,
#29317,#29318,#29319,#29320,#29321,#29322,#29323,#29324,#29325,#29326,#29327,
#29328,#29329,#29330,#29331,#29332,#29333,#29334,#29335,#29336,#29337,#29338,
#29339,#29340,#29341,#29342,#29343,#29344,#29345),.UNSPECIFIED.,.F.,.F.)
B_SPLINE_CURVE_WITH_KNOTS((6,1,1,1,1,1,1,1,1,1,1,1,1,1,1,1,1,1,1,1,1,1,
1,1,1,1,1,1,1,1,1,1,1,1,1,1,1,1,1,1,1,1,1,1,1,1,1,1,1,1,1,1,1,1,1,1,1,1,
1,1,1,1,1,1,1,6),(-1.,-0.984615384615383,-0.969230769230768,-0.953846153846152,
-0.938461538461537,-0.923076923076922,-0.907692307692306,-0.892307692307691,
-0.876923076923076,-0.86153846153846,-0.846153846153845,-0.83076923076923,
-0.815384615384614,-0.799999999999999,-0.784615384615384,-0.769230769230768,
-0.753846153846153,-0.738461538461538,-0.723076923076922,-0.707692307692307,
-0.692307692307692,-0.676923076923076,-0.661538461538461,-0.646153846153846,
-0.63076923076923,-0.615384615384615,-0.6,-0.584615384615384,-0.569230769230769,
-0.553846153846154,-0.538461538461538,-0.523076923076923,-0.507692307692308,
-0.492307692307692,-0.476923076923077,-0.461538461538462,-0.446153846153846,
-0.430769230769231,-0.415384615384615,-0.4,-0.384615384615385,-0.369230769230769,
-0.353846153846154,-0.338461538461538,-0.323076923076923,-0.307692307692308,
-0.292307692307692,-0.276923076923077,-0.261538461538462,-0.246153846153846,
-0.230769230769231,-0.215384615384615,-0.2,-0.184615384615385,-0.169230769230769,
-0.153846153846154,-0.138461538461538,-0.123076923076923,-0.107692307692308,
-0.0923076923076923,-0.0769230769230769,-0.0615384615384615,-0.0461538461538462,
-0.0307692307692308,-0.0153846153846154,0.),.UNSPECIFIED.)
CURVE()
GEOMETRIC_REPRESENTATION_ITEM()
RATIONAL_B_SPLINE_CURVE((1.,1.,1.,1.,1.,1.,1.,1.,1.,1.,1.,1.,1.,1.,1.,1.,
1.,1.,1.,1.,1.,1.,1.,1.,1.,1.,1.,1.,1.,1.,1.,1.,1.,1.,1.,1.,1.,1.,1.,1.,
1.,1.,1.,1.,1.,1.,1.,1.,1.,1.,1.,1.,1.,1.,1.,1.,1.,1.,1.,1.,1.,1.,1.,1.,
1.,1.,1.,1.,1.,1.))
REPRESENTATION_ITEM('')
);
#209=(
BOUNDED_CURVE()
B_SPLINE_CURVE(5,(#29492,#29493,#29494,#29495,#29496,#29497,#29498,#29499,
#29500,#29501,#29502,#29503,#29504,#29505,#29506,#29507,#29508,#29509,#29510,
#29511,#29512,#29513,#29514,#29515,#29516,#29517,#29518,#29519,#29520,#29521,
#29522,#29523,#29524,#29525,#29526,#29527,#29528,#29529,#29530,#29531,#29532,
#29533,#29534,#29535,#29536,#29537,#29538,#29539,#29540,#29541,#29542,#29543,
#29544,#29545,#29546,#29547,#29548,#29549,#29550,#29551,#29552,#29553,#29554,
#29555,#29556,#29557,#29558,#29559,#29560,#29561),.UNSPECIFIED.,.F.,.F.)
B_SPLINE_CURVE_WITH_KNOTS((6,1,1,1,1,1,1,1,1,1,1,1,1,1,1,1,1,1,1,1,1,1,
1,1,1,1,1,1,1,1,1,1,1,1,1,1,1,1,1,1,1,1,1,1,1,1,1,1,1,1,1,1,1,1,1,1,1,1,
1,1,1,1,1,1,1,6),(-1.,-0.984615384615383,-0.969230769230768,-0.953846153846152,
-0.938461538461537,-0.923076923076922,-0.907692307692306,-0.892307692307691,
-0.876923076923076,-0.86153846153846,-0.846153846153845,-0.83076923076923,
-0.815384615384614,-0.799999999999999,-0.784615384615384,-0.769230769230768,
-0.753846153846153,-0.738461538461538,-0.723076923076922,-0.707692307692307,
-0.692307692307692,-0.676923076923076,-0.661538461538461,-0.646153846153846,
-0.63076923076923,-0.615384615384615,-0.6,-0.584615384615384,-0.569230769230769,
-0.553846153846154,-0.538461538461538,-0.523076923076923,-0.507692307692308,
-0.492307692307692,-0.476923076923077,-0.461538461538462,-0.446153846153846,
-0.430769230769231,-0.415384615384615,-0.4,-0.384615384615385,-0.369230769230769,
-0.353846153846154,-0.338461538461538,-0.323076923076923,-0.307692307692308,
-0.292307692307692,-0.276923076923077,-0.261538461538462,-0.246153846153846,
-0.230769230769231,-0.215384615384615,-0.2,-0.184615384615385,-0.169230769230769,
-0.153846153846154,-0.138461538461538,-0.123076923076923,-0.107692307692308,
-0.0923076923076923,-0.0769230769230769,-0.0615384615384615,-0.0461538461538462,
-0.0307692307692308,-0.0153846153846154,0.),.UNSPECIFIED.)
CURVE()
GEOMETRIC_REPRESENTATION_ITEM()
RATIONAL_B_SPLINE_CURVE((1.,1.,1.,1.,1.,1.,1.,1.,1.,1.,1.,1.,1.,1.,1.,1.,
1.,1.,1.,1.,1.,1.,1.,1.,1.,1.,1.,1.,1.,1.,1.,1.,1.,1.,1.,1.,1.,1.,1.,1.,
1.,1.,1.,1.,1.,1.,1.,1.,1.,1.,1.,1.,1.,1.,1.,1.,1.,1.,1.,1.,1.,1.,1.,1.,
1.,1.,1.,1.,1.,1.))
REPRESENTATION_ITEM('')
);
#210=(
BOUNDED_CURVE()
B_SPLINE_CURVE(5,(#29708,#29709,#29710,#29711,#29712,#29713,#29714,#29715,
#29716,#29717,#29718,#29719,#29720,#29721,#29722,#29723,#29724,#29725,#29726,
#29727,#29728,#29729,#29730,#29731,#29732,#29733,#29734,#29735,#29736,#29737,
#29738,#29739,#29740,#29741,#29742,#29743,#29744,#29745,#29746,#29747,#29748,
#29749,#29750,#29751,#29752,#29753,#29754,#29755,#29756,#29757,#29758,#29759,
#29760,#29761,#29762,#29763,#29764,#29765,#29766,#29767,#29768,#29769,#29770,
#29771,#29772,#29773,#29774,#29775,#29776,#29777),.UNSPECIFIED.,.F.,.F.)
B_SPLINE_CURVE_WITH_KNOTS((6,1,1,1,1,1,1,1,1,1,1,1,1,1,1,1,1,1,1,1,1,1,
1,1,1,1,1,1,1,1,1,1,1,1,1,1,1,1,1,1,1,1,1,1,1,1,1,1,1,1,1,1,1,1,1,1,1,1,
1,1,1,1,1,1,1,6),(-1.,-0.984615384615383,-0.969230769230768,-0.953846153846152,
-0.938461538461537,-0.923076923076922,-0.907692307692306,-0.892307692307691,
-0.876923076923076,-0.86153846153846,-0.846153846153845,-0.83076923076923,
-0.815384615384614,-0.799999999999999,-0.784615384615384,-0.769230769230768,
-0.753846153846153,-0.738461538461538,-0.723076923076922,-0.707692307692307,
-0.692307692307692,-0.676923076923076,-0.661538461538461,-0.646153846153846,
-0.63076923076923,-0.615384615384615,-0.6,-0.584615384615384,-0.569230769230769,
-0.553846153846154,-0.538461538461538,-0.523076923076923,-0.507692307692308,
-0.492307692307692,-0.476923076923077,-0.461538461538462,-0.446153846153846,
-0.430769230769231,-0.415384615384615,-0.4,-0.384615384615385,-0.369230769230769,
-0.353846153846154,-0.338461538461538,-0.323076923076923,-0.307692307692308,
-0.292307692307692,-0.276923076923077,-0.261538461538462,-0.246153846153846,
-0.230769230769231,-0.215384615384615,-0.2,-0.184615384615385,-0.169230769230769,
-0.153846153846154,-0.138461538461538,-0.123076923076923,-0.107692307692308,
-0.0923076923076923,-0.0769230769230769,-0.0615384615384615,-0.0461538461538462,
-0.0307692307692308,-0.0153846153846154,0.),.UNSPECIFIED.)
CURVE()
GEOMETRIC_REPRESENTATION_ITEM()
RATIONAL_B_SPLINE_CURVE((1.,1.,1.,1.,1.,1.,1.,1.,1.,1.,1.,1.,1.,1.,1.,1.,
1.,1.,1.,1.,1.,1.,1.,1.,1.,1.,1.,1.,1.,1.,1.,1.,1.,1.,1.,1.,1.,1.,1.,1.,
1.,1.,1.,1.,1.,1.,1.,1.,1.,1.,1.,1.,1.,1.,1.,1.,1.,1.,1.,1.,1.,1.,1.,1.,
1.,1.,1.,1.,1.,1.))
REPRESENTATION_ITEM('')
);
#892=SHAPE_REPRESENTATION_RELATIONSHIP('SRR','None',#54122,#935);
#935=ADVANCED_BREP_SHAPE_REPRESENTATION('',(#1048),#53896);
#993=STYLED_ITEM('',(#54411),#1048);
#1048=MANIFOLD_SOLID_BREP('Body1',#11320);
#1214=FACE_BOUND('',#2627,.T.);
#1215=FACE_BOUND('',#2631,.T.);
#1216=FACE_BOUND('',#2712,.T.);
#1381=PLANE('',#12561);
#1382=PLANE('',#12562);
#1383=PLANE('',#12563);
#1384=PLANE('',#12564);
#1385=PLANE('',#12591);
#1386=PLANE('',#12592);
#1387=PLANE('',#12595);
#1388=PLANE('',#12598);
#1389=PLANE('',#12601);
#1390=PLANE('',#12604);
#1391=PLANE('',#12607);
#1392=PLANE('',#12610);
#1393=PLANE('',#12613);
#1394=PLANE('',#12616);
#1395=PLANE('',#12619);
#1396=PLANE('',#12622);
#1397=PLANE('',#12625);
#1398=PLANE('',#12628);
#1399=PLANE('',#12631);
#1400=PLANE('',#12634);
#1401=PLANE('',#12637);
#1402=PLANE('',#12640);
#1403=PLANE('',#12643);
#1404=PLANE('',#12646);
#1405=PLANE('',#12649);
#1406=PLANE('',#12650);
#1821=FACE_OUTER_BOUND('',#2623,.T.);
#1822=FACE_OUTER_BOUND('',#2624,.T.);
#1823=FACE_OUTER_BOUND('',#2625,.T.);
#1824=FACE_OUTER_BOUND('',#2626,.T.);
#1825=FACE_OUTER_BOUND('',#2628,.T.);
#1826=FACE_OUTER_BOUND('',#2629,.T.);
#1827=FACE_OUTER_BOUND('',#2630,.T.);
#1828=FACE_OUTER_BOUND('',#2632,.T.);
#1829=FACE_OUTER_BOUND('',#2633,.T.);
#1830=FACE_OUTER_BOUND('',#2634,.T.);
#1831=FACE_OUTER_BOUND('',#2635,.T.);
#1832=FACE_OUTER_BOUND('',#2636,.T.);
#1833=FACE_OUTER_BOUND('',#2637,.T.);
#1834=FACE_OUTER_BOUND('',#2638,.T.);
#1835=FACE_OUTER_BOUND('',#2639,.T.);
#1836=FACE_OUTER_BOUND('',#2640,.T.);
#1837=FACE_OUTER_BOUND('',#2641,.T.);
#1838=FACE_OUTER_BOUND('',#2642,.T.);
#1839=FACE_OUTER_BOUND('',#2643,.T.);
#1840=FACE_OUTER_BOUND('',#2644,.T.);
#1841=FACE_OUTER_BOUND('',#2645,.T.);
#1842=FACE_OUTER_BOUND('',#2646,.T.);
#1843=FACE_OUTER_BOUND('',#2647,.T.);
#1844=FACE_OUTER_BOUND('',#2648,.T.);
#1845=FACE_OUTER_BOUND('',#2649,.T.);
#1846=FACE_OUTER_BOUND('',#2650,.T.);
#1847=FACE_OUTER_BOUND('',#2651,.T.);
#1848=FACE_OUTER_BOUND('',#2652,.T.);
#1849=FACE_OUTER_BOUND('',#2653,.T.);
#1850=FACE_OUTER_BOUND('',#2654,.T.);
#1851=FACE_OUTER_BOUND('',#2655,.T.);
#1852=FACE_OUTER_BOUND('',#2656,.T.);
#1853=FACE_OUTER_BOUND('',#2657,.T.);
#1854=FACE_OUTER_BOUND('',#2658,.T.);
#1855=FACE_OUTER_BOUND('',#2659,.T.);
#1856=FACE_OUTER_BOUND('',#2660,.T.);
#1857=FACE_OUTER_BOUND('',#2661,.T.);
#1858=FACE_OUTER_BOUND('',#2662,.T.);
#1859=FACE_OUTER_BOUND('',#2663,.T.);
#1860=FACE_OUTER_BOUND('',#2664,.T.);
#1861=FACE_OUTER_BOUND('',#2665,.T.);
#1862=FACE_OUTER_BOUND('',#2666,.T.);
#1863=FACE_OUTER_BOUND('',#2667,.T.);
#1864=FACE_OUTER_BOUND('',#2668,.T.);
#1865=FACE_OUTER_BOUND('',#2669,.T.);
#1866=FACE_OUTER_BOUND('',#2670,.T.);
#1867=FACE_OUTER_BOUND('',#2671,.T.);
#1868=FACE_OUTER_BOUND('',#2672,.T.);
#1869=FACE_OUTER_BOUND('',#2673,.T.);
#1870=FACE_OUTER_BOUND('',#2674,.T.);
#1871=FACE_OUTER_BOUND('',#2675,.T.);
#1872=FACE_OUTER_BOUND('',#2676,.T.);
#1873=FACE_OUTER_BOUND('',#2677,.T.);
#1874=FACE_OUTER_BOUND('',#2678,.T.);
#1875=FACE_OUTER_BOUND('',#2679,.T.);
#1876=FACE_OUTER_BOUND('',#2680,.T.);
#1877=FACE_OUTER_BOUND('',#2681,.T.);
#1878=FACE_OUTER_BOUND('',#2682,.T.);
#1879=FACE_OUTER_BOUND('',#2683,.T.);
#1880=FACE_OUTER_BOUND('',#2684,.T.);
#1881=FACE_OUTER_BOUND('',#2685,.T.);
#1882=FACE_OUTER_BOUND('',#2686,.T.);
#1883=FACE_OUTER_BOUND('',#2687,.T.);
#1884=FACE_OUTER_BOUND('',#2688,.T.);
#1885=FACE_OUTER_BOUND('',#2689,.T.);
#1886=FACE_OUTER_BOUND('',#2690,.T.);
#1887=FACE_OUTER_BOUND('',#2691,.T.);
#1888=FACE_OUTER_BOUND('',#2692,.T.);
#1889=FACE_OUTER_BOUND('',#2693,.T.);
#1890=FACE_OUTER_BOUND('',#2694,.T.);
#1891=FACE_OUTER_BOUND('',#2695,.T.);
#1892=FACE_OUTER_BOUND('',#2696,.T.);
#1893=FACE_OUTER_BOUND('',#2697,.T.);
#1894=FACE_OUTER_BOUND('',#2698,.T.);
#1895=FACE_OUTER_BOUND('',#2699,.T.);
#1896=FACE_OUTER_BOUND('',#2700,.T.);
#1897=FACE_OUTER_BOUND('',#2701,.T.);
#1898=FACE_OUTER_BOUND('',#2702,.T.);
#1899=FACE_OUTER_BOUND('',#2703,.T.);
#1900=FACE_OUTER_BOUND('',#2704,.T.);
#1901=FACE_OUTER_BOUND('',#2705,.T.);
#1902=FACE_OUTER_BOUND('',#2706,.T.);
#1903=FACE_OUTER_BOUND('',#2707,.T.);
#1904=FACE_OUTER_BOUND('',#2708,.T.);
#1905=FACE_OUTER_BOUND('',#2709,.T.);
#1906=FACE_OUTER_BOUND('',#2710,.T.);
#1907=FACE_OUTER_BOUND('',#2711,.T.);
#1908=FACE_OUTER_BOUND('',#2713,.T.);
#2623=EDGE_LOOP('',(#8624,#8625,#8626,#8627));
#2624=EDGE_LOOP('',(#8628,#8629,#8630,#8631));
#2625=EDGE_LOOP('',(#8632,#8633,#8634,#8635));
#2626=EDGE_LOOP('',(#8636,#8637,#8638,#8639,#8640,#8641,#8642,#8643,#8644,
#8645,#8646,#8647,#8648,#8649,#8650,#8651,#8652,#8653,#8654,#8655,#8656,
#8657,#8658,#8659,#8660,#8661,#8662,#8663,#8664,#8665,#8666,#8667,#8668,
#8669,#8670,#8671,#8672,#8673,#8674,#8675,#8676,#8677,#8678,#8679,#8680,
#8681,#8682,#8683,#8684,#8685,#8686,#8687,#8688,#8689,#8690,#8691,#8692,
#8693,#8694,#8695,#8696,#8697,#8698,#8699,#8700,#8701,#8702,#8703,#8704,
#8705,#8706,#8707,#8708,#8709,#8710,#8711,#8712,#8713,#8714,#8715));
#2627=EDGE_LOOP('',(#8716,#8717,#8718,#8719));
#2628=EDGE_LOOP('',(#8720,#8721,#8722,#8723));
#2629=EDGE_LOOP('',(#8724,#8725,#8726,#8727));
#2630=EDGE_LOOP('',(#8728));
#2631=EDGE_LOOP('',(#8729,#8730,#8731,#8732));
#2632=EDGE_LOOP('',(#8733,#8734,#8735,#8736));
#2633=EDGE_LOOP('',(#8737,#8738,#8739,#8740));
#2634=EDGE_LOOP('',(#8741,#8742,#8743,#8744));
#2635=EDGE_LOOP('',(#8745,#8746,#8747,#8748));
#2636=EDGE_LOOP('',(#8749,#8750,#8751,#8752));
#2637=EDGE_LOOP('',(#8753,#8754,#8755,#8756));
#2638=EDGE_LOOP('',(#8757,#8758,#8759,#8760));
#2639=EDGE_LOOP('',(#8761,#8762,#8763,#8764));
#2640=EDGE_LOOP('',(#8765,#8766,#8767,#8768));
#2641=EDGE_LOOP('',(#8769,#8770,#8771,#8772));
#2642=EDGE_LOOP('',(#8773,#8774,#8775,#8776));
#2643=EDGE_LOOP('',(#8777,#8778,#8779,#8780));
#2644=EDGE_LOOP('',(#8781,#8782,#8783,#8784));
#2645=EDGE_LOOP('',(#8785,#8786,#8787,#8788));
#2646=EDGE_LOOP('',(#8789,#8790,#8791,#8792));
#2647=EDGE_LOOP('',(#8793,#8794,#8795,#8796));
#2648=EDGE_LOOP('',(#8797,#8798,#8799,#8800));
#2649=EDGE_LOOP('',(#8801,#8802,#8803,#8804));
#2650=EDGE_LOOP('',(#8805,#8806,#8807,#8808));
#2651=EDGE_LOOP('',(#8809,#8810,#8811,#8812));
#2652=EDGE_LOOP('',(#8813,#8814,#8815,#8816));
#2653=EDGE_LOOP('',(#8817,#8818,#8819,#8820));
#2654=EDGE_LOOP('',(#8821,#8822,#8823,#8824));
#2655=EDGE_LOOP('',(#8825,#8826,#8827,#8828));
#2656=EDGE_LOOP('',(#8829,#8830,#8831,#8832));
#2657=EDGE_LOOP('',(#8833,#8834,#8835,#8836));
#2658=EDGE_LOOP('',(#8837,#8838,#8839,#8840));
#2659=EDGE_LOOP('',(#8841,#8842,#8843,#8844));
#2660=EDGE_LOOP('',(#8845,#8846,#8847,#8848));
#2661=EDGE_LOOP('',(#8849,#8850,#8851,#8852));
#2662=EDGE_LOOP('',(#8853,#8854,#8855,#8856));
#2663=EDGE_LOOP('',(#8857,#8858,#8859,#8860));
#2664=EDGE_LOOP('',(#8861,#8862,#8863,#8864));
#2665=EDGE_LOOP('',(#8865,#8866,#8867,#8868));
#2666=EDGE_LOOP('',(#8869,#8870,#8871,#8872));
#2667=EDGE_LOOP('',(#8873,#8874,#8875,#8876));
#2668=EDGE_LOOP('',(#8877,#8878,#8879,#8880));
#2669=EDGE_LOOP('',(#8881,#8882,#8883,#8884));
#2670=EDGE_LOOP('',(#8885,#8886,#8887,#8888));
#2671=EDGE_LOOP('',(#8889,#8890,#8891,#8892));
#2672=EDGE_LOOP('',(#8893,#8894,#8895,#8896));
#2673=EDGE_LOOP('',(#8897,#8898,#8899,#8900));
#2674=EDGE_LOOP('',(#8901,#8902,#8903,#8904));
#2675=EDGE_LOOP('',(#8905,#8906,#8907,#8908));
#2676=EDGE_LOOP('',(#8909,#8910,#8911,#8912));
#2677=EDGE_LOOP('',(#8913,#8914,#8915,#8916));
#2678=EDGE_LOOP('',(#8917,#8918,#8919,#8920));
#2679=EDGE_LOOP('',(#8921,#8922,#8923,#8924));
#2680=EDGE_LOOP('',(#8925,#8926,#8927,#8928));
#2681=EDGE_LOOP('',(#8929,#8930,#8931,#8932));
#2682=EDGE_LOOP('',(#8933,#8934,#8935,#8936));
#2683=EDGE_LOOP('',(#8937,#8938,#8939,#8940));
#2684=EDGE_LOOP('',(#8941,#8942,#8943,#8944));
#2685=EDGE_LOOP('',(#8945,#8946,#8947,#8948));
#2686=EDGE_LOOP('',(#8949,#8950,#8951,#8952));
#2687=EDGE_LOOP('',(#8953,#8954,#8955,#8956));
#2688=EDGE_LOOP('',(#8957,#8958,#8959,#8960));
#2689=EDGE_LOOP('',(#8961,#8962,#8963,#8964));
#2690=EDGE_LOOP('',(#8965,#8966,#8967,#8968));
#2691=EDGE_LOOP('',(#8969,#8970,#8971,#8972));
#2692=EDGE_LOOP('',(#8973,#8974,#8975,#8976));
#2693=EDGE_LOOP('',(#8977,#8978,#8979,#8980));
#2694=EDGE_LOOP('',(#8981,#8982,#8983,#8984));
#2695=EDGE_LOOP('',(#8985,#8986,#8987,#8988));
#2696=EDGE_LOOP('',(#8989,#8990,#8991,#8992));
#2697=EDGE_LOOP('',(#8993,#8994,#8995,#8996));
#2698=EDGE_LOOP('',(#8997,#8998,#8999,#9000));
#2699=EDGE_LOOP('',(#9001,#9002,#9003,#9004));
#2700=EDGE_LOOP('',(#9005,#9006,#9007,#9008));
#2701=EDGE_LOOP('',(#9009,#9010,#9011,#9012));
#2702=EDGE_LOOP('',(#9013,#9014,#9015,#9016));
#2703=EDGE_LOOP('',(#9017,#9018,#9019,#9020));
#2704=EDGE_LOOP('',(#9021,#9022,#9023,#9024));
#2705=EDGE_LOOP('',(#9025,#9026,#9027,#9028));
#2706=EDGE_LOOP('',(#9029,#9030,#9031,#9032));
#2707=EDGE_LOOP('',(#9033,#9034,#9035,#9036));
#2708=EDGE_LOOP('',(#9037,#9038,#9039,#9040));
#2709=EDGE_LOOP('',(#9041,#9042,#9043,#9044));
#2710=EDGE_LOOP('',(#9045,#9046,#9047,#9048));
#2711=EDGE_LOOP('',(#9049,#9050,#9051,#9052,#9053,#9054,#9055,#9056,#9057,
#9058,#9059,#9060,#9061,#9062,#9063,#9064,#9065,#9066,#9067,#9068,#9069,
#9070,#9071,#9072,#9073,#9074,#9075,#9076,#9077,#9078,#9079,#9080,#9081,
#9082,#9083,#9084,#9085,#9086,#9087,#9088,#9089,#9090,#9091,#9092,#9093,
#9094,#9095,#9096,#9097,#9098,#9099,#9100,#9101,#9102,#9103,#9104,#9105,
#9106,#9107,#9108,#9109,#9110,#9111,#9112,#9113,#9114,#9115,#9116,#9117,
#9118,#9119,#9120,#9121,#9122,#9123,#9124,#9125,#9126,#9127,#9128));
#2712=EDGE_LOOP('',(#9129));
#2713=EDGE_LOOP('',(#9130,#9131,#9132,#9133));
#3222=LINE('',#18192,#3863);
#3223=LINE('',#18194,#3864);
#3224=LINE('',#18196,#3865);
#3225=LINE('',#18197,#3866);
#3226=LINE('',#18200,#3867);
#3227=LINE('',#18202,#3868);
#3228=LINE('',#18203,#3869);
#3229=LINE('',#18206,#3870);
#3230=LINE('',#18208,#3871);
#3231=LINE('',#18209,#3872);
#3232=LINE('',#18286,#3873);
#3233=LINE('',#18432,#3874);
#3234=LINE('',#18578,#3875);
#3235=LINE('',#18724,#3876);
#3236=LINE('',#18870,#3877);
#3237=LINE('',#19016,#3878);
#3238=LINE('',#19162,#3879);
#3239=LINE('',#19308,#3880);
#3240=LINE('',#19454,#3881);
#3241=LINE('',#19600,#3882);
#3242=LINE('',#19746,#3883);
#3243=LINE('',#19892,#3884);
#3244=LINE('',#20038,#3885);
#3245=LINE('',#20184,#3886);
#3246=LINE('',#20330,#3887);
#3247=LINE('',#20476,#3888);
#3248=LINE('',#20622,#3889);
#3249=LINE('',#20768,#3890);
#3250=LINE('',#20914,#3891);
#3251=LINE('',#21060,#3892);
#3252=LINE('',#21138,#3893);
#3253=LINE('',#21282,#3894);
#3254=LINE('',#21354,#3895);
#3255=LINE('',#21357,#3896);
#3256=LINE('',#21358,#3897);
#3257=LINE('',#21570,#3898);
#3258=LINE('',#21574,#3899);
#3259=LINE('',#21786,#3900);
#3260=LINE('',#21789,#3901);
#3261=LINE('',#21790,#3902);
#3262=LINE('',#22002,#3903);
#3263=LINE('',#22006,#3904);
#3264=LINE('',#22218,#3905);
#3265=LINE('',#22221,#3906);
#3266=LINE('',#22222,#3907);
#3267=LINE('',#22434,#3908);
#3268=LINE('',#22438,#3909);
#3269=LINE('',#22650,#3910);
#3270=LINE('',#22653,#3911);
#3271=LINE('',#22654,#3912);
#3272=LINE('',#22866,#3913);
#3273=LINE('',#22870,#3914);
#3274=LINE('',#23082,#3915);
#3275=LINE('',#23085,#3916);
#3276=LINE('',#23086,#3917);
#3277=LINE('',#23298,#3918);
#3278=LINE('',#23302,#3919);
#3279=LINE('',#23514,#3920);
#3280=LINE('',#23517,#3921);
#3281=LINE('',#23518,#3922);
#3282=LINE('',#23730,#3923);
#3283=LINE('',#23734,#3924);
#3284=LINE('',#23946,#3925);
#3285=LINE('',#23949,#3926);
#3286=LINE('',#23950,#3927);
#3287=LINE('',#24162,#3928);
#3288=LINE('',#24166,#3929);
#3289=LINE('',#24378,#3930);
#3290=LINE('',#24381,#3931);
#3291=LINE('',#24382,#3932);
#3292=LINE('',#24594,#3933);
#3293=LINE('',#24598,#3934);
#3294=LINE('',#24810,#3935);
#3295=LINE('',#24813,#3936);
#3296=LINE('',#24814,#3937);
#3297=LINE('',#25026,#3938);
#3298=LINE('',#25030,#3939);
#3299=LINE('',#25242,#3940);
#3300=LINE('',#25245,#3941);
#3301=LINE('',#25246,#3942);
#3302=LINE('',#25458,#3943);
#3303=LINE('',#25462,#3944);
#3304=LINE('',#25674,#3945);
#3305=LINE('',#25677,#3946);
#3306=LINE('',#25678,#3947);
#3307=LINE('',#25890,#3948);
#3308=LINE('',#25894,#3949);
#3309=LINE('',#26106,#3950);
#3310=LINE('',#26109,#3951);
#3311=LINE('',#26110,#3952);
#3312=LINE('',#26322,#3953);
#3313=LINE('',#26326,#3954);
#3314=LINE('',#26538,#3955);
#3315=LINE('',#26541,#3956);
#3316=LINE('',#26542,#3957);
#3317=LINE('',#26754,#3958);
#3318=LINE('',#26758,#3959);
#3319=LINE('',#26970,#3960);
#3320=LINE('',#26973,#3961);
#3321=LINE('',#26974,#3962);
#3322=LINE('',#27186,#3963);
#3323=LINE('',#27190,#3964);
#3324=LINE('',#27402,#3965);
#3325=LINE('',#27405,#3966);
#3326=LINE('',#27406,#3967);
#3327=LINE('',#27618,#3968);
#3328=LINE('',#27622,#3969);
#3329=LINE('',#27834,#3970);
#3330=LINE('',#27837,#3971);
#3331=LINE('',#27838,#3972);
#3332=LINE('',#28050,#3973);
#3333=LINE('',#28054,#3974);
#3334=LINE('',#28266,#3975);
#3335=LINE('',#28269,#3976);
#3336=LINE('',#28270,#3977);
#3337=LINE('',#28482,#3978);
#3338=LINE('',#28486,#3979);
#3339=LINE('',#28698,#3980);
#3340=LINE('',#28701,#3981);
#3341=LINE('',#28702,#3982);
#3342=LINE('',#28914,#3983);
#3343=LINE('',#28918,#3984);
#3344=LINE('',#29130,#3985);
#3345=LINE('',#29133,#3986);
#3346=LINE('',#29134,#3987);
#3347=LINE('',#29346,#3988);
#3348=LINE('',#29350,#3989);
#3349=LINE('',#29562,#3990);
#3350=LINE('',#29565,#3991);
#3351=LINE('',#29566,#3992);
#3352=LINE('',#29778,#3993);
#3863=VECTOR('',#14739,1.);
#3864=VECTOR('',#14740,1.);
#3865=VECTOR('',#14741,1.);
#3866=VECTOR('',#14742,1.);
#3867=VECTOR('',#14745,1.);
#3868=VECTOR('',#14746,1.);
#3869=VECTOR('',#14747,1.);
#3870=VECTOR('',#14750,1.);
#3871=VECTOR('',#14751,1.);
#3872=VECTOR('',#14752,1.);
#3873=VECTOR('',#14757,1.);
#3874=VECTOR('',#14760,1.);
#3875=VECTOR('',#14763,1.);
#3876=VECTOR('',#14766,1.);
#3877=VECTOR('',#14769,1.);
#3878=VECTOR('',#14772,1.);
#3879=VECTOR('',#14775,1.);
#3880=VECTOR('',#14778,1.);
#3881=VECTOR('',#14781,1.);
#3882=VECTOR('',#14784,1.);
#3883=VECTOR('',#14787,1.);
#3884=VECTOR('',#14790,1.);
#3885=VECTOR('',#14793,1.);
#3886=VECTOR('',#14796,1.);
#3887=VECTOR('',#14799,1.);
#3888=VECTOR('',#14802,1.);
#3889=VECTOR('',#14805,1.);
#3890=VECTOR('',#14808,1.);
#3891=VECTOR('',#14811,1.);
#3892=VECTOR('',#14814,1.);
#3893=VECTOR('',#14825,1.4);
#3894=VECTOR('',#14830,1.);
#3895=VECTOR('',#14831,1.);
#3896=VECTOR('',#14834,1.);
#3897=VECTOR('',#14835,1.);
#3898=VECTOR('',#14836,1.);
#3899=VECTOR('',#14841,1.);
#3900=VECTOR('',#14842,1.);
#3901=VECTOR('',#14845,1.);
#3902=VECTOR('',#14846,1.);
#3903=VECTOR('',#14847,1.);
#3904=VECTOR('',#14852,1.);
#3905=VECTOR('',#14853,1.);
#3906=VECTOR('',#14856,1.);
#3907=VECTOR('',#14857,1.);
#3908=VECTOR('',#14858,1.);
#3909=VECTOR('',#14863,1.);
#3910=VECTOR('',#14864,1.);
#3911=VECTOR('',#14867,1.);
#3912=VECTOR('',#14868,1.);
#3913=VECTOR('',#14869,1.);
#3914=VECTOR('',#14874,1.);
#3915=VECTOR('',#14875,1.);
#3916=VECTOR('',#14878,1.);
#3917=VECTOR('',#14879,1.);
#3918=VECTOR('',#14880,1.);
#3919=VECTOR('',#14885,1.);
#3920=VECTOR('',#14886,1.);
#3921=VECTOR('',#14889,1.);
#3922=VECTOR('',#14890,1.);
#3923=VECTOR('',#14891,1.);
#3924=VECTOR('',#14896,1.);
#3925=VECTOR('',#14897,1.);
#3926=VECTOR('',#14900,1.);
#3927=VECTOR('',#14901,1.);
#3928=VECTOR('',#14902,1.);
#3929=VECTOR('',#14907,1.);
#3930=VECTOR('',#14908,1.);
#3931=VECTOR('',#14911,1.);
#3932=VECTOR('',#14912,1.);
#3933=VECTOR('',#14913,1.);
#3934=VECTOR('',#14918,1.);
#3935=VECTOR('',#14919,1.);
#3936=VECTOR('',#14922,1.);
#3937=VECTOR('',#14923,1.);
#3938=VECTOR('',#14924,1.);
#3939=VECTOR('',#14929,1.);
#3940=VECTOR('',#14930,1.);
#3941=VECTOR('',#14933,1.);
#3942=VECTOR('',#14934,1.);
#3943=VECTOR('',#14935,1.);
#3944=VECTOR('',#14940,1.);
#3945=VECTOR('',#14941,1.);
#3946=VECTOR('',#14944,1.);
#3947=VECTOR('',#14945,1.);
#3948=VECTOR('',#14946,1.);
#3949=VECTOR('',#14951,1.);
#3950=VECTOR('',#14952,1.);
#3951=VECTOR('',#14955,1.);
#3952=VECTOR('',#14956,1.);
#3953=VECTOR('',#14957,1.);
#3954=VECTOR('',#14962,1.);
#3955=VECTOR('',#14963,1.);
#3956=VECTOR('',#14966,1.);
#3957=VECTOR('',#14967,1.);
#3958=VECTOR('',#14968,1.);
#3959=VECTOR('',#14973,1.);
#3960=VECTOR('',#14974,1.);
#3961=VECTOR('',#14977,1.);
#3962=VECTOR('',#14978,1.);
#3963=VECTOR('',#14979,1.);
#3964=VECTOR('',#14984,1.);
#3965=VECTOR('',#14985,1.);
#3966=VECTOR('',#14988,1.);
#3967=VECTOR('',#14989,1.);
#3968=VECTOR('',#14990,1.);
#3969=VECTOR('',#14995,1.);
#3970=VECTOR('',#14996,1.);
#3971=VECTOR('',#14999,1.);
#3972=VECTOR('',#15000,1.);
#3973=VECTOR('',#15001,1.);
#3974=VECTOR('',#15006,1.);
#3975=VECTOR('',#15007,1.);
#3976=VECTOR('',#15010,1.);
#3977=VECTOR('',#15011,1.);
#3978=VECTOR('',#15012,1.);
#3979=VECTOR('',#15017,1.);
#3980=VECTOR('',#15018,1.);
#3981=VECTOR('',#15021,1.);
#3982=VECTOR('',#15022,1.);
#3983=VECTOR('',#15023,1.);
#3984=VECTOR('',#15028,1.);
#3985=VECTOR('',#15029,1.);
#3986=VECTOR('',#15032,1.);
#3987=VECTOR('',#15033,1.);
#3988=VECTOR('',#15034,1.);
#3989=VECTOR('',#15039,1.);
#3990=VECTOR('',#15040,1.);
#3991=VECTOR('',#15043,1.);
#3992=VECTOR('',#15044,1.);
#3993=VECTOR('',#15045,1.);
#4610=CIRCLE('',#12565,1.75);
#4611=CIRCLE('',#12566,1.75);
#4612=CIRCLE('',#12567,1.75);
#4613=CIRCLE('',#12568,1.75);
#4614=CIRCLE('',#12569,1.75);
#4615=CIRCLE('',#12570,1.75);
#4616=CIRCLE('',#12571,1.75);
#4617=CIRCLE('',#12572,1.75);
#4618=CIRCLE('',#12573,1.75);
#4619=CIRCLE('',#12574,1.75);
#4620=CIRCLE('',#12575,1.75);
#4621=CIRCLE('',#12576,1.75);
#4622=CIRCLE('',#12577,1.75);
#4623=CIRCLE('',#12578,1.75);
#4624=CIRCLE('',#12579,1.75);
#4625=CIRCLE('',#12580,1.75);
#4626=CIRCLE('',#12581,1.75);
#4627=CIRCLE('',#12582,1.75);
#4628=CIRCLE('',#12583,1.75);
#4629=CIRCLE('',#12584,1.75);
#4630=CIRCLE('',#12585,0.6);
#4631=CIRCLE('',#12587,0.6);
#4632=CIRCLE('',#12589,1.4);
#4633=CIRCLE('',#12590,1.4);
#4634=CIRCLE('',#12594,1.75);
#4635=CIRCLE('',#12597,1.75);
#4636=CIRCLE('',#12600,1.75);
#4637=CIRCLE('',#12603,1.75);
#4638=CIRCLE('',#12606,1.75);
#4639=CIRCLE('',#12609,1.75);
#4640=CIRCLE('',#12612,1.75);
#4641=CIRCLE('',#12615,1.75);
#4642=CIRCLE('',#12618,1.75);
#4643=CIRCLE('',#12621,1.75);
#4644=CIRCLE('',#12624,1.75);
#4645=CIRCLE('',#12627,1.75);
#4646=CIRCLE('',#12630,1.75);
#4647=CIRCLE('',#12633,1.75);
#4648=CIRCLE('',#12636,1.75);
#4649=CIRCLE('',#12639,1.75);
#4650=CIRCLE('',#12642,1.75);
#4651=CIRCLE('',#12645,1.75);
#4652=CIRCLE('',#12648,1.75);
#4653=CIRCLE('',#12651,1.75);
#5222=VERTEX_POINT('',#18190);
#5223=VERTEX_POINT('',#18191);
#5224=VERTEX_POINT('',#18193);
#5225=VERTEX_POINT('',#18195);
#5226=VERTEX_POINT('',#18199);
#5227=VERTEX_POINT('',#18201);
#5228=VERTEX_POINT('',#18205);
#5229=VERTEX_POINT('',#18207);
#5230=VERTEX_POINT('',#18211);
#5231=VERTEX_POINT('',#18212);
#5232=VERTEX_POINT('',#18214);
#5233=VERTEX_POINT('',#18285);
#5234=VERTEX_POINT('',#18287);
#5235=VERTEX_POINT('',#18358);
#5236=VERTEX_POINT('',#18360);
#5237=VERTEX_POINT('',#18431);
#5238=VERTEX_POINT('',#18433);
#5239=VERTEX_POINT('',#18504);
#5240=VERTEX_POINT('',#18506);
#5241=VERTEX_POINT('',#18577);
#5242=VERTEX_POINT('',#18579);
#5243=VERTEX_POINT('',#18650);
#5244=VERTEX_POINT('',#18652);
#5245=VERTEX_POINT('',#18723);
#5246=VERTEX_POINT('',#18725);
#5247=VERTEX_POINT('',#18796);
#5248=VERTEX_POINT('',#18798);
#5249=VERTEX_POINT('',#18869);
#5250=VERTEX_POINT('',#18871);
#5251=VERTEX_POINT('',#18942);
#5252=VERTEX_POINT('',#18944);
#5253=VERTEX_POINT('',#19015);
#5254=VERTEX_POINT('',#19017);
#5255=VERTEX_POINT('',#19088);
#5256=VERTEX_POINT('',#19090);
#5257=VERTEX_POINT('',#19161);
#5258=VERTEX_POINT('',#19163);
#5259=VERTEX_POINT('',#19234);
#5260=VERTEX_POINT('',#19236);
#5261=VERTEX_POINT('',#19307);
#5262=VERTEX_POINT('',#19309);
#5263=VERTEX_POINT('',#19380);
#5264=VERTEX_POINT('',#19382);
#5265=VERTEX_POINT('',#19453);
#5266=VERTEX_POINT('',#19455);
#5267=VERTEX_POINT('',#19526);
#5268=VERTEX_POINT('',#19528);
#5269=VERTEX_POINT('',#19599);
#5270=VERTEX_POINT('',#19601);
#5271=VERTEX_POINT('',#19672);
#5272=VERTEX_POINT('',#19674);
#5273=VERTEX_POINT('',#19745);
#5274=VERTEX_POINT('',#19747);
#5275=VERTEX_POINT('',#19818);
#5276=VERTEX_POINT('',#19820);
#5277=VERTEX_POINT('',#19891);
#5278=VERTEX_POINT('',#19893);
#5279=VERTEX_POINT('',#19964);
#5280=VERTEX_POINT('',#19966);
#5281=VERTEX_POINT('',#20037);
#5282=VERTEX_POINT('',#20039);
#5283=VERTEX_POINT('',#20110);
#5284=VERTEX_POINT('',#20112);
#5285=VERTEX_POINT('',#20183);
#5286=VERTEX_POINT('',#20185);
#5287=VERTEX_POINT('',#20256);
#5288=VERTEX_POINT('',#20258);
#5289=VERTEX_POINT('',#20329);
#5290=VERTEX_POINT('',#20331);
#5291=VERTEX_POINT('',#20402);
#5292=VERTEX_POINT('',#20404);
#5293=VERTEX_POINT('',#20475);
#5294=VERTEX_POINT('',#20477);
#5295=VERTEX_POINT('',#20548);
#5296=VERTEX_POINT('',#20550);
#5297=VERTEX_POINT('',#20621);
#5298=VERTEX_POINT('',#20623);
#5299=VERTEX_POINT('',#20694);
#5300=VERTEX_POINT('',#20696);
#5301=VERTEX_POINT('',#20767);
#5302=VERTEX_POINT('',#20769);
#5303=VERTEX_POINT('',#20840);
#5304=VERTEX_POINT('',#20842);
#5305=VERTEX_POINT('',#20913);
#5306=VERTEX_POINT('',#20915);
#5307=VERTEX_POINT('',#20986);
#5308=VERTEX_POINT('',#20988);
#5309=VERTEX_POINT('',#21059);
#5310=VERTEX_POINT('',#21135);
#5311=VERTEX_POINT('',#21137);
#5312=VERTEX_POINT('',#21281);
#5313=VERTEX_POINT('',#21283);
#5314=VERTEX_POINT('',#21356);
#5315=VERTEX_POINT('',#21499);
#5316=VERTEX_POINT('',#21572);
#5317=VERTEX_POINT('',#21715);
#5318=VERTEX_POINT('',#21788);
#5319=VERTEX_POINT('',#21931);
#5320=VERTEX_POINT('',#22004);
#5321=VERTEX_POINT('',#22147);
#5322=VERTEX_POINT('',#22220);
#5323=VERTEX_POINT('',#22363);
#5324=VERTEX_POINT('',#22436);
#5325=VERTEX_POINT('',#22579);
#5326=VERTEX_POINT('',#22652);
#5327=VERTEX_POINT('',#22795);
#5328=VERTEX_POINT('',#22868);
#5329=VERTEX_POINT('',#23011);
#5330=VERTEX_POINT('',#23084);
#5331=VERTEX_POINT('',#23227);
#5332=VERTEX_POINT('',#23300);
#5333=VERTEX_POINT('',#23443);
#5334=VERTEX_POINT('',#23516);
#5335=VERTEX_POINT('',#23659);
#5336=VERTEX_POINT('',#23732);
#5337=VERTEX_POINT('',#23875);
#5338=VERTEX_POINT('',#23948);
#5339=VERTEX_POINT('',#24091);
#5340=VERTEX_POINT('',#24164);
#5341=VERTEX_POINT('',#24307);
#5342=VERTEX_POINT('',#24380);
#5343=VERTEX_POINT('',#24523);
#5344=VERTEX_POINT('',#24596);
#5345=VERTEX_POINT('',#24739);
#5346=VERTEX_POINT('',#24812);
#5347=VERTEX_POINT('',#24955);
#5348=VERTEX_POINT('',#25028);
#5349=VERTEX_POINT('',#25171);
#5350=VERTEX_POINT('',#25244);
#5351=VERTEX_POINT('',#25387);
#5352=VERTEX_POINT('',#25460);
#5353=VERTEX_POINT('',#25603);
#5354=VERTEX_POINT('',#25676);
#5355=VERTEX_POINT('',#25819);
#5356=VERTEX_POINT('',#25892);
#5357=VERTEX_POINT('',#26035);
#5358=VERTEX_POINT('',#26108);
#5359=VERTEX_POINT('',#26251);
#5360=VERTEX_POINT('',#26324);
#5361=VERTEX_POINT('',#26467);
#5362=VERTEX_POINT('',#26540);
#5363=VERTEX_POINT('',#26683);
#5364=VERTEX_POINT('',#26756);
#5365=VERTEX_POINT('',#26899);
#5366=VERTEX_POINT('',#26972);
#5367=VERTEX_POINT('',#27115);
#5368=VERTEX_POINT('',#27188);
#5369=VERTEX_POINT('',#27331);
#5370=VERTEX_POINT('',#27404);
#5371=VERTEX_POINT('',#27547);
#5372=VERTEX_POINT('',#27620);
#5373=VERTEX_POINT('',#27763);
#5374=VERTEX_POINT('',#27836);
#5375=VERTEX_POINT('',#27979);
#5376=VERTEX_POINT('',#28052);
#5377=VERTEX_POINT('',#28195);
#5378=VERTEX_POINT('',#28268);
#5379=VERTEX_POINT('',#28411);
#5380=VERTEX_POINT('',#28484);
#5381=VERTEX_POINT('',#28627);
#5382=VERTEX_POINT('',#28700);
#5383=VERTEX_POINT('',#28843);
#5384=VERTEX_POINT('',#28916);
#5385=VERTEX_POINT('',#29059);
#5386=VERTEX_POINT('',#29132);
#5387=VERTEX_POINT('',#29275);
#5388=VERTEX_POINT('',#29348);
#5389=VERTEX_POINT('',#29491);
#5390=VERTEX_POINT('',#29564);
#5391=VERTEX_POINT('',#29707);
#6454=EDGE_CURVE('',#5222,#5223,#3222,.T.);
#6455=EDGE_CURVE('',#5224,#5222,#3223,.T.);
#6456=EDGE_CURVE('',#5225,#5224,#3224,.T.);
#6457=EDGE_CURVE('',#5223,#5225,#3225,.T.);
#6458=EDGE_CURVE('',#5226,#5222,#3226,.T.);
#6459=EDGE_CURVE('',#5226,#5227,#3227,.T.);
#6460=EDGE_CURVE('',#5224,#5227,#3228,.T.);
#6461=EDGE_CURVE('',#5228,#5226,#3229,.T.);
#6462=EDGE_CURVE('',#5229,#5228,#3230,.T.);
#6463=EDGE_CURVE('',#5227,#5229,#3231,.T.);
#6464=EDGE_CURVE('',#5230,#5231,#4610,.T.);
#6465=EDGE_CURVE('',#5231,#5232,#131,.T.);
#6466=EDGE_CURVE('',#5232,#5233,#3232,.T.);
#6467=EDGE_CURVE('',#5233,#5234,#132,.T.);
#6468=EDGE_CURVE('',#5234,#5235,#4611,.T.);
#6469=EDGE_CURVE('',#5235,#5236,#133,.T.);
#6470=EDGE_CURVE('',#5236,#5237,#3233,.T.);
#6471=EDGE_CURVE('',#5237,#5238,#134,.T.);
#6472=EDGE_CURVE('',#5238,#5239,#4612,.T.);
#6473=EDGE_CURVE('',#5239,#5240,#135,.T.);
#6474=EDGE_CURVE('',#5240,#5241,#3234,.T.);
#6475=EDGE_CURVE('',#5241,#5242,#136,.T.);
#6476=EDGE_CURVE('',#5242,#5243,#4613,.T.);
#6477=EDGE_CURVE('',#5243,#5244,#137,.T.);
#6478=EDGE_CURVE('',#5244,#5245,#3235,.T.);
#6479=EDGE_CURVE('',#5245,#5246,#138,.T.);
#6480=EDGE_CURVE('',#5246,#5247,#4614,.T.);
#6481=EDGE_CURVE('',#5247,#5248,#139,.T.);
#6482=EDGE_CURVE('',#5248,#5249,#3236,.T.);
#6483=EDGE_CURVE('',#5249,#5250,#140,.T.);
#6484=EDGE_CURVE('',#5250,#5251,#4615,.T.);
#6485=EDGE_CURVE('',#5251,#5252,#141,.T.);
#6486=EDGE_CURVE('',#5252,#5253,#3237,.T.);
#6487=EDGE_CURVE('',#5253,#5254,#142,.T.);
#6488=EDGE_CURVE('',#5254,#5255,#4616,.T.);
#6489=EDGE_CURVE('',#5255,#5256,#143,.T.);
#6490=EDGE_CURVE('',#5256,#5257,#3238,.T.);
#6491=EDGE_CURVE('',#5257,#5258,#144,.T.);
#6492=EDGE_CURVE('',#5258,#5259,#4617,.T.);
#6493=EDGE_CURVE('',#5259,#5260,#145,.T.);
#6494=EDGE_CURVE('',#5260,#5261,#3239,.T.);
#6495=EDGE_CURVE('',#5261,#5262,#146,.T.);
#6496=EDGE_CURVE('',#5262,#5263,#4618,.T.);
#6497=EDGE_CURVE('',#5263,#5264,#147,.T.);
#6498=EDGE_CURVE('',#5264,#5265,#3240,.T.);
#6499=EDGE_CURVE('',#5265,#5266,#148,.T.);
#6500=EDGE_CURVE('',#5266,#5267,#4619,.T.);
#6501=EDGE_CURVE('',#5267,#5268,#149,.T.);
#6502=EDGE_CURVE('',#5268,#5269,#3241,.T.);
#6503=EDGE_CURVE('',#5269,#5270,#150,.T.);
#6504=EDGE_CURVE('',#5270,#5271,#4620,.T.);
#6505=EDGE_CURVE('',#5271,#5272,#151,.T.);
#6506=EDGE_CURVE('',#5272,#5273,#3242,.T.);
#6507=EDGE_CURVE('',#5273,#5274,#152,.T.);
#6508=EDGE_CURVE('',#5274,#5275,#4621,.T.);
#6509=EDGE_CURVE('',#5275,#5276,#153,.T.);
#6510=EDGE_CURVE('',#5276,#5277,#3243,.T.);
#6511=EDGE_CURVE('',#5277,#5278,#154,.T.);
#6512=EDGE_CURVE('',#5278,#5279,#4622,.T.);
#6513=EDGE_CURVE('',#5279,#5280,#155,.T.);
#6514=EDGE_CURVE('',#5280,#5281,#3244,.T.);
#6515=EDGE_CURVE('',#5281,#5282,#156,.T.);
#6516=EDGE_CURVE('',#5282,#5283,#4623,.T.);
#6517=EDGE_CURVE('',#5283,#5284,#157,.T.);
#6518=EDGE_CURVE('',#5284,#5285,#3245,.T.);
#6519=EDGE_CURVE('',#5285,#5286,#158,.T.);
#6520=EDGE_CURVE('',#5286,#5287,#4624,.T.);
#6521=EDGE_CURVE('',#5287,#5288,#159,.T.);
#6522=EDGE_CURVE('',#5288,#5289,#3246,.T.);
#6523=EDGE_CURVE('',#5289,#5290,#160,.T.);
#6524=EDGE_CURVE('',#5290,#5291,#4625,.T.);
#6525=EDGE_CURVE('',#5291,#5292,#161,.T.);
#6526=EDGE_CURVE('',#5292,#5293,#3247,.T.);
#6527=EDGE_CURVE('',#5293,#5294,#162,.T.);
#6528=EDGE_CURVE('',#5294,#5295,#4626,.T.);
#6529=EDGE_CURVE('',#5295,#5296,#163,.T.);
#6530=EDGE_CURVE('',#5296,#5297,#3248,.T.);
#6531=EDGE_CURVE('',#5297,#5298,#164,.T.);
#6532=EDGE_CURVE('',#5298,#5299,#4627,.T.);
#6533=EDGE_CURVE('',#5299,#5300,#165,.T.);
#6534=EDGE_CURVE('',#5300,#5301,#3249,.T.);
#6535=EDGE_CURVE('',#5301,#5302,#166,.T.);
#6536=EDGE_CURVE('',#5302,#5303,#4628,.T.);
#6537=EDGE_CURVE('',#5303,#5304,#167,.T.);
#6538=EDGE_CURVE('',#5304,#5305,#3250,.T.);
#6539=EDGE_CURVE('',#5305,#5306,#168,.T.);
#6540=EDGE_CURVE('',#5306,#5307,#4629,.T.);
#6541=EDGE_CURVE('',#5307,#5308,#169,.T.);
#6542=EDGE_CURVE('',#5308,#5309,#3251,.T.);
#6543=EDGE_CURVE('',#5309,#5230,#170,.T.);
#6544=EDGE_CURVE('',#5229,#5225,#4630,.T.);
#6545=EDGE_CURVE('',#5223,#5228,#4631,.T.);
#6546=EDGE_CURVE('',#5310,#5310,#4632,.T.);
#6547=EDGE_CURVE('',#5310,#5311,#3252,.T.);
#6548=EDGE_CURVE('',#5311,#5311,#4633,.T.);
#6549=EDGE_CURVE('',#5312,#5307,#3253,.T.);
#6550=EDGE_CURVE('',#5313,#5312,#171,.T.);
#6551=EDGE_CURVE('',#5308,#5313,#3254,.T.);
#6552=EDGE_CURVE('',#5314,#5313,#3255,.T.);
#6553=EDGE_CURVE('',#5309,#5314,#3256,.T.);
#6554=EDGE_CURVE('',#5315,#5314,#172,.T.);
#6555=EDGE_CURVE('',#5230,#5315,#3257,.T.);
#6556=EDGE_CURVE('',#5316,#5315,#4634,.T.);
#6557=EDGE_CURVE('',#5316,#5231,#3258,.T.);
#6558=EDGE_CURVE('',#5317,#5316,#173,.T.);
#6559=EDGE_CURVE('',#5232,#5317,#3259,.T.);
#6560=EDGE_CURVE('',#5318,#5317,#3260,.T.);
#6561=EDGE_CURVE('',#5233,#5318,#3261,.T.);
#6562=EDGE_CURVE('',#5319,#5318,#174,.T.);
#6563=EDGE_CURVE('',#5234,#5319,#3262,.T.);
#6564=EDGE_CURVE('',#5320,#5319,#4635,.T.);
#6565=EDGE_CURVE('',#5320,#5235,#3263,.T.);
#6566=EDGE_CURVE('',#5321,#5320,#175,.T.);
#6567=EDGE_CURVE('',#5236,#5321,#3264,.T.);
#6568=EDGE_CURVE('',#5322,#5321,#3265,.T.);
#6569=EDGE_CURVE('',#5237,#5322,#3266,.T.);
#6570=EDGE_CURVE('',#5323,#5322,#176,.T.);
#6571=EDGE_CURVE('',#5238,#5323,#3267,.T.);
#6572=EDGE_CURVE('',#5324,#5323,#4636,.T.);
#6573=EDGE_CURVE('',#5324,#5239,#3268,.T.);
#6574=EDGE_CURVE('',#5325,#5324,#177,.T.);
#6575=EDGE_CURVE('',#5240,#5325,#3269,.T.);
#6576=EDGE_CURVE('',#5326,#5325,#3270,.T.);
#6577=EDGE_CURVE('',#5241,#5326,#3271,.T.);
#6578=EDGE_CURVE('',#5327,#5326,#178,.T.);
#6579=EDGE_CURVE('',#5242,#5327,#3272,.T.);
#6580=EDGE_CURVE('',#5328,#5327,#4637,.T.);
#6581=EDGE_CURVE('',#5328,#5243,#3273,.T.);
#6582=EDGE_CURVE('',#5329,#5328,#179,.T.);
#6583=EDGE_CURVE('',#5244,#5329,#3274,.T.);
#6584=EDGE_CURVE('',#5330,#5329,#3275,.T.);
#6585=EDGE_CURVE('',#5245,#5330,#3276,.T.);
#6586=EDGE_CURVE('',#5331,#5330,#180,.T.);
#6587=EDGE_CURVE('',#5246,#5331,#3277,.T.);
#6588=EDGE_CURVE('',#5332,#5331,#4638,.T.);
#6589=EDGE_CURVE('',#5332,#5247,#3278,.T.);
#6590=EDGE_CURVE('',#5333,#5332,#181,.T.);
#6591=EDGE_CURVE('',#5248,#5333,#3279,.T.);
#6592=EDGE_CURVE('',#5334,#5333,#3280,.T.);
#6593=EDGE_CURVE('',#5249,#5334,#3281,.T.);
#6594=EDGE_CURVE('',#5335,#5334,#182,.T.);
#6595=EDGE_CURVE('',#5250,#5335,#3282,.T.);
#6596=EDGE_CURVE('',#5336,#5335,#4639,.T.);
#6597=EDGE_CURVE('',#5336,#5251,#3283,.T.);
#6598=EDGE_CURVE('',#5337,#5336,#183,.T.);
#6599=EDGE_CURVE('',#5252,#5337,#3284,.T.);
#6600=EDGE_CURVE('',#5338,#5337,#3285,.T.);
#6601=EDGE_CURVE('',#5253,#5338,#3286,.T.);
#6602=EDGE_CURVE('',#5339,#5338,#184,.T.);
#6603=EDGE_CURVE('',#5254,#5339,#3287,.T.);
#6604=EDGE_CURVE('',#5340,#5339,#4640,.T.);
#6605=EDGE_CURVE('',#5340,#5255,#3288,.T.);
#6606=EDGE_CURVE('',#5341,#5340,#185,.T.);
#6607=EDGE_CURVE('',#5256,#5341,#3289,.T.);
#6608=EDGE_CURVE('',#5342,#5341,#3290,.T.);
#6609=EDGE_CURVE('',#5257,#5342,#3291,.T.);
#6610=EDGE_CURVE('',#5343,#5342,#186,.T.);
#6611=EDGE_CURVE('',#5258,#5343,#3292,.T.);
#6612=EDGE_CURVE('',#5344,#5343,#4641,.T.);
#6613=EDGE_CURVE('',#5344,#5259,#3293,.T.);
#6614=EDGE_CURVE('',#5345,#5344,#187,.T.);
#6615=EDGE_CURVE('',#5260,#5345,#3294,.T.);
#6616=EDGE_CURVE('',#5346,#5345,#3295,.T.);
#6617=EDGE_CURVE('',#5261,#5346,#3296,.T.);
#6618=EDGE_CURVE('',#5347,#5346,#188,.T.);
#6619=EDGE_CURVE('',#5262,#5347,#3297,.T.);
#6620=EDGE_CURVE('',#5348,#5347,#4642,.T.);
#6621=EDGE_CURVE('',#5348,#5263,#3298,.T.);
#6622=EDGE_CURVE('',#5349,#5348,#189,.T.);
#6623=EDGE_CURVE('',#5264,#5349,#3299,.T.);
#6624=EDGE_CURVE('',#5350,#5349,#3300,.T.);
#6625=EDGE_CURVE('',#5265,#5350,#3301,.T.);
#6626=EDGE_CURVE('',#5351,#5350,#190,.T.);
#6627=EDGE_CURVE('',#5266,#5351,#3302,.T.);
#6628=EDGE_CURVE('',#5352,#5351,#4643,.T.);
#6629=EDGE_CURVE('',#5352,#5267,#3303,.T.);
#6630=EDGE_CURVE('',#5353,#5352,#191,.T.);
#6631=EDGE_CURVE('',#5268,#5353,#3304,.T.);
#6632=EDGE_CURVE('',#5354,#5353,#3305,.T.);
#6633=EDGE_CURVE('',#5269,#5354,#3306,.T.);
#6634=EDGE_CURVE('',#5355,#5354,#192,.T.);
#6635=EDGE_CURVE('',#5270,#5355,#3307,.T.);
#6636=EDGE_CURVE('',#5356,#5355,#4644,.T.);
#6637=EDGE_CURVE('',#5356,#5271,#3308,.T.);
#6638=EDGE_CURVE('',#5357,#5356,#193,.T.);
#6639=EDGE_CURVE('',#5272,#5357,#3309,.T.);
#6640=EDGE_CURVE('',#5358,#5357,#3310,.T.);
#6641=EDGE_CURVE('',#5273,#5358,#3311,.T.);
#6642=EDGE_CURVE('',#5359,#5358,#194,.T.);
#6643=EDGE_CURVE('',#5274,#5359,#3312,.T.);
#6644=EDGE_CURVE('',#5360,#5359,#4645,.T.);
#6645=EDGE_CURVE('',#5360,#5275,#3313,.T.);
#6646=EDGE_CURVE('',#5361,#5360,#195,.T.);
#6647=EDGE_CURVE('',#5276,#5361,#3314,.T.);
#6648=EDGE_CURVE('',#5362,#5361,#3315,.T.);
#6649=EDGE_CURVE('',#5277,#5362,#3316,.T.);
#6650=EDGE_CURVE('',#5363,#5362,#196,.T.);
#6651=EDGE_CURVE('',#5278,#5363,#3317,.T.);
#6652=EDGE_CURVE('',#5364,#5363,#4646,.T.);
#6653=EDGE_CURVE('',#5364,#5279,#3318,.T.);
#6654=EDGE_CURVE('',#5365,#5364,#197,.T.);
#6655=EDGE_CURVE('',#5280,#5365,#3319,.T.);
#6656=EDGE_CURVE('',#5366,#5365,#3320,.T.);
#6657=EDGE_CURVE('',#5281,#5366,#3321,.T.);
#6658=EDGE_CURVE('',#5367,#5366,#198,.T.);
#6659=EDGE_CURVE('',#5282,#5367,#3322,.T.);
#6660=EDGE_CURVE('',#5368,#5367,#4647,.T.);
#6661=EDGE_CURVE('',#5368,#5283,#3323,.T.);
#6662=EDGE_CURVE('',#5369,#5368,#199,.T.);
#6663=EDGE_CURVE('',#5284,#5369,#3324,.T.);
#6664=EDGE_CURVE('',#5370,#5369,#3325,.T.);
#6665=EDGE_CURVE('',#5285,#5370,#3326,.T.);
#6666=EDGE_CURVE('',#5371,#5370,#200,.T.);
#6667=EDGE_CURVE('',#5286,#5371,#3327,.T.);
#6668=EDGE_CURVE('',#5372,#5371,#4648,.T.);
#6669=EDGE_CURVE('',#5372,#5287,#3328,.T.);
#6670=EDGE_CURVE('',#5373,#5372,#201,.T.);
#6671=EDGE_CURVE('',#5288,#5373,#3329,.T.);
#6672=EDGE_CURVE('',#5374,#5373,#3330,.T.);
#6673=EDGE_CURVE('',#5289,#5374,#3331,.T.);
#6674=EDGE_CURVE('',#5375,#5374,#202,.T.);
#6675=EDGE_CURVE('',#5290,#5375,#3332,.T.);
#6676=EDGE_CURVE('',#5376,#5375,#4649,.T.);
#6677=EDGE_CURVE('',#5376,#5291,#3333,.T.);
#6678=EDGE_CURVE('',#5377,#5376,#203,.T.);
#6679=EDGE_CURVE('',#5292,#5377,#3334,.T.);
#6680=EDGE_CURVE('',#5378,#5377,#3335,.T.);
#6681=EDGE_CURVE('',#5293,#5378,#3336,.T.);
#6682=EDGE_CURVE('',#5379,#5378,#204,.T.);
#6683=EDGE_CURVE('',#5294,#5379,#3337,.T.);
#6684=EDGE_CURVE('',#5380,#5379,#4650,.T.);
#6685=EDGE_CURVE('',#5380,#5295,#3338,.T.);
#6686=EDGE_CURVE('',#5381,#5380,#205,.T.);
#6687=EDGE_CURVE('',#5296,#5381,#3339,.T.);
#6688=EDGE_CURVE('',#5382,#5381,#3340,.T.);
#6689=EDGE_CURVE('',#5297,#5382,#3341,.T.);
#6690=EDGE_CURVE('',#5383,#5382,#206,.T.);
#6691=EDGE_CURVE('',#5298,#5383,#3342,.T.);
#6692=EDGE_CURVE('',#5384,#5383,#4651,.T.);
#6693=EDGE_CURVE('',#5384,#5299,#3343,.T.);
#6694=EDGE_CURVE('',#5385,#5384,#207,.T.);
#6695=EDGE_CURVE('',#5300,#5385,#3344,.T.);
#6696=EDGE_CURVE('',#5386,#5385,#3345,.T.);
#6697=EDGE_CURVE('',#5301,#5386,#3346,.T.);
#6698=EDGE_CURVE('',#5387,#5386,#208,.T.);
#6699=EDGE_CURVE('',#5302,#5387,#3347,.T.);
#6700=EDGE_CURVE('',#5388,#5387,#4652,.T.);
#6701=EDGE_CURVE('',#5388,#5303,#3348,.T.);
#6702=EDGE_CURVE('',#5389,#5388,#209,.T.);
#6703=EDGE_CURVE('',#5304,#5389,#3349,.T.);
#6704=EDGE_CURVE('',#5390,#5389,#3350,.T.);
#6705=EDGE_CURVE('',#5305,#5390,#3351,.T.);
#6706=EDGE_CURVE('',#5391,#5390,#210,.T.);
#6707=EDGE_CURVE('',#5306,#5391,#3352,.T.);
#6708=EDGE_CURVE('',#5312,#5391,#4653,.T.);
#8624=ORIENTED_EDGE('',*,*,#6454,.F.);
#8625=ORIENTED_EDGE('',*,*,#6455,.F.);
#8626=ORIENTED_EDGE('',*,*,#6456,.F.);
#8627=ORIENTED_EDGE('',*,*,#6457,.F.);
#8628=ORIENTED_EDGE('',*,*,#6458,.F.);
#8629=ORIENTED_EDGE('',*,*,#6459,.T.);
#8630=ORIENTED_EDGE('',*,*,#6460,.F.);
#8631=ORIENTED_EDGE('',*,*,#6455,.T.);
#8632=ORIENTED_EDGE('',*,*,#6461,.F.);
#8633=ORIENTED_EDGE('',*,*,#6462,.F.);
#8634=ORIENTED_EDGE('',*,*,#6463,.F.);
#8635=ORIENTED_EDGE('',*,*,#6459,.F.);
#8636=ORIENTED_EDGE('',*,*,#6464,.T.);
#8637=ORIENTED_EDGE('',*,*,#6465,.T.);
#8638=ORIENTED_EDGE('',*,*,#6466,.T.);
#8639=ORIENTED_EDGE('',*,*,#6467,.T.);
#8640=ORIENTED_EDGE('',*,*,#6468,.T.);
#8641=ORIENTED_EDGE('',*,*,#6469,.T.);
#8642=ORIENTED_EDGE('',*,*,#6470,.T.);
#8643=ORIENTED_EDGE('',*,*,#6471,.T.);
#8644=ORIENTED_EDGE('',*,*,#6472,.T.);
#8645=ORIENTED_EDGE('',*,*,#6473,.T.);
#8646=ORIENTED_EDGE('',*,*,#6474,.T.);
#8647=ORIENTED_EDGE('',*,*,#6475,.T.);
#8648=ORIENTED_EDGE('',*,*,#6476,.T.);
#8649=ORIENTED_EDGE('',*,*,#6477,.T.);
#8650=ORIENTED_EDGE('',*,*,#6478,.T.);
#8651=ORIENTED_EDGE('',*,*,#6479,.T.);
#8652=ORIENTED_EDGE('',*,*,#6480,.T.);
#8653=ORIENTED_EDGE('',*,*,#6481,.T.);
#8654=ORIENTED_EDGE('',*,*,#6482,.T.);
#8655=ORIENTED_EDGE('',*,*,#6483,.T.);
#8656=ORIENTED_EDGE('',*,*,#6484,.T.);
#8657=ORIENTED_EDGE('',*,*,#6485,.T.);
#8658=ORIENTED_EDGE('',*,*,#6486,.T.);
#8659=ORIENTED_EDGE('',*,*,#6487,.T.);
#8660=ORIENTED_EDGE('',*,*,#6488,.T.);
#8661=ORIENTED_EDGE('',*,*,#6489,.T.);
#8662=ORIENTED_EDGE('',*,*,#6490,.T.);
#8663=ORIENTED_EDGE('',*,*,#6491,.T.);
#8664=ORIENTED_EDGE('',*,*,#6492,.T.);
#8665=ORIENTED_EDGE('',*,*,#6493,.T.);
#8666=ORIENTED_EDGE('',*,*,#6494,.T.);
#8667=ORIENTED_EDGE('',*,*,#6495,.T.);
#8668=ORIENTED_EDGE('',*,*,#6496,.T.);
#8669=ORIENTED_EDGE('',*,*,#6497,.T.);
#8670=ORIENTED_EDGE('',*,*,#6498,.T.);
#8671=ORIENTED_EDGE('',*,*,#6499,.T.);
#8672=ORIENTED_EDGE('',*,*,#6500,.T.);
#8673=ORIENTED_EDGE('',*,*,#6501,.T.);
#8674=ORIENTED_EDGE('',*,*,#6502,.T.);
#8675=ORIENTED_EDGE('',*,*,#6503,.T.);
#8676=ORIENTED_EDGE('',*,*,#6504,.T.);
#8677=ORIENTED_EDGE('',*,*,#6505,.T.);
#8678=ORIENTED_EDGE('',*,*,#6506,.T.);
#8679=ORIENTED_EDGE('',*,*,#6507,.T.);
#8680=ORIENTED_EDGE('',*,*,#6508,.T.);
#8681=ORIENTED_EDGE('',*,*,#6509,.T.);
#8682=ORIENTED_EDGE('',*,*,#6510,.T.);
#8683=ORIENTED_EDGE('',*,*,#6511,.T.);
#8684=ORIENTED_EDGE('',*,*,#6512,.T.);
#8685=ORIENTED_EDGE('',*,*,#6513,.T.);
#8686=ORIENTED_EDGE('',*,*,#6514,.T.);
#8687=ORIENTED_EDGE('',*,*,#6515,.T.);
#8688=ORIENTED_EDGE('',*,*,#6516,.T.);
#8689=ORIENTED_EDGE('',*,*,#6517,.T.);
#8690=ORIENTED_EDGE('',*,*,#6518,.T.);
#8691=ORIENTED_EDGE('',*,*,#6519,.T.);
#8692=ORIENTED_EDGE('',*,*,#6520,.T.);
#8693=ORIENTED_EDGE('',*,*,#6521,.T.);
#8694=ORIENTED_EDGE('',*,*,#6522,.T.);
#8695=ORIENTED_EDGE('',*,*,#6523,.T.);
#8696=ORIENTED_EDGE('',*,*,#6524,.T.);
#8697=ORIENTED_EDGE('',*,*,#6525,.T.);
#8698=ORIENTED_EDGE('',*,*,#6526,.T.);
#8699=ORIENTED_EDGE('',*,*,#6527,.T.);
#8700=ORIENTED_EDGE('',*,*,#6528,.T.);
#8701=ORIENTED_EDGE('',*,*,#6529,.T.);
#8702=ORIENTED_EDGE('',*,*,#6530,.T.);
#8703=ORIENTED_EDGE('',*,*,#6531,.T.);
#8704=ORIENTED_EDGE('',*,*,#6532,.T.);
#8705=ORIENTED_EDGE('',*,*,#6533,.T.);
#8706=ORIENTED_EDGE('',*,*,#6534,.T.);
#8707=ORIENTED_EDGE('',*,*,#6535,.T.);
#8708=ORIENTED_EDGE('',*,*,#6536,.T.);
#8709=ORIENTED_EDGE('',*,*,#6537,.T.);
#8710=ORIENTED_EDGE('',*,*,#6538,.T.);
#8711=ORIENTED_EDGE('',*,*,#6539,.T.);
#8712=ORIENTED_EDGE('',*,*,#6540,.T.);
#8713=ORIENTED_EDGE('',*,*,#6541,.T.);
#8714=ORIENTED_EDGE('',*,*,#6542,.T.);
#8715=ORIENTED_EDGE('',*,*,#6543,.T.);
#8716=ORIENTED_EDGE('',*,*,#6456,.T.);
#8717=ORIENTED_EDGE('',*,*,#6460,.T.);
#8718=ORIENTED_EDGE('',*,*,#6463,.T.);
#8719=ORIENTED_EDGE('',*,*,#6544,.T.);
#8720=ORIENTED_EDGE('',*,*,#6457,.T.);
#8721=ORIENTED_EDGE('',*,*,#6544,.F.);
#8722=ORIENTED_EDGE('',*,*,#6462,.T.);
#8723=ORIENTED_EDGE('',*,*,#6545,.F.);
#8724=ORIENTED_EDGE('',*,*,#6546,.F.);
#8725=ORIENTED_EDGE('',*,*,#6547,.T.);
#8726=ORIENTED_EDGE('',*,*,#6548,.F.);
#8727=ORIENTED_EDGE('',*,*,#6547,.F.);
#8728=ORIENTED_EDGE('',*,*,#6546,.T.);
#8729=ORIENTED_EDGE('',*,*,#6454,.T.);
#8730=ORIENTED_EDGE('',*,*,#6545,.T.);
#8731=ORIENTED_EDGE('',*,*,#6461,.T.);
#8732=ORIENTED_EDGE('',*,*,#6458,.T.);
#8733=ORIENTED_EDGE('',*,*,#6549,.F.);
#8734=ORIENTED_EDGE('',*,*,#6550,.F.);
#8735=ORIENTED_EDGE('',*,*,#6551,.F.);
#8736=ORIENTED_EDGE('',*,*,#6541,.F.);
#8737=ORIENTED_EDGE('',*,*,#6551,.T.);
#8738=ORIENTED_EDGE('',*,*,#6552,.F.);
#8739=ORIENTED_EDGE('',*,*,#6553,.F.);
#8740=ORIENTED_EDGE('',*,*,#6542,.F.);
#8741=ORIENTED_EDGE('',*,*,#6553,.T.);
#8742=ORIENTED_EDGE('',*,*,#6554,.F.);
#8743=ORIENTED_EDGE('',*,*,#6555,.F.);
#8744=ORIENTED_EDGE('',*,*,#6543,.F.);
#8745=ORIENTED_EDGE('',*,*,#6555,.T.);
#8746=ORIENTED_EDGE('',*,*,#6556,.F.);
#8747=ORIENTED_EDGE('',*,*,#6557,.T.);
#8748=ORIENTED_EDGE('',*,*,#6464,.F.);
#8749=ORIENTED_EDGE('',*,*,#6557,.F.);
#8750=ORIENTED_EDGE('',*,*,#6558,.F.);
#8751=ORIENTED_EDGE('',*,*,#6559,.F.);
#8752=ORIENTED_EDGE('',*,*,#6465,.F.);
#8753=ORIENTED_EDGE('',*,*,#6559,.T.);
#8754=ORIENTED_EDGE('',*,*,#6560,.F.);
#8755=ORIENTED_EDGE('',*,*,#6561,.F.);
#8756=ORIENTED_EDGE('',*,*,#6466,.F.);
#8757=ORIENTED_EDGE('',*,*,#6561,.T.);
#8758=ORIENTED_EDGE('',*,*,#6562,.F.);
#8759=ORIENTED_EDGE('',*,*,#6563,.F.);
#8760=ORIENTED_EDGE('',*,*,#6467,.F.);
#8761=ORIENTED_EDGE('',*,*,#6563,.T.);
#8762=ORIENTED_EDGE('',*,*,#6564,.F.);
#8763=ORIENTED_EDGE('',*,*,#6565,.T.);
#8764=ORIENTED_EDGE('',*,*,#6468,.F.);
#8765=ORIENTED_EDGE('',*,*,#6565,.F.);
#8766=ORIENTED_EDGE('',*,*,#6566,.F.);
#8767=ORIENTED_EDGE('',*,*,#6567,.F.);
#8768=ORIENTED_EDGE('',*,*,#6469,.F.);
#8769=ORIENTED_EDGE('',*,*,#6567,.T.);
#8770=ORIENTED_EDGE('',*,*,#6568,.F.);
#8771=ORIENTED_EDGE('',*,*,#6569,.F.);
#8772=ORIENTED_EDGE('',*,*,#6470,.F.);
#8773=ORIENTED_EDGE('',*,*,#6569,.T.);
#8774=ORIENTED_EDGE('',*,*,#6570,.F.);
#8775=ORIENTED_EDGE('',*,*,#6571,.F.);
#8776=ORIENTED_EDGE('',*,*,#6471,.F.);
#8777=ORIENTED_EDGE('',*,*,#6571,.T.);
#8778=ORIENTED_EDGE('',*,*,#6572,.F.);
#8779=ORIENTED_EDGE('',*,*,#6573,.T.);
#8780=ORIENTED_EDGE('',*,*,#6472,.F.);
#8781=ORIENTED_EDGE('',*,*,#6573,.F.);
#8782=ORIENTED_EDGE('',*,*,#6574,.F.);
#8783=ORIENTED_EDGE('',*,*,#6575,.F.);
#8784=ORIENTED_EDGE('',*,*,#6473,.F.);
#8785=ORIENTED_EDGE('',*,*,#6575,.T.);
#8786=ORIENTED_EDGE('',*,*,#6576,.F.);
#8787=ORIENTED_EDGE('',*,*,#6577,.F.);
#8788=ORIENTED_EDGE('',*,*,#6474,.F.);
#8789=ORIENTED_EDGE('',*,*,#6577,.T.);
#8790=ORIENTED_EDGE('',*,*,#6578,.F.);
#8791=ORIENTED_EDGE('',*,*,#6579,.F.);
#8792=ORIENTED_EDGE('',*,*,#6475,.F.);
#8793=ORIENTED_EDGE('',*,*,#6579,.T.);
#8794=ORIENTED_EDGE('',*,*,#6580,.F.);
#8795=ORIENTED_EDGE('',*,*,#6581,.T.);
#8796=ORIENTED_EDGE('',*,*,#6476,.F.);
#8797=ORIENTED_EDGE('',*,*,#6581,.F.);
#8798=ORIENTED_EDGE('',*,*,#6582,.F.);
#8799=ORIENTED_EDGE('',*,*,#6583,.F.);
#8800=ORIENTED_EDGE('',*,*,#6477,.F.);
#8801=ORIENTED_EDGE('',*,*,#6583,.T.);
#8802=ORIENTED_EDGE('',*,*,#6584,.F.);
#8803=ORIENTED_EDGE('',*,*,#6585,.F.);
#8804=ORIENTED_EDGE('',*,*,#6478,.F.);
#8805=ORIENTED_EDGE('',*,*,#6585,.T.);
#8806=ORIENTED_EDGE('',*,*,#6586,.F.);
#8807=ORIENTED_EDGE('',*,*,#6587,.F.);
#8808=ORIENTED_EDGE('',*,*,#6479,.F.);
#8809=ORIENTED_EDGE('',*,*,#6587,.T.);
#8810=ORIENTED_EDGE('',*,*,#6588,.F.);
#8811=ORIENTED_EDGE('',*,*,#6589,.T.);
#8812=ORIENTED_EDGE('',*,*,#6480,.F.);
#8813=ORIENTED_EDGE('',*,*,#6589,.F.);
#8814=ORIENTED_EDGE('',*,*,#6590,.F.);
#8815=ORIENTED_EDGE('',*,*,#6591,.F.);
#8816=ORIENTED_EDGE('',*,*,#6481,.F.);
#8817=ORIENTED_EDGE('',*,*,#6591,.T.);
#8818=ORIENTED_EDGE('',*,*,#6592,.F.);
#8819=ORIENTED_EDGE('',*,*,#6593,.F.);
#8820=ORIENTED_EDGE('',*,*,#6482,.F.);
#8821=ORIENTED_EDGE('',*,*,#6593,.T.);
#8822=ORIENTED_EDGE('',*,*,#6594,.F.);
#8823=ORIENTED_EDGE('',*,*,#6595,.F.);
#8824=ORIENTED_EDGE('',*,*,#6483,.F.);
#8825=ORIENTED_EDGE('',*,*,#6595,.T.);
#8826=ORIENTED_EDGE('',*,*,#6596,.F.);
#8827=ORIENTED_EDGE('',*,*,#6597,.T.);
#8828=ORIENTED_EDGE('',*,*,#6484,.F.);
#8829=ORIENTED_EDGE('',*,*,#6597,.F.);
#8830=ORIENTED_EDGE('',*,*,#6598,.F.);
#8831=ORIENTED_EDGE('',*,*,#6599,.F.);
#8832=ORIENTED_EDGE('',*,*,#6485,.F.);
#8833=ORIENTED_EDGE('',*,*,#6599,.T.);
#8834=ORIENTED_EDGE('',*,*,#6600,.F.);
#8835=ORIENTED_EDGE('',*,*,#6601,.F.);
#8836=ORIENTED_EDGE('',*,*,#6486,.F.);
#8837=ORIENTED_EDGE('',*,*,#6601,.T.);
#8838=ORIENTED_EDGE('',*,*,#6602,.F.);
#8839=ORIENTED_EDGE('',*,*,#6603,.F.);
#8840=ORIENTED_EDGE('',*,*,#6487,.F.);
#8841=ORIENTED_EDGE('',*,*,#6603,.T.);
#8842=ORIENTED_EDGE('',*,*,#6604,.F.);
#8843=ORIENTED_EDGE('',*,*,#6605,.T.);
#8844=ORIENTED_EDGE('',*,*,#6488,.F.);
#8845=ORIENTED_EDGE('',*,*,#6605,.F.);
#8846=ORIENTED_EDGE('',*,*,#6606,.F.);
#8847=ORIENTED_EDGE('',*,*,#6607,.F.);
#8848=ORIENTED_EDGE('',*,*,#6489,.F.);
#8849=ORIENTED_EDGE('',*,*,#6607,.T.);
#8850=ORIENTED_EDGE('',*,*,#6608,.F.);
#8851=ORIENTED_EDGE('',*,*,#6609,.F.);
#8852=ORIENTED_EDGE('',*,*,#6490,.F.);
#8853=ORIENTED_EDGE('',*,*,#6609,.T.);
#8854=ORIENTED_EDGE('',*,*,#6610,.F.);
#8855=ORIENTED_EDGE('',*,*,#6611,.F.);
#8856=ORIENTED_EDGE('',*,*,#6491,.F.);
#8857=ORIENTED_EDGE('',*,*,#6611,.T.);
#8858=ORIENTED_EDGE('',*,*,#6612,.F.);
#8859=ORIENTED_EDGE('',*,*,#6613,.T.);
#8860=ORIENTED_EDGE('',*,*,#6492,.F.);
#8861=ORIENTED_EDGE('',*,*,#6613,.F.);
#8862=ORIENTED_EDGE('',*,*,#6614,.F.);
#8863=ORIENTED_EDGE('',*,*,#6615,.F.);
#8864=ORIENTED_EDGE('',*,*,#6493,.F.);
#8865=ORIENTED_EDGE('',*,*,#6615,.T.);
#8866=ORIENTED_EDGE('',*,*,#6616,.F.);
#8867=ORIENTED_EDGE('',*,*,#6617,.F.);
#8868=ORIENTED_EDGE('',*,*,#6494,.F.);
#8869=ORIENTED_EDGE('',*,*,#6617,.T.);
#8870=ORIENTED_EDGE('',*,*,#6618,.F.);
#8871=ORIENTED_EDGE('',*,*,#6619,.F.);
#8872=ORIENTED_EDGE('',*,*,#6495,.F.);
#8873=ORIENTED_EDGE('',*,*,#6619,.T.);
#8874=ORIENTED_EDGE('',*,*,#6620,.F.);
#8875=ORIENTED_EDGE('',*,*,#6621,.T.);
#8876=ORIENTED_EDGE('',*,*,#6496,.F.);
#8877=ORIENTED_EDGE('',*,*,#6621,.F.);
#8878=ORIENTED_EDGE('',*,*,#6622,.F.);
#8879=ORIENTED_EDGE('',*,*,#6623,.F.);
#8880=ORIENTED_EDGE('',*,*,#6497,.F.);
#8881=ORIENTED_EDGE('',*,*,#6623,.T.);
#8882=ORIENTED_EDGE('',*,*,#6624,.F.);
#8883=ORIENTED_EDGE('',*,*,#6625,.F.);
#8884=ORIENTED_EDGE('',*,*,#6498,.F.);
#8885=ORIENTED_EDGE('',*,*,#6625,.T.);
#8886=ORIENTED_EDGE('',*,*,#6626,.F.);
#8887=ORIENTED_EDGE('',*,*,#6627,.F.);
#8888=ORIENTED_EDGE('',*,*,#6499,.F.);
#8889=ORIENTED_EDGE('',*,*,#6627,.T.);
#8890=ORIENTED_EDGE('',*,*,#6628,.F.);
#8891=ORIENTED_EDGE('',*,*,#6629,.T.);
#8892=ORIENTED_EDGE('',*,*,#6500,.F.);
#8893=ORIENTED_EDGE('',*,*,#6629,.F.);
#8894=ORIENTED_EDGE('',*,*,#6630,.F.);
#8895=ORIENTED_EDGE('',*,*,#6631,.F.);
#8896=ORIENTED_EDGE('',*,*,#6501,.F.);
#8897=ORIENTED_EDGE('',*,*,#6631,.T.);
#8898=ORIENTED_EDGE('',*,*,#6632,.F.);
#8899=ORIENTED_EDGE('',*,*,#6633,.F.);
#8900=ORIENTED_EDGE('',*,*,#6502,.F.);
#8901=ORIENTED_EDGE('',*,*,#6633,.T.);
#8902=ORIENTED_EDGE('',*,*,#6634,.F.);
#8903=ORIENTED_EDGE('',*,*,#6635,.F.);
#8904=ORIENTED_EDGE('',*,*,#6503,.F.);
#8905=ORIENTED_EDGE('',*,*,#6635,.T.);
#8906=ORIENTED_EDGE('',*,*,#6636,.F.);
#8907=ORIENTED_EDGE('',*,*,#6637,.T.);
#8908=ORIENTED_EDGE('',*,*,#6504,.F.);
#8909=ORIENTED_EDGE('',*,*,#6637,.F.);
#8910=ORIENTED_EDGE('',*,*,#6638,.F.);
#8911=ORIENTED_EDGE('',*,*,#6639,.F.);
#8912=ORIENTED_EDGE('',*,*,#6505,.F.);
#8913=ORIENTED_EDGE('',*,*,#6639,.T.);
#8914=ORIENTED_EDGE('',*,*,#6640,.F.);
#8915=ORIENTED_EDGE('',*,*,#6641,.F.);
#8916=ORIENTED_EDGE('',*,*,#6506,.F.);
#8917=ORIENTED_EDGE('',*,*,#6641,.T.);
#8918=ORIENTED_EDGE('',*,*,#6642,.F.);
#8919=ORIENTED_EDGE('',*,*,#6643,.F.);
#8920=ORIENTED_EDGE('',*,*,#6507,.F.);
#8921=ORIENTED_EDGE('',*,*,#6643,.T.);
#8922=ORIENTED_EDGE('',*,*,#6644,.F.);
#8923=ORIENTED_EDGE('',*,*,#6645,.T.);
#8924=ORIENTED_EDGE('',*,*,#6508,.F.);
#8925=ORIENTED_EDGE('',*,*,#6645,.F.);
#8926=ORIENTED_EDGE('',*,*,#6646,.F.);
#8927=ORIENTED_EDGE('',*,*,#6647,.F.);
#8928=ORIENTED_EDGE('',*,*,#6509,.F.);
#8929=ORIENTED_EDGE('',*,*,#6647,.T.);
#8930=ORIENTED_EDGE('',*,*,#6648,.F.);
#8931=ORIENTED_EDGE('',*,*,#6649,.F.);
#8932=ORIENTED_EDGE('',*,*,#6510,.F.);
#8933=ORIENTED_EDGE('',*,*,#6649,.T.);
#8934=ORIENTED_EDGE('',*,*,#6650,.F.);
#8935=ORIENTED_EDGE('',*,*,#6651,.F.);
#8936=ORIENTED_EDGE('',*,*,#6511,.F.);
#8937=ORIENTED_EDGE('',*,*,#6651,.T.);
#8938=ORIENTED_EDGE('',*,*,#6652,.F.);
#8939=ORIENTED_EDGE('',*,*,#6653,.T.);
#8940=ORIENTED_EDGE('',*,*,#6512,.F.);
#8941=ORIENTED_EDGE('',*,*,#6653,.F.);
#8942=ORIENTED_EDGE('',*,*,#6654,.F.);
#8943=ORIENTED_EDGE('',*,*,#6655,.F.);
#8944=ORIENTED_EDGE('',*,*,#6513,.F.);
#8945=ORIENTED_EDGE('',*,*,#6655,.T.);
#8946=ORIENTED_EDGE('',*,*,#6656,.F.);
#8947=ORIENTED_EDGE('',*,*,#6657,.F.);
#8948=ORIENTED_EDGE('',*,*,#6514,.F.);
#8949=ORIENTED_EDGE('',*,*,#6657,.T.);
#8950=ORIENTED_EDGE('',*,*,#6658,.F.);
#8951=ORIENTED_EDGE('',*,*,#6659,.F.);
#8952=ORIENTED_EDGE('',*,*,#6515,.F.);
#8953=ORIENTED_EDGE('',*,*,#6659,.T.);
#8954=ORIENTED_EDGE('',*,*,#6660,.F.);
#8955=ORIENTED_EDGE('',*,*,#6661,.T.);
#8956=ORIENTED_EDGE('',*,*,#6516,.F.);
#8957=ORIENTED_EDGE('',*,*,#6661,.F.);
#8958=ORIENTED_EDGE('',*,*,#6662,.F.);
#8959=ORIENTED_EDGE('',*,*,#6663,.F.);
#8960=ORIENTED_EDGE('',*,*,#6517,.F.);
#8961=ORIENTED_EDGE('',*,*,#6663,.T.);
#8962=ORIENTED_EDGE('',*,*,#6664,.F.);
#8963=ORIENTED_EDGE('',*,*,#6665,.F.);
#8964=ORIENTED_EDGE('',*,*,#6518,.F.);
#8965=ORIENTED_EDGE('',*,*,#6665,.T.);
#8966=ORIENTED_EDGE('',*,*,#6666,.F.);
#8967=ORIENTED_EDGE('',*,*,#6667,.F.);
#8968=ORIENTED_EDGE('',*,*,#6519,.F.);
#8969=ORIENTED_EDGE('',*,*,#6667,.T.);
#8970=ORIENTED_EDGE('',*,*,#6668,.F.);
#8971=ORIENTED_EDGE('',*,*,#6669,.T.);
#8972=ORIENTED_EDGE('',*,*,#6520,.F.);
#8973=ORIENTED_EDGE('',*,*,#6669,.F.);
#8974=ORIENTED_EDGE('',*,*,#6670,.F.);
#8975=ORIENTED_EDGE('',*,*,#6671,.F.);
#8976=ORIENTED_EDGE('',*,*,#6521,.F.);
#8977=ORIENTED_EDGE('',*,*,#6671,.T.);
#8978=ORIENTED_EDGE('',*,*,#6672,.F.);
#8979=ORIENTED_EDGE('',*,*,#6673,.F.);
#8980=ORIENTED_EDGE('',*,*,#6522,.F.);
#8981=ORIENTED_EDGE('',*,*,#6673,.T.);
#8982=ORIENTED_EDGE('',*,*,#6674,.F.);
#8983=ORIENTED_EDGE('',*,*,#6675,.F.);
#8984=ORIENTED_EDGE('',*,*,#6523,.F.);
#8985=ORIENTED_EDGE('',*,*,#6675,.T.);
#8986=ORIENTED_EDGE('',*,*,#6676,.F.);
#8987=ORIENTED_EDGE('',*,*,#6677,.T.);
#8988=ORIENTED_EDGE('',*,*,#6524,.F.);
#8989=ORIENTED_EDGE('',*,*,#6677,.F.);
#8990=ORIENTED_EDGE('',*,*,#6678,.F.);
#8991=ORIENTED_EDGE('',*,*,#6679,.F.);
#8992=ORIENTED_EDGE('',*,*,#6525,.F.);
#8993=ORIENTED_EDGE('',*,*,#6679,.T.);
#8994=ORIENTED_EDGE('',*,*,#6680,.F.);
#8995=ORIENTED_EDGE('',*,*,#6681,.F.);
#8996=ORIENTED_EDGE('',*,*,#6526,.F.);
#8997=ORIENTED_EDGE('',*,*,#6681,.T.);
#8998=ORIENTED_EDGE('',*,*,#6682,.F.);
#8999=ORIENTED_EDGE('',*,*,#6683,.F.);
#9000=ORIENTED_EDGE('',*,*,#6527,.F.);
#9001=ORIENTED_EDGE('',*,*,#6683,.T.);
#9002=ORIENTED_EDGE('',*,*,#6684,.F.);
#9003=ORIENTED_EDGE('',*,*,#6685,.T.);
#9004=ORIENTED_EDGE('',*,*,#6528,.F.);
#9005=ORIENTED_EDGE('',*,*,#6685,.F.);
#9006=ORIENTED_EDGE('',*,*,#6686,.F.);
#9007=ORIENTED_EDGE('',*,*,#6687,.F.);
#9008=ORIENTED_EDGE('',*,*,#6529,.F.);
#9009=ORIENTED_EDGE('',*,*,#6687,.T.);
#9010=ORIENTED_EDGE('',*,*,#6688,.F.);
#9011=ORIENTED_EDGE('',*,*,#6689,.F.);
#9012=ORIENTED_EDGE('',*,*,#6530,.F.);
#9013=ORIENTED_EDGE('',*,*,#6689,.T.);
#9014=ORIENTED_EDGE('',*,*,#6690,.F.);
#9015=ORIENTED_EDGE('',*,*,#6691,.F.);
#9016=ORIENTED_EDGE('',*,*,#6531,.F.);
#9017=ORIENTED_EDGE('',*,*,#6691,.T.);
#9018=ORIENTED_EDGE('',*,*,#6692,.F.);
#9019=ORIENTED_EDGE('',*,*,#6693,.T.);
#9020=ORIENTED_EDGE('',*,*,#6532,.F.);
#9021=ORIENTED_EDGE('',*,*,#6693,.F.);
#9022=ORIENTED_EDGE('',*,*,#6694,.F.);
#9023=ORIENTED_EDGE('',*,*,#6695,.F.);
#9024=ORIENTED_EDGE('',*,*,#6533,.F.);
#9025=ORIENTED_EDGE('',*,*,#6695,.T.);
#9026=ORIENTED_EDGE('',*,*,#6696,.F.);
#9027=ORIENTED_EDGE('',*,*,#6697,.F.);
#9028=ORIENTED_EDGE('',*,*,#6534,.F.);
#9029=ORIENTED_EDGE('',*,*,#6697,.T.);
#9030=ORIENTED_EDGE('',*,*,#6698,.F.);
#9031=ORIENTED_EDGE('',*,*,#6699,.F.);
#9032=ORIENTED_EDGE('',*,*,#6535,.F.);
#9033=ORIENTED_EDGE('',*,*,#6699,.T.);
#9034=ORIENTED_EDGE('',*,*,#6700,.F.);
#9035=ORIENTED_EDGE('',*,*,#6701,.T.);
#9036=ORIENTED_EDGE('',*,*,#6536,.F.);
#9037=ORIENTED_EDGE('',*,*,#6701,.F.);
#9038=ORIENTED_EDGE('',*,*,#6702,.F.);
#9039=ORIENTED_EDGE('',*,*,#6703,.F.);
#9040=ORIENTED_EDGE('',*,*,#6537,.F.);
#9041=ORIENTED_EDGE('',*,*,#6703,.T.);
#9042=ORIENTED_EDGE('',*,*,#6704,.F.);
#9043=ORIENTED_EDGE('',*,*,#6705,.F.);
#9044=ORIENTED_EDGE('',*,*,#6538,.F.);
#9045=ORIENTED_EDGE('',*,*,#6705,.T.);
#9046=ORIENTED_EDGE('',*,*,#6706,.F.);
#9047=ORIENTED_EDGE('',*,*,#6707,.F.);
#9048=ORIENTED_EDGE('',*,*,#6539,.F.);
#9049=ORIENTED_EDGE('',*,*,#6708,.T.);
#9050=ORIENTED_EDGE('',*,*,#6706,.T.);
#9051=ORIENTED_EDGE('',*,*,#6704,.T.);
#9052=ORIENTED_EDGE('',*,*,#6702,.T.);
#9053=ORIENTED_EDGE('',*,*,#6700,.T.);
#9054=ORIENTED_EDGE('',*,*,#6698,.T.);
#9055=ORIENTED_EDGE('',*,*,#6696,.T.);
#9056=ORIENTED_EDGE('',*,*,#6694,.T.);
#9057=ORIENTED_EDGE('',*,*,#6692,.T.);
#9058=ORIENTED_EDGE('',*,*,#6690,.T.);
#9059=ORIENTED_EDGE('',*,*,#6688,.T.);
#9060=ORIENTED_EDGE('',*,*,#6686,.T.);
#9061=ORIENTED_EDGE('',*,*,#6684,.T.);
#9062=ORIENTED_EDGE('',*,*,#6682,.T.);
#9063=ORIENTED_EDGE('',*,*,#6680,.T.);
#9064=ORIENTED_EDGE('',*,*,#6678,.T.);
#9065=ORIENTED_EDGE('',*,*,#6676,.T.);
#9066=ORIENTED_EDGE('',*,*,#6674,.T.);
#9067=ORIENTED_EDGE('',*,*,#6672,.T.);
#9068=ORIENTED_EDGE('',*,*,#6670,.T.);
#9069=ORIENTED_EDGE('',*,*,#6668,.T.);
#9070=ORIENTED_EDGE('',*,*,#6666,.T.);
#9071=ORIENTED_EDGE('',*,*,#6664,.T.);
#9072=ORIENTED_EDGE('',*,*,#6662,.T.);
#9073=ORIENTED_EDGE('',*,*,#6660,.T.);
#9074=ORIENTED_EDGE('',*,*,#6658,.T.);
#9075=ORIENTED_EDGE('',*,*,#6656,.T.);
#9076=ORIENTED_EDGE('',*,*,#6654,.T.);
#9077=ORIENTED_EDGE('',*,*,#6652,.T.);
#9078=ORIENTED_EDGE('',*,*,#6650,.T.);
#9079=ORIENTED_EDGE('',*,*,#6648,.T.);
#9080=ORIENTED_EDGE('',*,*,#6646,.T.);
#9081=ORIENTED_EDGE('',*,*,#6644,.T.);
#9082=ORIENTED_EDGE('',*,*,#6642,.T.);
#9083=ORIENTED_EDGE('',*,*,#6640,.T.);
#9084=ORIENTED_EDGE('',*,*,#6638,.T.);
#9085=ORIENTED_EDGE('',*,*,#6636,.T.);
#9086=ORIENTED_EDGE('',*,*,#6634,.T.);
#9087=ORIENTED_EDGE('',*,*,#6632,.T.);
#9088=ORIENTED_EDGE('',*,*,#6630,.T.);
#9089=ORIENTED_EDGE('',*,*,#6628,.T.);
#9090=ORIENTED_EDGE('',*,*,#6626,.T.);
#9091=ORIENTED_EDGE('',*,*,#6624,.T.);
#9092=ORIENTED_EDGE('',*,*,#6622,.T.);
#9093=ORIENTED_EDGE('',*,*,#6620,.T.);
#9094=ORIENTED_EDGE('',*,*,#6618,.T.);
#9095=ORIENTED_EDGE('',*,*,#6616,.T.);
#9096=ORIENTED_EDGE('',*,*,#6614,.T.);
#9097=ORIENTED_EDGE('',*,*,#6612,.T.);
#9098=ORIENTED_EDGE('',*,*,#6610,.T.);
#9099=ORIENTED_EDGE('',*,*,#6608,.T.);
#9100=ORIENTED_EDGE('',*,*,#6606,.T.);
#9101=ORIENTED_EDGE('',*,*,#6604,.T.);
#9102=ORIENTED_EDGE('',*,*,#6602,.T.);
#9103=ORIENTED_EDGE('',*,*,#6600,.T.);
#9104=ORIENTED_EDGE('',*,*,#6598,.T.);
#9105=ORIENTED_EDGE('',*,*,#6596,.T.);
#9106=ORIENTED_EDGE('',*,*,#6594,.T.);
#9107=ORIENTED_EDGE('',*,*,#6592,.T.);
#9108=ORIENTED_EDGE('',*,*,#6590,.T.);
#9109=ORIENTED_EDGE('',*,*,#6588,.T.);
#9110=ORIENTED_EDGE('',*,*,#6586,.T.);
#9111=ORIENTED_EDGE('',*,*,#6584,.T.);
#9112=ORIENTED_EDGE('',*,*,#6582,.T.);
#9113=ORIENTED_EDGE('',*,*,#6580,.T.);
#9114=ORIENTED_EDGE('',*,*,#6578,.T.);
#9115=ORIENTED_EDGE('',*,*,#6576,.T.);
#9116=ORIENTED_EDGE('',*,*,#6574,.T.);
#9117=ORIENTED_EDGE('',*,*,#6572,.T.);
#9118=ORIENTED_EDGE('',*,*,#6570,.T.);
#9119=ORIENTED_EDGE('',*,*,#6568,.T.);
#9120=ORIENTED_EDGE('',*,*,#6566,.T.);
#9121=ORIENTED_EDGE('',*,*,#6564,.T.);
#9122=ORIENTED_EDGE('',*,*,#6562,.T.);
#9123=ORIENTED_EDGE('',*,*,#6560,.T.);
#9124=ORIENTED_EDGE('',*,*,#6558,.T.);
#9125=ORIENTED_EDGE('',*,*,#6556,.T.);
#9126=ORIENTED_EDGE('',*,*,#6554,.T.);
#9127=ORIENTED_EDGE('',*,*,#6552,.T.);
#9128=ORIENTED_EDGE('',*,*,#6550,.T.);
#9129=ORIENTED_EDGE('',*,*,#6548,.T.);
#9130=ORIENTED_EDGE('',*,*,#6549,.T.);
#9131=ORIENTED_EDGE('',*,*,#6540,.F.);
#9132=ORIENTED_EDGE('',*,*,#6707,.T.);
#9133=ORIENTED_EDGE('',*,*,#6708,.F.);
#10541=CYLINDRICAL_SURFACE('',#12586,0.6);
#10542=CYLINDRICAL_SURFACE('',#12588,1.4);
#10543=CYLINDRICAL_SURFACE('',#12593,1.75);
#10544=CYLINDRICAL_SURFACE('',#12596,1.75);
#10545=CYLINDRICAL_SURFACE('',#12599,1.75);
#10546=CYLINDRICAL_SURFACE('',#12602,1.75);
#10547=CYLINDRICAL_SURFACE('',#12605,1.75);
#10548=CYLINDRICAL_SURFACE('',#12608,1.75);
#10549=CYLINDRICAL_SURFACE('',#12611,1.75);
#10550=CYLINDRICAL_SURFACE('',#12614,1.75);
#10551=CYLINDRICAL_SURFACE('',#12617,1.75);
#10552=CYLINDRICAL_SURFACE('',#12620,1.75);
#10553=CYLINDRICAL_SURFACE('',#12623,1.75);
#10554=CYLINDRICAL_SURFACE('',#12626,1.75);
#10555=CYLINDRICAL_SURFACE('',#12629,1.75);
#10556=CYLINDRICAL_SURFACE('',#12632,1.75);
#10557=CYLINDRICAL_SURFACE('',#12635,1.75);
#10558=CYLINDRICAL_SURFACE('',#12638,1.75);
#10559=CYLINDRICAL_SURFACE('',#12641,1.75);
#10560=CYLINDRICAL_SURFACE('',#12644,1.75);
#10561=CYLINDRICAL_SURFACE('',#12647,1.75);
#10562=CYLINDRICAL_SURFACE('',#12652,1.75);
#10941=ADVANCED_FACE('',(#1821),#1381,.F.);
#10942=ADVANCED_FACE('',(#1822),#1382,.F.);
#10943=ADVANCED_FACE('',(#1823),#1383,.F.);
#10944=ADVANCED_FACE('',(#1824,#1214),#1384,.F.);
#10945=ADVANCED_FACE('',(#1825),#10541,.F.);
#10946=ADVANCED_FACE('',(#1826),#10542,.T.);
#10947=ADVANCED_FACE('',(#1827,#1215),#1385,.T.);
#10948=ADVANCED_FACE('',(#1828),#11,.T.);
#10949=ADVANCED_FACE('',(#1829),#1386,.T.);
#10950=ADVANCED_FACE('',(#1830),#12,.T.);
#10951=ADVANCED_FACE('',(#1831),#10543,.T.);
#10952=ADVANCED_FACE('',(#1832),#13,.T.);
#10953=ADVANCED_FACE('',(#1833),#1387,.T.);
#10954=ADVANCED_FACE('',(#1834),#14,.T.);
#10955=ADVANCED_FACE('',(#1835),#10544,.T.);
#10956=ADVANCED_FACE('',(#1836),#15,.T.);
#10957=ADVANCED_FACE('',(#1837),#1388,.T.);
#10958=ADVANCED_FACE('',(#1838),#16,.T.);
#10959=ADVANCED_FACE('',(#1839),#10545,.T.);
#10960=ADVANCED_FACE('',(#1840),#17,.T.);
#10961=ADVANCED_FACE('',(#1841),#1389,.T.);
#10962=ADVANCED_FACE('',(#1842),#18,.T.);
#10963=ADVANCED_FACE('',(#1843),#10546,.T.);
#10964=ADVANCED_FACE('',(#1844),#19,.T.);
#10965=ADVANCED_FACE('',(#1845),#1390,.T.);
#10966=ADVANCED_FACE('',(#1846),#20,.T.);
#10967=ADVANCED_FACE('',(#1847),#10547,.T.);
#10968=ADVANCED_FACE('',(#1848),#21,.T.);
#10969=ADVANCED_FACE('',(#1849),#1391,.T.);
#10970=ADVANCED_FACE('',(#1850),#22,.T.);
#10971=ADVANCED_FACE('',(#1851),#10548,.T.);
#10972=ADVANCED_FACE('',(#1852),#23,.T.);
#10973=ADVANCED_FACE('',(#1853),#1392,.T.);
#10974=ADVANCED_FACE('',(#1854),#24,.T.);
#10975=ADVANCED_FACE('',(#1855),#10549,.T.);
#10976=ADVANCED_FACE('',(#1856),#25,.T.);
#10977=ADVANCED_FACE('',(#1857),#1393,.T.);
#10978=ADVANCED_FACE('',(#1858),#26,.T.);
#10979=ADVANCED_FACE('',(#1859),#10550,.T.);
#10980=ADVANCED_FACE('',(#1860),#27,.T.);
#10981=ADVANCED_FACE('',(#1861),#1394,.T.);
#10982=ADVANCED_FACE('',(#1862),#28,.T.);
#10983=ADVANCED_FACE('',(#1863),#10551,.T.);
#10984=ADVANCED_FACE('',(#1864),#29,.T.);
#10985=ADVANCED_FACE('',(#1865),#1395,.T.);
#10986=ADVANCED_FACE('',(#1866),#30,.T.);
#10987=ADVANCED_FACE('',(#1867),#10552,.T.);
#10988=ADVANCED_FACE('',(#1868),#31,.T.);
#10989=ADVANCED_FACE('',(#1869),#1396,.T.);
#10990=ADVANCED_FACE('',(#1870),#32,.T.);
#10991=ADVANCED_FACE('',(#1871),#10553,.T.);
#10992=ADVANCED_FACE('',(#1872),#33,.T.);
#10993=ADVANCED_FACE('',(#1873),#1397,.T.);
#10994=ADVANCED_FACE('',(#1874),#34,.T.);
#10995=ADVANCED_FACE('',(#1875),#10554,.T.);
#10996=ADVANCED_FACE('',(#1876),#35,.T.);
#10997=ADVANCED_FACE('',(#1877),#1398,.T.);
#10998=ADVANCED_FACE('',(#1878),#36,.T.);
#10999=ADVANCED_FACE('',(#1879),#10555,.T.);
#11000=ADVANCED_FACE('',(#1880),#37,.T.);
#11001=ADVANCED_FACE('',(#1881),#1399,.T.);
#11002=ADVANCED_FACE('',(#1882),#38,.T.);
#11003=ADVANCED_FACE('',(#1883),#10556,.T.);
#11004=ADVANCED_FACE('',(#1884),#39,.T.);
#11005=ADVANCED_FACE('',(#1885),#1400,.T.);
#11006=ADVANCED_FACE('',(#1886),#40,.T.);
#11007=ADVANCED_FACE('',(#1887),#10557,.T.);
#11008=ADVANCED_FACE('',(#1888),#41,.T.);
#11009=ADVANCED_FACE('',(#1889),#1401,.T.);
#11010=ADVANCED_FACE('',(#1890),#42,.T.);
#11011=ADVANCED_FACE('',(#1891),#10558,.T.);
#11012=ADVANCED_FACE('',(#1892),#43,.T.);
#11013=ADVANCED_FACE('',(#1893),#1402,.T.);
#11014=ADVANCED_FACE('',(#1894),#44,.T.);
#11015=ADVANCED_FACE('',(#1895),#10559,.T.);
#11016=ADVANCED_FACE('',(#1896),#45,.T.);
#11017=ADVANCED_FACE('',(#1897),#1403,.T.);
#11018=ADVANCED_FACE('',(#1898),#46,.T.);
#11019=ADVANCED_FACE('',(#1899),#10560,.T.);
#11020=ADVANCED_FACE('',(#1900),#47,.T.);
#11021=ADVANCED_FACE('',(#1901),#1404,.T.);
#11022=ADVANCED_FACE('',(#1902),#48,.T.);
#11023=ADVANCED_FACE('',(#1903),#10561,.T.);
#11024=ADVANCED_FACE('',(#1904),#49,.T.);
#11025=ADVANCED_FACE('',(#1905),#1405,.T.);
#11026=ADVANCED_FACE('',(#1906),#50,.T.);
#11027=ADVANCED_FACE('',(#1907,#1216),#1406,.T.);
#11028=ADVANCED_FACE('',(#1908),#10562,.T.);
#11320=CLOSED_SHELL('',(#10941,#10942,#10943,#10944,#10945,#10946,#10947,
#10948,#10949,#10950,#10951,#10952,#10953,#10954,#10955,#10956,#10957,#10958,
#10959,#10960,#10961,#10962,#10963,#10964,#10965,#10966,#10967,#10968,#10969,
#10970,#10971,#10972,#10973,#10974,#10975,#10976,#10977,#10978,#10979,#10980,
#10981,#10982,#10983,#10984,#10985,#10986,#10987,#10988,#10989,#10990,#10991,
#10992,#10993,#10994,#10995,#10996,#10997,#10998,#10999,#11000,#11001,#11002,
#11003,#11004,#11005,#11006,#11007,#11008,#11009,#11010,#11011,#11012,#11013,
#11014,#11015,#11016,#11017,#11018,#11019,#11020,#11021,#11022,#11023,#11024,
#11025,#11026,#11027,#11028));
#12560=AXIS2_PLACEMENT_3D('',#18188,#14735,#14736);
#12561=AXIS2_PLACEMENT_3D('',#18189,#14737,#14738);
#12562=AXIS2_PLACEMENT_3D('',#18198,#14743,#14744);
#12563=AXIS2_PLACEMENT_3D('',#18204,#14748,#14749);
#12564=AXIS2_PLACEMENT_3D('',#18210,#14753,#14754);
#12565=AXIS2_PLACEMENT_3D('',#18213,#14755,#14756);
#12566=AXIS2_PLACEMENT_3D('',#18359,#14758,#14759);
#12567=AXIS2_PLACEMENT_3D('',#18505,#14761,#14762);
#12568=AXIS2_PLACEMENT_3D('',#18651,#14764,#14765);
#12569=AXIS2_PLACEMENT_3D('',#18797,#14767,#14768);
#12570=AXIS2_PLACEMENT_3D('',#18943,#14770,#14771);
#12571=AXIS2_PLACEMENT_3D('',#19089,#14773,#14774);
#12572=AXIS2_PLACEMENT_3D('',#19235,#14776,#14777);
#12573=AXIS2_PLACEMENT_3D('',#19381,#14779,#14780);
#12574=AXIS2_PLACEMENT_3D('',#19527,#14782,#14783);
#12575=AXIS2_PLACEMENT_3D('',#19673,#14785,#14786);
#12576=AXIS2_PLACEMENT_3D('',#19819,#14788,#14789);
#12577=AXIS2_PLACEMENT_3D('',#19965,#14791,#14792);
#12578=AXIS2_PLACEMENT_3D('',#20111,#14794,#14795);
#12579=AXIS2_PLACEMENT_3D('',#20257,#14797,#14798);
#12580=AXIS2_PLACEMENT_3D('',#20403,#14800,#14801);
#12581=AXIS2_PLACEMENT_3D('',#20549,#14803,#14804);
#12582=AXIS2_PLACEMENT_3D('',#20695,#14806,#14807);
#12583=AXIS2_PLACEMENT_3D('',#20841,#14809,#14810);
#12584=AXIS2_PLACEMENT_3D('',#20987,#14812,#14813);
#12585=AXIS2_PLACEMENT_3D('',#21131,#14815,#14816);
#12586=AXIS2_PLACEMENT_3D('',#21132,#14817,#14818);
#12587=AXIS2_PLACEMENT_3D('',#21133,#14819,#14820);
#12588=AXIS2_PLACEMENT_3D('',#21134,#14821,#14822);
#12589=AXIS2_PLACEMENT_3D('',#21136,#14823,#14824);
#12590=AXIS2_PLACEMENT_3D('',#21139,#14826,#14827);
#12591=AXIS2_PLACEMENT_3D('',#21140,#14828,#14829);
#12592=AXIS2_PLACEMENT_3D('',#21355,#14832,#14833);
#12593=AXIS2_PLACEMENT_3D('',#21571,#14837,#14838);
#12594=AXIS2_PLACEMENT_3D('',#21573,#14839,#14840);
#12595=AXIS2_PLACEMENT_3D('',#21787,#14843,#14844);
#12596=AXIS2_PLACEMENT_3D('',#22003,#14848,#14849);
#12597=AXIS2_PLACEMENT_3D('',#22005,#14850,#14851);
#12598=AXIS2_PLACEMENT_3D('',#22219,#14854,#14855);
#12599=AXIS2_PLACEMENT_3D('',#22435,#14859,#14860);
#12600=AXIS2_PLACEMENT_3D('',#22437,#14861,#14862);
#12601=AXIS2_PLACEMENT_3D('',#22651,#14865,#14866);
#12602=AXIS2_PLACEMENT_3D('',#22867,#14870,#14871);
#12603=AXIS2_PLACEMENT_3D('',#22869,#14872,#14873);
#12604=AXIS2_PLACEMENT_3D('',#23083,#14876,#14877);
#12605=AXIS2_PLACEMENT_3D('',#23299,#14881,#14882);
#12606=AXIS2_PLACEMENT_3D('',#23301,#14883,#14884);
#12607=AXIS2_PLACEMENT_3D('',#23515,#14887,#14888);
#12608=AXIS2_PLACEMENT_3D('',#23731,#14892,#14893);
#12609=AXIS2_PLACEMENT_3D('',#23733,#14894,#14895);
#12610=AXIS2_PLACEMENT_3D('',#23947,#14898,#14899);
#12611=AXIS2_PLACEMENT_3D('',#24163,#14903,#14904);
#12612=AXIS2_PLACEMENT_3D('',#24165,#14905,#14906);
#12613=AXIS2_PLACEMENT_3D('',#24379,#14909,#14910);
#12614=AXIS2_PLACEMENT_3D('',#24595,#14914,#14915);
#12615=AXIS2_PLACEMENT_3D('',#24597,#14916,#14917);
#12616=AXIS2_PLACEMENT_3D('',#24811,#14920,#14921);
#12617=AXIS2_PLACEMENT_3D('',#25027,#14925,#14926);
#12618=AXIS2_PLACEMENT_3D('',#25029,#14927,#14928);
#12619=AXIS2_PLACEMENT_3D('',#25243,#14931,#14932);
#12620=AXIS2_PLACEMENT_3D('',#25459,#14936,#14937);
#12621=AXIS2_PLACEMENT_3D('',#25461,#14938,#14939);
#12622=AXIS2_PLACEMENT_3D('',#25675,#14942,#14943);
#12623=AXIS2_PLACEMENT_3D('',#25891,#14947,#14948);
#12624=AXIS2_PLACEMENT_3D('',#25893,#14949,#14950);
#12625=AXIS2_PLACEMENT_3D('',#26107,#14953,#14954);
#12626=AXIS2_PLACEMENT_3D('',#26323,#14958,#14959);
#12627=AXIS2_PLACEMENT_3D('',#26325,#14960,#14961);
#12628=AXIS2_PLACEMENT_3D('',#26539,#14964,#14965);
#12629=AXIS2_PLACEMENT_3D('',#26755,#14969,#14970);
#12630=AXIS2_PLACEMENT_3D('',#26757,#14971,#14972);
#12631=AXIS2_PLACEMENT_3D('',#26971,#14975,#14976);
#12632=AXIS2_PLACEMENT_3D('',#27187,#14980,#14981);
#12633=AXIS2_PLACEMENT_3D('',#27189,#14982,#14983);
#12634=AXIS2_PLACEMENT_3D('',#27403,#14986,#14987);
#12635=AXIS2_PLACEMENT_3D('',#27619,#14991,#14992);
#12636=AXIS2_PLACEMENT_3D('',#27621,#14993,#14994);
#12637=AXIS2_PLACEMENT_3D('',#27835,#14997,#14998);
#12638=AXIS2_PLACEMENT_3D('',#28051,#15002,#15003);
#12639=AXIS2_PLACEMENT_3D('',#28053,#15004,#15005);
#12640=AXIS2_PLACEMENT_3D('',#28267,#15008,#15009);
#12641=AXIS2_PLACEMENT_3D('',#28483,#15013,#15014);
#12642=AXIS2_PLACEMENT_3D('',#28485,#15015,#15016);
#12643=AXIS2_PLACEMENT_3D('',#28699,#15019,#15020);
#12644=AXIS2_PLACEMENT_3D('',#28915,#15024,#15025);
#12645=AXIS2_PLACEMENT_3D('',#28917,#15026,#15027);
#12646=AXIS2_PLACEMENT_3D('',#29131,#15030,#15031);
#12647=AXIS2_PLACEMENT_3D('',#29347,#15035,#15036);
#12648=AXIS2_PLACEMENT_3D('',#29349,#15037,#15038);
#12649=AXIS2_PLACEMENT_3D('',#29563,#15041,#15042);
#12650=AXIS2_PLACEMENT_3D('',#29779,#15046,#15047);
#12651=AXIS2_PLACEMENT_3D('',#29780,#15048,#15049);
#12652=AXIS2_PLACEMENT_3D('',#29781,#15050,#15051);
#14735=DIRECTION('axis',(0.,0.,1.));
#14736=DIRECTION('refdir',(1.,0.,0.));
#14737=DIRECTION('center_axis',(1.,0.,0.));
#14738=DIRECTION('ref_axis',(0.,0.,-1.));
#14739=DIRECTION('',(0.,0.,1.));
#14740=DIRECTION('',(0.,1.,0.));
#14741=DIRECTION('',(0.,0.,-1.));
#14742=DIRECTION('',(0.,-1.,0.));
#14743=DIRECTION('center_axis',(0.,0.,-1.));
#14744=DIRECTION('ref_axis',(-1.,0.,0.));
#14745=DIRECTION('',(1.,0.,0.));
#14746=DIRECTION('',(0.,-1.,0.));
#14747=DIRECTION('',(-1.,0.,0.));
#14748=DIRECTION('center_axis',(-1.,0.,0.));
#14749=DIRECTION('ref_axis',(0.,0.,1.));
#14750=DIRECTION('',(0.,0.,-1.));
#14751=DIRECTION('',(0.,1.,0.));
#14752=DIRECTION('',(0.,0.,1.));
#14753=DIRECTION('center_axis',(0.,1.,0.));
#14754=DIRECTION('ref_axis',(1.,0.,0.));
#14755=DIRECTION('center_axis',(0.,-1.,0.));
#14756=DIRECTION('ref_axis',(1.,0.,0.));
#14757=DIRECTION('',(-0.587785252292473,0.,0.809016994374947));
#14758=DIRECTION('center_axis',(0.,-1.,0.));
#14759=DIRECTION('ref_axis',(1.,0.,0.));
#14760=DIRECTION('',(-0.809016994374948,0.,0.587785252292473));
#14761=DIRECTION('center_axis',(0.,-1.,0.));
#14762=DIRECTION('ref_axis',(1.,0.,0.));
#14763=DIRECTION('',(-0.951056516295154,0.,0.309016994374947));
#14764=DIRECTION('center_axis',(0.,-1.,0.));
#14765=DIRECTION('ref_axis',(1.,0.,0.));
#14766=DIRECTION('',(-1.,0.,-1.83697019872103E-16));
#14767=DIRECTION('center_axis',(0.,-1.,0.));
#14768=DIRECTION('ref_axis',(1.,0.,0.));
#14769=DIRECTION('',(-0.951056516295154,0.,-0.309016994374948));
#14770=DIRECTION('center_axis',(0.,-1.,0.));
#14771=DIRECTION('ref_axis',(1.,0.,0.));
#14772=DIRECTION('',(-0.809016994374947,0.,-0.587785252292473));
#14773=DIRECTION('center_axis',(0.,-1.,0.));
#14774=DIRECTION('ref_axis',(1.,0.,0.));
#14775=DIRECTION('',(-0.587785252292473,0.,-0.809016994374948));
#14776=DIRECTION('center_axis',(0.,-1.,0.));
#14777=DIRECTION('ref_axis',(1.,0.,0.));
#14778=DIRECTION('',(-0.309016994374947,0.,-0.951056516295154));
#14779=DIRECTION('center_axis',(0.,-1.,0.));
#14780=DIRECTION('ref_axis',(1.,0.,0.));
#14781=DIRECTION('',(1.22464679914735E-16,0.,-1.));
#14782=DIRECTION('center_axis',(0.,-1.,0.));
#14783=DIRECTION('ref_axis',(1.,0.,0.));
#14784=DIRECTION('',(0.309016994374948,0.,-0.951056516295154));
#14785=DIRECTION('center_axis',(0.,-1.,0.));
#14786=DIRECTION('ref_axis',(1.,0.,0.));
#14787=DIRECTION('',(0.587785252292473,0.,-0.809016994374947));
#14788=DIRECTION('center_axis',(0.,-1.,0.));
#14789=DIRECTION('ref_axis',(1.,0.,0.));
#14790=DIRECTION('',(0.809016994374948,0.,-0.587785252292473));
#14791=DIRECTION('center_axis',(0.,-1.,0.));
#14792=DIRECTION('ref_axis',(1.,0.,0.));
#14793=DIRECTION('',(0.951056516295154,0.,-0.309016994374947));
#14794=DIRECTION('center_axis',(0.,-1.,0.));
#14795=DIRECTION('ref_axis',(1.,0.,0.));
#14796=DIRECTION('',(1.,0.,6.12323399573677E-17));
#14797=DIRECTION('center_axis',(0.,-1.,0.));
#14798=DIRECTION('ref_axis',(1.,0.,0.));
#14799=DIRECTION('',(0.951056516295154,0.,0.309016994374948));
#14800=DIRECTION('center_axis',(0.,-1.,0.));
#14801=DIRECTION('ref_axis',(1.,0.,0.));
#14802=DIRECTION('',(0.809016994374947,0.,0.587785252292473));
#14803=DIRECTION('center_axis',(0.,-1.,0.));
#14804=DIRECTION('ref_axis',(1.,0.,0.));
#14805=DIRECTION('',(0.587785252292473,0.,0.809016994374947));
#14806=DIRECTION('center_axis',(0.,-1.,0.));
#14807=DIRECTION('ref_axis',(1.,0.,0.));
#14808=DIRECTION('',(0.309016994374947,0.,0.951056516295154));
#14809=DIRECTION('center_axis',(0.,-1.,0.));
#14810=DIRECTION('ref_axis',(1.,0.,0.));
#14811=DIRECTION('',(0.,0.,1.));
#14812=DIRECTION('center_axis',(0.,-1.,0.));
#14813=DIRECTION('ref_axis',(1.,0.,0.));
#14814=DIRECTION('',(-0.309016994374948,0.,0.951056516295154));
#14815=DIRECTION('center_axis',(0.,1.,0.));
#14816=DIRECTION('ref_axis',(1.,0.,0.));
#14817=DIRECTION('center_axis',(0.,1.,0.));
#14818=DIRECTION('ref_axis',(6.12323399573677E-17,0.,1.));
#14819=DIRECTION('center_axis',(0.,-1.,0.));
#14820=DIRECTION('ref_axis',(1.,0.,0.));
#14821=DIRECTION('center_axis',(0.,1.,0.));
#14822=DIRECTION('ref_axis',(1.,0.,0.));
#14823=DIRECTION('center_axis',(0.,1.,0.));
#14824=DIRECTION('ref_axis',(1.,0.,0.));
#14825=DIRECTION('',(0.,-1.,0.));
#14826=DIRECTION('center_axis',(0.,-1.,0.));
#14827=DIRECTION('ref_axis',(1.,0.,0.));
#14828=DIRECTION('center_axis',(0.,1.,0.));
#14829=DIRECTION('ref_axis',(1.,0.,0.));
#14830=DIRECTION('',(0.,-1.,0.));
#14831=DIRECTION('',(0.,1.,0.));
#14832=DIRECTION('center_axis',(0.951056516295154,0.,0.309016994374948));
#14833=DIRECTION('ref_axis',(0.309016994374948,0.,-0.951056516295154));
#14834=DIRECTION('',(0.309016994374948,0.,-0.951056516295154));
#14835=DIRECTION('',(0.,1.,0.));
#14836=DIRECTION('',(0.,1.,0.));
#14837=DIRECTION('center_axis',(0.,1.,0.));
#14838=DIRECTION('ref_axis',(1.,0.,0.));
#14839=DIRECTION('center_axis',(0.,1.,0.));
#14840=DIRECTION('ref_axis',(1.,0.,0.));
#14841=DIRECTION('',(0.,-1.,0.));
#14842=DIRECTION('',(0.,1.,0.));
#14843=DIRECTION('center_axis',(0.809016994374947,0.,0.587785252292473));
#14844=DIRECTION('ref_axis',(0.587785252292473,0.,-0.809016994374947));
#14845=DIRECTION('',(0.587785252292473,0.,-0.809016994374947));
#14846=DIRECTION('',(0.,1.,0.));
#14847=DIRECTION('',(0.,1.,0.));
#14848=DIRECTION('center_axis',(0.,1.,0.));
#14849=DIRECTION('ref_axis',(1.,0.,0.));
#14850=DIRECTION('center_axis',(0.,1.,0.));
#14851=DIRECTION('ref_axis',(1.,0.,0.));
#14852=DIRECTION('',(0.,-1.,0.));
#14853=DIRECTION('',(0.,1.,0.));
#14854=DIRECTION('center_axis',(0.587785252292473,0.,0.809016994374948));
#14855=DIRECTION('ref_axis',(0.809016994374948,0.,-0.587785252292473));
#14856=DIRECTION('',(0.809016994374948,0.,-0.587785252292473));
#14857=DIRECTION('',(0.,1.,0.));
#14858=DIRECTION('',(0.,1.,0.));
#14859=DIRECTION('center_axis',(0.,1.,0.));
#14860=DIRECTION('ref_axis',(1.,0.,0.));
#14861=DIRECTION('center_axis',(0.,1.,0.));
#14862=DIRECTION('ref_axis',(1.,0.,0.));
#14863=DIRECTION('',(0.,-1.,0.));
#14864=DIRECTION('',(0.,1.,0.));
#14865=DIRECTION('center_axis',(0.309016994374947,0.,0.951056516295154));
#14866=DIRECTION('ref_axis',(0.951056516295154,0.,-0.309016994374947));
#14867=DIRECTION('',(0.951056516295154,0.,-0.309016994374947));
#14868=DIRECTION('',(0.,1.,0.));
#14869=DIRECTION('',(0.,1.,0.));
#14870=DIRECTION('center_axis',(0.,1.,0.));
#14871=DIRECTION('ref_axis',(1.,0.,0.));
#14872=DIRECTION('center_axis',(0.,1.,0.));
#14873=DIRECTION('ref_axis',(1.,0.,0.));
#14874=DIRECTION('',(0.,-1.,0.));
#14875=DIRECTION('',(0.,1.,0.));
#14876=DIRECTION('center_axis',(-1.83697019872103E-16,0.,1.));
#14877=DIRECTION('ref_axis',(1.,0.,1.83697019872103E-16));
#14878=DIRECTION('',(1.,0.,1.83697019872103E-16));
#14879=DIRECTION('',(0.,1.,0.));
#14880=DIRECTION('',(0.,1.,0.));
#14881=DIRECTION('center_axis',(0.,1.,0.));
#14882=DIRECTION('ref_axis',(1.,0.,0.));
#14883=DIRECTION('center_axis',(0.,1.,0.));
#14884=DIRECTION('ref_axis',(1.,0.,0.));
#14885=DIRECTION('',(0.,-1.,0.));
#14886=DIRECTION('',(0.,1.,0.));
#14887=DIRECTION('center_axis',(-0.309016994374948,0.,0.951056516295154));
#14888=DIRECTION('ref_axis',(0.951056516295154,0.,0.309016994374948));
#14889=DIRECTION('',(0.951056516295154,0.,0.309016994374948));
#14890=DIRECTION('',(0.,1.,0.));
#14891=DIRECTION('',(0.,1.,0.));
#14892=DIRECTION('center_axis',(0.,1.,0.));
#14893=DIRECTION('ref_axis',(1.,0.,0.));
#14894=DIRECTION('center_axis',(0.,1.,0.));
#14895=DIRECTION('ref_axis',(1.,0.,0.));
#14896=DIRECTION('',(0.,-1.,0.));
#14897=DIRECTION('',(0.,1.,0.));
#14898=DIRECTION('center_axis',(-0.587785252292473,0.,0.809016994374947));
#14899=DIRECTION('ref_axis',(0.809016994374947,0.,0.587785252292473));
#14900=DIRECTION('',(0.809016994374947,0.,0.587785252292473));
#14901=DIRECTION('',(0.,1.,0.));
#14902=DIRECTION('',(0.,1.,0.));
#14903=DIRECTION('center_axis',(0.,1.,0.));
#14904=DIRECTION('ref_axis',(1.,0.,0.));
#14905=DIRECTION('center_axis',(0.,1.,0.));
#14906=DIRECTION('ref_axis',(1.,0.,0.));
#14907=DIRECTION('',(0.,-1.,0.));
#14908=DIRECTION('',(0.,1.,0.));
#14909=DIRECTION('center_axis',(-0.809016994374948,0.,0.587785252292473));
#14910=DIRECTION('ref_axis',(0.587785252292473,0.,0.809016994374948));
#14911=DIRECTION('',(0.587785252292473,0.,0.809016994374948));
#14912=DIRECTION('',(0.,1.,0.));
#14913=DIRECTION('',(0.,1.,0.));
#14914=DIRECTION('center_axis',(0.,1.,0.));
#14915=DIRECTION('ref_axis',(1.,0.,0.));
#14916=DIRECTION('center_axis',(0.,1.,0.));
#14917=DIRECTION('ref_axis',(1.,0.,0.));
#14918=DIRECTION('',(0.,-1.,0.));
#14919=DIRECTION('',(0.,1.,0.));
#14920=DIRECTION('center_axis',(-0.951056516295154,0.,0.309016994374947));
#14921=DIRECTION('ref_axis',(0.309016994374947,0.,0.951056516295154));
#14922=DIRECTION('',(0.309016994374947,0.,0.951056516295154));
#14923=DIRECTION('',(0.,1.,0.));
#14924=DIRECTION('',(0.,1.,0.));
#14925=DIRECTION('center_axis',(0.,1.,0.));
#14926=DIRECTION('ref_axis',(1.,0.,0.));
#14927=DIRECTION('center_axis',(0.,1.,0.));
#14928=DIRECTION('ref_axis',(1.,0.,0.));
#14929=DIRECTION('',(0.,-1.,0.));
#14930=DIRECTION('',(0.,1.,0.));
#14931=DIRECTION('center_axis',(-1.,0.,-1.22464679914735E-16));
#14932=DIRECTION('ref_axis',(-1.22464679914735E-16,0.,1.));
#14933=DIRECTION('',(-1.22464679914735E-16,0.,1.));
#14934=DIRECTION('',(0.,1.,0.));
#14935=DIRECTION('',(0.,1.,0.));
#14936=DIRECTION('center_axis',(0.,1.,0.));
#14937=DIRECTION('ref_axis',(1.,0.,0.));
#14938=DIRECTION('center_axis',(0.,1.,0.));
#14939=DIRECTION('ref_axis',(1.,0.,0.));
#14940=DIRECTION('',(0.,-1.,0.));
#14941=DIRECTION('',(0.,1.,0.));
#14942=DIRECTION('center_axis',(-0.951056516295154,0.,-0.309016994374948));
#14943=DIRECTION('ref_axis',(-0.309016994374948,0.,0.951056516295154));
#14944=DIRECTION('',(-0.309016994374948,0.,0.951056516295154));
#14945=DIRECTION('',(0.,1.,0.));
#14946=DIRECTION('',(0.,1.,0.));
#14947=DIRECTION('center_axis',(0.,1.,0.));
#14948=DIRECTION('ref_axis',(1.,0.,0.));
#14949=DIRECTION('center_axis',(0.,1.,0.));
#14950=DIRECTION('ref_axis',(1.,0.,0.));
#14951=DIRECTION('',(0.,-1.,0.));
#14952=DIRECTION('',(0.,1.,0.));
#14953=DIRECTION('center_axis',(-0.809016994374947,0.,-0.587785252292473));
#14954=DIRECTION('ref_axis',(-0.587785252292473,0.,0.809016994374947));
#14955=DIRECTION('',(-0.587785252292473,0.,0.809016994374947));
#14956=DIRECTION('',(0.,1.,0.));
#14957=DIRECTION('',(0.,1.,0.));
#14958=DIRECTION('center_axis',(0.,1.,0.));
#14959=DIRECTION('ref_axis',(1.,0.,0.));
#14960=DIRECTION('center_axis',(0.,1.,0.));
#14961=DIRECTION('ref_axis',(1.,0.,0.));
#14962=DIRECTION('',(0.,-1.,0.));
#14963=DIRECTION('',(0.,1.,0.));
#14964=DIRECTION('center_axis',(-0.587785252292473,0.,-0.809016994374948));
#14965=DIRECTION('ref_axis',(-0.809016994374948,0.,0.587785252292473));
#14966=DIRECTION('',(-0.809016994374948,0.,0.587785252292473));
#14967=DIRECTION('',(0.,1.,0.));
#14968=DIRECTION('',(0.,1.,0.));
#14969=DIRECTION('center_axis',(0.,1.,0.));
#14970=DIRECTION('ref_axis',(1.,0.,0.));
#14971=DIRECTION('center_axis',(0.,1.,0.));
#14972=DIRECTION('ref_axis',(1.,0.,0.));
#14973=DIRECTION('',(0.,-1.,0.));
#14974=DIRECTION('',(0.,1.,0.));
#14975=DIRECTION('center_axis',(-0.309016994374947,0.,-0.951056516295154));
#14976=DIRECTION('ref_axis',(-0.951056516295154,0.,0.309016994374947));
#14977=DIRECTION('',(-0.951056516295154,0.,0.309016994374947));
#14978=DIRECTION('',(0.,1.,0.));
#14979=DIRECTION('',(0.,1.,0.));
#14980=DIRECTION('center_axis',(0.,1.,0.));
#14981=DIRECTION('ref_axis',(1.,0.,0.));
#14982=DIRECTION('center_axis',(0.,1.,0.));
#14983=DIRECTION('ref_axis',(1.,0.,0.));
#14984=DIRECTION('',(0.,-1.,0.));
#14985=DIRECTION('',(0.,1.,0.));
#14986=DIRECTION('center_axis',(6.12323399573677E-17,0.,-1.));
#14987=DIRECTION('ref_axis',(-1.,0.,-6.12323399573677E-17));
#14988=DIRECTION('',(-1.,0.,-6.12323399573677E-17));
#14989=DIRECTION('',(0.,1.,0.));
#14990=DIRECTION('',(0.,1.,0.));
#14991=DIRECTION('center_axis',(0.,1.,0.));
#14992=DIRECTION('ref_axis',(1.,0.,0.));
#14993=DIRECTION('center_axis',(0.,1.,0.));
#14994=DIRECTION('ref_axis',(1.,0.,0.));
#14995=DIRECTION('',(0.,-1.,0.));
#14996=DIRECTION('',(0.,1.,0.));
#14997=DIRECTION('center_axis',(0.309016994374948,0.,-0.951056516295154));
#14998=DIRECTION('ref_axis',(-0.951056516295154,0.,-0.309016994374948));
#14999=DIRECTION('',(-0.951056516295154,0.,-0.309016994374948));
#15000=DIRECTION('',(0.,1.,0.));
#15001=DIRECTION('',(0.,1.,0.));
#15002=DIRECTION('center_axis',(0.,1.,0.));
#15003=DIRECTION('ref_axis',(1.,0.,0.));
#15004=DIRECTION('center_axis',(0.,1.,0.));
#15005=DIRECTION('ref_axis',(1.,0.,0.));
#15006=DIRECTION('',(0.,-1.,0.));
#15007=DIRECTION('',(0.,1.,0.));
#15008=DIRECTION('center_axis',(0.587785252292473,0.,-0.809016994374947));
#15009=DIRECTION('ref_axis',(-0.809016994374947,0.,-0.587785252292473));
#15010=DIRECTION('',(-0.809016994374947,0.,-0.587785252292473));
#15011=DIRECTION('',(0.,1.,0.));
#15012=DIRECTION('',(0.,1.,0.));
#15013=DIRECTION('center_axis',(0.,1.,0.));
#15014=DIRECTION('ref_axis',(1.,0.,0.));
#15015=DIRECTION('center_axis',(0.,1.,0.));
#15016=DIRECTION('ref_axis',(1.,0.,0.));
#15017=DIRECTION('',(0.,-1.,0.));
#15018=DIRECTION('',(0.,1.,0.));
#15019=DIRECTION('center_axis',(0.809016994374947,0.,-0.587785252292473));
#15020=DIRECTION('ref_axis',(-0.587785252292473,0.,-0.809016994374947));
#15021=DIRECTION('',(-0.587785252292473,0.,-0.809016994374947));
#15022=DIRECTION('',(0.,1.,0.));
#15023=DIRECTION('',(0.,1.,0.));
#15024=DIRECTION('center_axis',(0.,1.,0.));
#15025=DIRECTION('ref_axis',(1.,0.,0.));
#15026=DIRECTION('center_axis',(0.,1.,0.));
#15027=DIRECTION('ref_axis',(1.,0.,0.));
#15028=DIRECTION('',(0.,-1.,0.));
#15029=DIRECTION('',(0.,1.,0.));
#15030=DIRECTION('center_axis',(0.951056516295154,0.,-0.309016994374947));
#15031=DIRECTION('ref_axis',(-0.309016994374947,0.,-0.951056516295154));
#15032=DIRECTION('',(-0.309016994374947,0.,-0.951056516295154));
#15033=DIRECTION('',(0.,1.,0.));
#15034=DIRECTION('',(0.,1.,0.));
#15035=DIRECTION('center_axis',(0.,1.,0.));
#15036=DIRECTION('ref_axis',(1.,0.,0.));
#15037=DIRECTION('center_axis',(0.,1.,0.));
#15038=DIRECTION('ref_axis',(1.,0.,0.));
#15039=DIRECTION('',(0.,-1.,0.));
#15040=DIRECTION('',(0.,1.,0.));
#15041=DIRECTION('center_axis',(1.,0.,0.));
#15042=DIRECTION('ref_axis',(0.,0.,-1.));
#15043=DIRECTION('',(0.,0.,-1.));
#15044=DIRECTION('',(0.,1.,0.));
#15045=DIRECTION('',(0.,1.,0.));
#15046=DIRECTION('center_axis',(0.,1.,0.));
#15047=DIRECTION('ref_axis',(1.,0.,0.));
#15048=DIRECTION('center_axis',(0.,1.,0.));
#15049=DIRECTION('ref_axis',(1.,0.,0.));
#15050=DIRECTION('center_axis',(0.,1.,0.));
#15051=DIRECTION('ref_axis',(1.,0.,0.));
#18188=CARTESIAN_POINT('',(0.,0.,0.));
#18189=CARTESIAN_POINT('Origin',(0.2,0.,0.));
#18190=CARTESIAN_POINT('',(0.2,2.2,-0.78));
#18191=CARTESIAN_POINT('',(0.2,2.2,-0.565685424949238));
#18192=CARTESIAN_POINT('',(0.2,2.2,0.));
#18193=CARTESIAN_POINT('',(0.2,-1.,-0.78));
#18194=CARTESIAN_POINT('',(0.2,0.,-0.78));
#18195=CARTESIAN_POINT('',(0.2,-1.,-0.565685424949238));
#18196=CARTESIAN_POINT('',(0.2,-1.,0.));
#18197=CARTESIAN_POINT('',(0.2,0.,-0.565685424949238));
#18198=CARTESIAN_POINT('Origin',(0.2,0.,-0.78));
#18199=CARTESIAN_POINT('',(-0.2,2.2,-0.78));
#18200=CARTESIAN_POINT('',(0.1,2.2,-0.78));
#18201=CARTESIAN_POINT('',(-0.2,-1.,-0.78));
#18202=CARTESIAN_POINT('',(-0.2,0.,-0.78));
#18203=CARTESIAN_POINT('',(0.1,-1.,-0.78));
#18204=CARTESIAN_POINT('Origin',(-0.2,0.,-0.78));
#18205=CARTESIAN_POINT('',(-0.2,2.2,-0.565685424949238));
#18206=CARTESIAN_POINT('',(-0.2,2.2,-0.39));
#18207=CARTESIAN_POINT('',(-0.2,-1.,-0.565685424949238));
#18208=CARTESIAN_POINT('',(-0.2,0.,-0.565685424949238));
#18209=CARTESIAN_POINT('',(-0.2,-1.,-0.39));
#18210=CARTESIAN_POINT('Origin',(0.,-1.,0.));
#18211=CARTESIAN_POINT('',(1.60662857109684,-1.,0.693717979106306));
#18212=CARTESIAN_POINT('',(1.5055822144029,-1.,0.892032620296856));
#18213=CARTESIAN_POINT('Origin',(0.,-1.,0.));
#18214=CARTESIAN_POINT('',(1.81978687191668,-1.,1.23627494547115));
#18215=CARTESIAN_POINT('Ctrl Pts',(1.5055822144029,-1.,0.892032620296856));
#18216=CARTESIAN_POINT('Ctrl Pts',(1.50980486806688,-1.,0.894452006964544));
#18217=CARTESIAN_POINT('Ctrl Pts',(1.51805569590094,-1.,0.899185047483511));
#18218=CARTESIAN_POINT('Ctrl Pts',(1.52984849887993,-1.,0.905967409625651));
#18219=CARTESIAN_POINT('Ctrl Pts',(1.54440491149498,-1.,0.914375919026456));
#18220=CARTESIAN_POINT('Ctrl Pts',(1.56065988578893,-1.,0.923832188944341));
#18221=CARTESIAN_POINT('Ctrl Pts',(1.57499388382243,-1.,0.932246680108685));
#18222=CARTESIAN_POINT('Ctrl Pts',(1.58744937487176,-1.,0.939646377893399));
#18223=CARTESIAN_POINT('Ctrl Pts',(1.59810042043673,-1.,0.946078063315257));
#18224=CARTESIAN_POINT('Ctrl Pts',(1.60706069896936,-1.,0.951613284356035));
#18225=CARTESIAN_POINT('Ctrl Pts',(1.61449324337085,-1.,0.956354422920671));
#18226=CARTESIAN_POINT('Ctrl Pts',(1.62061638140221,-1.,0.960438326101729));
#18227=CARTESIAN_POINT('Ctrl Pts',(1.62571930670187,-1.,0.964046107040536));
#18228=CARTESIAN_POINT('Ctrl Pts',(1.63013849959461,-1.,0.967387853230345));
#18229=CARTESIAN_POINT('Ctrl Pts',(1.63420665729798,-1.,0.970669715997509));
#18230=CARTESIAN_POINT('Ctrl Pts',(1.63820952658144,-1.,0.974066058287419));
#18231=CARTESIAN_POINT('Ctrl Pts',(1.64233990826687,-1.,0.977689794119417));
#18232=CARTESIAN_POINT('Ctrl Pts',(1.64665139190656,-1.,0.981562530939489));
#18233=CARTESIAN_POINT('Ctrl Pts',(1.65110016612638,-1.,0.985642622920821));
#18234=CARTESIAN_POINT('Ctrl Pts',(1.65559044289699,-1.,0.989855627854165));
#18235=CARTESIAN_POINT('Ctrl Pts',(1.66001553809947,-1.,0.994121836661306));
#18236=CARTESIAN_POINT('Ctrl Pts',(1.66430758030376,-1.,0.998389654952758));
#18237=CARTESIAN_POINT('Ctrl Pts',(1.66846059277303,-1.,1.00265091003727));
#18238=CARTESIAN_POINT('Ctrl Pts',(1.67250335383293,-1.,1.00692206696414));
#18239=CARTESIAN_POINT('Ctrl Pts',(1.67648246776464,-1.,1.01123236493511));
#18240=CARTESIAN_POINT('Ctrl Pts',(1.68044289894798,-1.,1.01561026162773));
#18241=CARTESIAN_POINT('Ctrl Pts',(1.68440578021706,-1.,1.02006795074201));
#18242=CARTESIAN_POINT('Ctrl Pts',(1.68836910178447,-1.,1.02460180535255));
#18243=CARTESIAN_POINT('Ctrl Pts',(1.69231840863458,-1.,1.02919977579147));
#18244=CARTESIAN_POINT('Ctrl Pts',(1.69623414782771,-1.,1.03384646003588));
#18245=CARTESIAN_POINT('Ctrl Pts',(1.70010052930962,-1.,1.03852922490789));
#18246=CARTESIAN_POINT('Ctrl Pts',(1.70391338707982,-1.,1.04324363334554));
#18247=CARTESIAN_POINT('Ctrl Pts',(1.70767646263649,-1.,1.04799085404995));
#18248=CARTESIAN_POINT('Ctrl Pts',(1.71139783543989,-1.,1.05277517202855));
#18249=CARTESIAN_POINT('Ctrl Pts',(1.7150865442702,-1.,1.05760163192479));
#18250=CARTESIAN_POINT('Ctrl Pts',(1.71874858456904,-1.,1.06247324680647));
#18251=CARTESIAN_POINT('Ctrl Pts',(1.72238500928453,-1.,1.06738966975462));
#18252=CARTESIAN_POINT('Ctrl Pts',(1.72599406198488,-1.,1.07234866990252));
#18253=CARTESIAN_POINT('Ctrl Pts',(1.72957248977424,-1.,1.0773470373727));
#18254=CARTESIAN_POINT('Ctrl Pts',(1.73311705663407,-1.,1.08238162784749));
#18255=CARTESIAN_POINT('Ctrl Pts',(1.73662628326091,-1.,1.08745056285427));
#18256=CARTESIAN_POINT('Ctrl Pts',(1.74010053962247,-1.,1.09255329056493));
#18257=CARTESIAN_POINT('Ctrl Pts',(1.74354119236208,-1.,1.09768999241226));
#18258=CARTESIAN_POINT('Ctrl Pts',(1.74695004214923,-1.,1.10286118991143));
#18259=CARTESIAN_POINT('Ctrl Pts',(1.7503286607592,-1.,1.10806728183007));
#18260=CARTESIAN_POINT('Ctrl Pts',(1.7536777209463,-1.,1.11330807582551));
#18261=CARTESIAN_POINT('Ctrl Pts',(1.75699720772105,-1.,1.11858293216763));
#18262=CARTESIAN_POINT('Ctrl Pts',(1.76028671825096,-1.,1.12389096855086));
#18263=CARTESIAN_POINT('Ctrl Pts',(1.7635457196617,-1.,1.12923123555075));
#18264=CARTESIAN_POINT('Ctrl Pts',(1.76677384551862,-1.,1.1346029180462));
#18265=CARTESIAN_POINT('Ctrl Pts',(1.76997111386769,-1.,1.14000548336975));
#18266=CARTESIAN_POINT('Ctrl Pts',(1.77313777896194,-1.,1.1454385822692));
#18267=CARTESIAN_POINT('Ctrl Pts',(1.7762742255701,-1.,1.15090197841515));
#18268=CARTESIAN_POINT('Ctrl Pts',(1.77938085564275,-1.,1.15639547194698));
#18269=CARTESIAN_POINT('Ctrl Pts',(1.78245795881009,-1.,1.16191881298499));
#18270=CARTESIAN_POINT('Ctrl Pts',(1.78550566040443,-1.,1.16747166312303));
#18271=CARTESIAN_POINT('Ctrl Pts',(1.78852398877616,-1.,1.17305363177328));
#18272=CARTESIAN_POINT('Ctrl Pts',(1.79151291552689,-1.,1.17866429440809));
#18273=CARTESIAN_POINT('Ctrl Pts',(1.79447240321515,-1.,1.18430321697432));
#18274=CARTESIAN_POINT('Ctrl Pts',(1.79740245923478,-1.,1.18996997934445));
#18275=CARTESIAN_POINT('Ctrl Pts',(1.80030314369879,-1.,1.19566418930242));
#18276=CARTESIAN_POINT('Ctrl Pts',(1.80317454838603,-1.,1.20138548938974));
#18277=CARTESIAN_POINT('Ctrl Pts',(1.80601678480707,-1.,1.20713356605475));
#18278=CARTESIAN_POINT('Ctrl Pts',(1.80882996917129,-1.,1.21290815708314));
#18279=CARTESIAN_POINT('Ctrl Pts',(1.81161420806656,-1.,1.21870906103557));
#18280=CARTESIAN_POINT('Ctrl Pts',(1.81436959210434,-1.,1.2245361330495));
#18281=CARTESIAN_POINT('Ctrl Pts',(1.8165508718364,-1.,1.2292186489137));
#18282=CARTESIAN_POINT('Ctrl Pts',(1.81817389921279,-1.,1.2327422452705));
#18283=CARTESIAN_POINT('Ctrl Pts',(1.81925017193666,-1.,1.23509651170476));
#18284=CARTESIAN_POINT('Ctrl Pts',(1.81978687191668,-1.,1.23627494547115));
#18285=CARTESIAN_POINT('',(1.73811241238545,-1.,1.34869019493419));
#18286=CARTESIAN_POINT('',(1.81978687191668,-1.,1.23627494547115));
#18287=CARTESIAN_POINT('',(1.31362392696032,-1.,1.15624053661742));
#18288=CARTESIAN_POINT('Ctrl Pts',(1.73811241238545,-1.,1.34869019493419));
#18289=CARTESIAN_POINT('Ctrl Pts',(1.73682580585691,-1.,1.34854391898045));
#18290=CARTESIAN_POINT('Ctrl Pts',(1.73425417885907,-1.,1.34824783112887));
#18291=CARTESIAN_POINT('Ctrl Pts',(1.7304014965394,-1.,1.34779309152035));
#18292=CARTESIAN_POINT('Ctrl Pts',(1.72527410680674,-1.,1.34716554819527));
#18293=CARTESIAN_POINT('Ctrl Pts',(1.7188807715049,-1.,1.34634568653227));
#18294=CARTESIAN_POINT('Ctrl Pts',(1.71250340686822,-1.,1.34549029589416));
#18295=CARTESIAN_POINT('Ctrl Pts',(1.70614212266738,-1.,1.34459924533831));
#18296=CARTESIAN_POINT('Ctrl Pts',(1.69979707754427,-1.,1.34367237124483));
#18297=CARTESIAN_POINT('Ctrl Pts',(1.6934684849687,-1.,1.34270948206319));
#18298=CARTESIAN_POINT('Ctrl Pts',(1.68715660868764,-1.,1.341710374848));
#18299=CARTESIAN_POINT('Ctrl Pts',(1.68086176030362,-1.,1.34067485185203));
#18300=CARTESIAN_POINT('Ctrl Pts',(1.67458429426086,-1.,1.3396027347034));
#18301=CARTESIAN_POINT('Ctrl Pts',(1.66832460783989,-1.,1.33849388654388));
#18302=CARTESIAN_POINT('Ctrl Pts',(1.66208312541983,-1.,1.33734820885262));
#18303=CARTESIAN_POINT('Ctrl Pts',(1.65586025952593,-1.,1.33616559745172));
#18304=CARTESIAN_POINT('Ctrl Pts',(1.6496563728683,-1.,1.33494590467993));
#18305=CARTESIAN_POINT('Ctrl Pts',(1.6434717485603,-1.,1.33368890676572));
#18306=CARTESIAN_POINT('Ctrl Pts',(1.63730653475089,-1.,1.33239425103724));
#18307=CARTESIAN_POINT('Ctrl Pts',(1.63116079730923,-1.,1.33106149345645));
#18308=CARTESIAN_POINT('Ctrl Pts',(1.62503464209797,-1.,1.3296901950568));
#18309=CARTESIAN_POINT('Ctrl Pts',(1.61892832270724,-1.,1.32828000610449));
#18310=CARTESIAN_POINT('Ctrl Pts',(1.6128423401575,-1.,1.32683074483356));
#18311=CARTESIAN_POINT('Ctrl Pts',(1.60677758290954,-1.,1.32534250785782));
#18312=CARTESIAN_POINT('Ctrl Pts',(1.60073511858687,-1.,1.32381550858256));
#18313=CARTESIAN_POINT('Ctrl Pts',(1.59471591079403,-1.,1.32224985747682));
#18314=CARTESIAN_POINT('Ctrl Pts',(1.58872057258245,-1.,1.32064537110892));
#18315=CARTESIAN_POINT('Ctrl Pts',(1.58274907898834,-1.,1.31900135021432));
#18316=CARTESIAN_POINT('Ctrl Pts',(1.5768005650559,-1.,1.31731642317187));
#18317=CARTESIAN_POINT('Ctrl Pts',(1.57087397835723,-1.,1.31558903860016));
#18318=CARTESIAN_POINT('Ctrl Pts',(1.56496872402353,-1.,1.31381795281002));
#18319=CARTESIAN_POINT('Ctrl Pts',(1.55908521254821,-1.,1.31200264341696));
#18320=CARTESIAN_POINT('Ctrl Pts',(1.55322568759481,-1.,1.31014393684222));
#18321=CARTESIAN_POINT('Ctrl Pts',(1.54739413957185,-1.,1.30824393907473));
#18322=CARTESIAN_POINT('Ctrl Pts',(1.54159462645432,-1.,1.30630475189556));
#18323=CARTESIAN_POINT('Ctrl Pts',(1.53582981268977,-1.,1.30432735639489));
#18324=CARTESIAN_POINT('Ctrl Pts',(1.53009970283891,-1.,1.30231064395568));
#18325=CARTESIAN_POINT('Ctrl Pts',(1.52439957861062,-1.,1.30024984366328));
#18326=CARTESIAN_POINT('Ctrl Pts',(1.51872184912724,-1.,1.29813791800747));
#18327=CARTESIAN_POINT('Ctrl Pts',(1.51305994241402,-1.,1.29596850710509));
#18328=CARTESIAN_POINT('Ctrl Pts',(1.50741159078365,-1.,1.29373841372842));
#18329=CARTESIAN_POINT('Ctrl Pts',(1.50178230149776,-1.,1.29145022885181));
#18330=CARTESIAN_POINT('Ctrl Pts',(1.49618896881754,-1.,1.28911506584254));
#18331=CARTESIAN_POINT('Ctrl Pts',(1.4906522831278,-1.,1.2867467611644));
#18332=CARTESIAN_POINT('Ctrl Pts',(1.4851881711891,-1.,1.28435533880201));
#18333=CARTESIAN_POINT('Ctrl Pts',(1.47980070347095,-1.,1.28194158939517));
#18334=CARTESIAN_POINT('Ctrl Pts',(1.4744717526707,-1.,1.2794891824849));
#18335=CARTESIAN_POINT('Ctrl Pts',(1.46916035917133,-1.,1.2769641483109));
#18336=CARTESIAN_POINT('Ctrl Pts',(1.46382431332476,-1.,1.27433119897822));
#18337=CARTESIAN_POINT('Ctrl Pts',(1.45843906294697,-1.,1.27156805265289));
#18338=CARTESIAN_POINT('Ctrl Pts',(1.45301422764247,-1.,1.2686778680489));
#18339=CARTESIAN_POINT('Ctrl Pts',(1.44761985001662,-1.,1.26570925118868));
#18340=CARTESIAN_POINT('Ctrl Pts',(1.44236470511303,-1.,1.26273903323859));
#18341=CARTESIAN_POINT('Ctrl Pts',(1.43734919180847,-1.,1.25983531012005));
#18342=CARTESIAN_POINT('Ctrl Pts',(1.43262645609691,-1.,1.25702687965755));
#18343=CARTESIAN_POINT('Ctrl Pts',(1.42815938799387,-1.,1.25426945222639));
#18344=CARTESIAN_POINT('Ctrl Pts',(1.42378102115575,-1.,1.2514145557001));
#18345=CARTESIAN_POINT('Ctrl Pts',(1.41923722596025,-1.,1.24824430986571));
#18346=CARTESIAN_POINT('Ctrl Pts',(1.41422913175179,-1.,1.24450600513056));
#18347=CARTESIAN_POINT('Ctrl Pts',(1.40845295531283,-1.,1.23994455029534));
#18348=CARTESIAN_POINT('Ctrl Pts',(1.40164708206106,-1.,1.23434087290423));
#18349=CARTESIAN_POINT('Ctrl Pts',(1.39361389568796,-1.,1.22752961899387));
#18350=CARTESIAN_POINT('Ctrl Pts',(1.38420564527715,-1.,1.21938737280852));
#18351=CARTESIAN_POINT('Ctrl Pts',(1.37331915607905,-1.,1.20982812925645));
#18352=CARTESIAN_POINT('Ctrl Pts',(1.36088705043885,-1.,1.1987959077932));
#18353=CARTESIAN_POINT('Ctrl Pts',(1.34687054001093,-1.,1.18625865667441));
#18354=CARTESIAN_POINT('Ctrl Pts',(1.33437539347008,-1.,1.17501305789857));
#18355=CARTESIAN_POINT('Ctrl Pts',(1.32428080721772,-1.,1.16589330093588));
#18356=CARTESIAN_POINT('Ctrl Pts',(1.31722977216397,-1.,1.15950888730809));
#18357=CARTESIAN_POINT('Ctrl Pts',(1.31362392696032,-1.,1.15624053661742));
#18358=CARTESIAN_POINT('',(1.15624053661742,-1.,1.31362392696033));
#18359=CARTESIAN_POINT('Origin',(0.,-1.,0.));
#18360=CARTESIAN_POINT('',(1.34869019493419,-1.,1.73811241238545));
#18361=CARTESIAN_POINT('Ctrl Pts',(1.15624053661742,-1.,1.31362392696033));
#18362=CARTESIAN_POINT('Ctrl Pts',(1.15950888730433,-1.,1.3172297721596));
#18363=CARTESIAN_POINT('Ctrl Pts',(1.16589330092532,-1.,1.32428080720544));
#18364=CARTESIAN_POINT('Ctrl Pts',(1.17501305787994,-1.,1.33437539344842));
#18365=CARTESIAN_POINT('Ctrl Pts',(1.18625865664915,-1.,1.34687053998157));
#18366=CARTESIAN_POINT('Ctrl Pts',(1.1987959077656,-1.,1.36088705040677));
#18367=CARTESIAN_POINT('Ctrl Pts',(1.20982812923113,-1.,1.37331915604962));
#18368=CARTESIAN_POINT('Ctrl Pts',(1.21938737278853,-1.,1.38420564525391));
#18369=CARTESIAN_POINT('Ctrl Pts',(1.22752961898063,-1.,1.39361389567257));
#18370=CARTESIAN_POINT('Ctrl Pts',(1.23434087289768,-1.,1.40164708205345));
#18371=CARTESIAN_POINT('Ctrl Pts',(1.23994455029421,-1.,1.40845295531151));
#18372=CARTESIAN_POINT('Ctrl Pts',(1.24450600513278,-1.,1.41422913175437));
#18373=CARTESIAN_POINT('Ctrl Pts',(1.24824430986911,-1.,1.41923722596421));
#18374=CARTESIAN_POINT('Ctrl Pts',(1.25141455570299,-1.,1.42378102115911));
#18375=CARTESIAN_POINT('Ctrl Pts',(1.25426945222783,-1.,1.42815938799555));
#18376=CARTESIAN_POINT('Ctrl Pts',(1.25702687965744,-1.,1.43262645609679));
#18377=CARTESIAN_POINT('Ctrl Pts',(1.25983531011894,-1.,1.43734919180719));
#18378=CARTESIAN_POINT('Ctrl Pts',(1.26273903323723,-1.,1.44236470511145));
#18379=CARTESIAN_POINT('Ctrl Pts',(1.26570925118767,-1.,1.44761985001544));
#18380=CARTESIAN_POINT('Ctrl Pts',(1.26867786804854,-1.,1.45301422764205));
#18381=CARTESIAN_POINT('Ctrl Pts',(1.27156805265312,-1.,1.45843906294725));
#18382=CARTESIAN_POINT('Ctrl Pts',(1.27433119897877,-1.,1.4638243133254));
#18383=CARTESIAN_POINT('Ctrl Pts',(1.27696414831144,-1.,1.46916035917197));
#18384=CARTESIAN_POINT('Ctrl Pts',(1.27948918248524,-1.,1.4744717526711));
#18385=CARTESIAN_POINT('Ctrl Pts',(1.28194158939522,-1.,1.47980070347102));
#18386=CARTESIAN_POINT('Ctrl Pts',(1.28435533880184,-1.,1.48518817118891));
#18387=CARTESIAN_POINT('Ctrl Pts',(1.28674676116415,-1.,1.4906522831275));
#18388=CARTESIAN_POINT('Ctrl Pts',(1.28911506584232,-1.,1.49618896881729));
#18389=CARTESIAN_POINT('Ctrl Pts',(1.29145022885171,-1.,1.50178230149764));
#18390=CARTESIAN_POINT('Ctrl Pts',(1.29373841372843,-1.,1.50741159078367));
#18391=CARTESIAN_POINT('Ctrl Pts',(1.29596850710518,-1.,1.51305994241412));
#18392=CARTESIAN_POINT('Ctrl Pts',(1.29813791800757,-1.,1.51872184912735));
#18393=CARTESIAN_POINT('Ctrl Pts',(1.30024984366334,-1.,1.5243995786107));
#18394=CARTESIAN_POINT('Ctrl Pts',(1.3023106439557,-1.,1.53009970283893));
#18395=CARTESIAN_POINT('Ctrl Pts',(1.30432735639487,-1.,1.53582981268976));
#18396=CARTESIAN_POINT('Ctrl Pts',(1.30630475189553,-1.,1.54159462645428));
#18397=CARTESIAN_POINT('Ctrl Pts',(1.30824393907471,-1.,1.54739413957183));
#18398=CARTESIAN_POINT('Ctrl Pts',(1.31014393684221,-1.,1.55322568759481));
#18399=CARTESIAN_POINT('Ctrl Pts',(1.31200264341696,-1.,1.55908521254822));
#18400=CARTESIAN_POINT('Ctrl Pts',(1.31381795281002,-1.,1.56496872402352));
#18401=CARTESIAN_POINT('Ctrl Pts',(1.31558903860015,-1.,1.57087397835721));
#18402=CARTESIAN_POINT('Ctrl Pts',(1.31731642317183,-1.,1.57680056505585));
#18403=CARTESIAN_POINT('Ctrl Pts',(1.31900135021428,-1.,1.58274907898829));
#18404=CARTESIAN_POINT('Ctrl Pts',(1.32064537110891,-1.,1.58872057258244));
#18405=CARTESIAN_POINT('Ctrl Pts',(1.32224985747686,-1.,1.59471591079408));
#18406=CARTESIAN_POINT('Ctrl Pts',(1.32381550858266,-1.,1.600735118587));
#18407=CARTESIAN_POINT('Ctrl Pts',(1.32534250785794,-1.,1.6067775829097));
#18408=CARTESIAN_POINT('Ctrl Pts',(1.32683074483365,-1.,1.61284234015762));
#18409=CARTESIAN_POINT('Ctrl Pts',(1.32828000610448,-1.,1.61892832270723));
#18410=CARTESIAN_POINT('Ctrl Pts',(1.32969019505665,-1.,1.62503464209777));
#18411=CARTESIAN_POINT('Ctrl Pts',(1.33106149345618,-1.,1.63116079730887));
#18412=CARTESIAN_POINT('Ctrl Pts',(1.33239425103694,-1.,1.6373065347505));
#18413=CARTESIAN_POINT('Ctrl Pts',(1.33368890676554,-1.,1.64347174856007));
#18414=CARTESIAN_POINT('Ctrl Pts',(1.33494590468003,-1.,1.64965637286843));
#18415=CARTESIAN_POINT('Ctrl Pts',(1.33616559745217,-1.,1.65586025952651));
#18416=CARTESIAN_POINT('Ctrl Pts',(1.33734820885331,-1.,1.66208312542073));
#18417=CARTESIAN_POINT('Ctrl Pts',(1.33849388654458,-1.,1.66832460784078));
#18418=CARTESIAN_POINT('Ctrl Pts',(1.33960273470372,-1.,1.67458429426126));
#18419=CARTESIAN_POINT('Ctrl Pts',(1.3406748518516,-1.,1.68086176030308));
#18420=CARTESIAN_POINT('Ctrl Pts',(1.34171037484673,-1.,1.68715660868602));
#18421=CARTESIAN_POINT('Ctrl Pts',(1.34270948206139,-1.,1.6934684849664));
#18422=CARTESIAN_POINT('Ctrl Pts',(1.34367237124322,-1.,1.69979707754221));
#18423=CARTESIAN_POINT('Ctrl Pts',(1.34459924533783,-1.,1.70614212266676));
#18424=CARTESIAN_POINT('Ctrl Pts',(1.34549029589563,-1.,1.71250340687011));
#18425=CARTESIAN_POINT('Ctrl Pts',(1.34634568653586,-1.,1.7188807715095));
#18426=CARTESIAN_POINT('Ctrl Pts',(1.34716554820013,-1.,1.72527410681298));
#18427=CARTESIAN_POINT('Ctrl Pts',(1.3477930915247,-1.,1.73040149654497));
#18428=CARTESIAN_POINT('Ctrl Pts',(1.34824783113158,-1.,1.73425417886255));
#18429=CARTESIAN_POINT('Ctrl Pts',(1.34854391898145,-1.,1.73682580585819));
#18430=CARTESIAN_POINT('Ctrl Pts',(1.34869019493419,-1.,1.73811241238545));
#18431=CARTESIAN_POINT('',(1.23627494547115,-1.,1.81978687191668));
#18432=CARTESIAN_POINT('',(1.34869019493419,-1.,1.73811241238545));
#18433=CARTESIAN_POINT('',(0.892032620296855,-1.,1.5055822144029));
#18434=CARTESIAN_POINT('Ctrl Pts',(1.23627494547115,-1.,1.81978687191668));
#18435=CARTESIAN_POINT('Ctrl Pts',(1.23509651170384,-1.,1.81925017193531));
#18436=CARTESIAN_POINT('Ctrl Pts',(1.23274224526804,-1.,1.81817389920914));
#18437=CARTESIAN_POINT('Ctrl Pts',(1.22921864890975,-1.,1.81655087183054));
#18438=CARTESIAN_POINT('Ctrl Pts',(1.22453613304507,-1.,1.81436959209778));
#18439=CARTESIAN_POINT('Ctrl Pts',(1.2187090610323,-1.,1.81161420806172));
#18440=CARTESIAN_POINT('Ctrl Pts',(1.2129081570818,-1.,1.80882996916931));
#18441=CARTESIAN_POINT('Ctrl Pts',(1.20713356605519,-1.,1.80601678480772));
#18442=CARTESIAN_POINT('Ctrl Pts',(1.2013854893912,-1.,1.8031745483882));
#18443=CARTESIAN_POINT('Ctrl Pts',(1.19566418930405,-1.,1.80030314370121));
#18444=CARTESIAN_POINT('Ctrl Pts',(1.1899699793456,-1.,1.79740245923649));
#18445=CARTESIAN_POINT('Ctrl Pts',(1.18430321697471,-1.,1.79447240321572));
#18446=CARTESIAN_POINT('Ctrl Pts',(1.17866429440781,-1.,1.79151291552646));
#18447=CARTESIAN_POINT('Ctrl Pts',(1.17305363177265,-1.,1.78852398877523));
#18448=CARTESIAN_POINT('Ctrl Pts',(1.16747166312239,-1.,1.78550566040349));
#18449=CARTESIAN_POINT('Ctrl Pts',(1.16191881298458,-1.,1.78245795880949));
#18450=CARTESIAN_POINT('Ctrl Pts',(1.15639547194689,-1.,1.77938085564261));
#18451=CARTESIAN_POINT('Ctrl Pts',(1.15090197841531,-1.,1.77627422557034));
#18452=CARTESIAN_POINT('Ctrl Pts',(1.14543858226948,-1.,1.77313777896234));
#18453=CARTESIAN_POINT('Ctrl Pts',(1.14000548337,-1.,1.76997111386806));
#18454=CARTESIAN_POINT('Ctrl Pts',(1.13460291804634,-1.,1.76677384551883));
#18455=CARTESIAN_POINT('Ctrl Pts',(1.12923123555076,-1.,1.76354571966171));
#18456=CARTESIAN_POINT('Ctrl Pts',(1.12389096855078,-1.,1.76028671825084));
#18457=CARTESIAN_POINT('Ctrl Pts',(1.11858293216752,-1.,1.75699720772089));
#18458=CARTESIAN_POINT('Ctrl Pts',(1.11330807582542,-1.,1.75367772094617));
#18459=CARTESIAN_POINT('Ctrl Pts',(1.10806728183003,-1.,1.75032866075914));
#18460=CARTESIAN_POINT('Ctrl Pts',(1.10286118991144,-1.,1.74695004214924));
#18461=CARTESIAN_POINT('Ctrl Pts',(1.09768999241229,-1.,1.74354119236212));
#18462=CARTESIAN_POINT('Ctrl Pts',(1.09255329056496,-1.,1.74010053962252));
#18463=CARTESIAN_POINT('Ctrl Pts',(1.08745056285429,-1.,1.73662628326093));
#18464=CARTESIAN_POINT('Ctrl Pts',(1.08238162784749,-1.,1.73311705663407));
#18465=CARTESIAN_POINT('Ctrl Pts',(1.0773470373727,-1.,1.72957248977424));
#18466=CARTESIAN_POINT('Ctrl Pts',(1.07234866990252,-1.,1.72599406198489));
#18467=CARTESIAN_POINT('Ctrl Pts',(1.06738966975463,-1.,1.72238500928456));
#18468=CARTESIAN_POINT('Ctrl Pts',(1.06247324680649,-1.,1.71874858456908));
#18469=CARTESIAN_POINT('Ctrl Pts',(1.05760163192481,-1.,1.71508654427022));
#18470=CARTESIAN_POINT('Ctrl Pts',(1.05277517202853,-1.,1.71139783543986));
#18471=CARTESIAN_POINT('Ctrl Pts',(1.0479908540499,-1.,1.70767646263641));
#18472=CARTESIAN_POINT('Ctrl Pts',(1.04324363334546,-1.,1.70391338707969));
#18473=CARTESIAN_POINT('Ctrl Pts',(1.03852922490782,-1.,1.70010052930951));
#18474=CARTESIAN_POINT('Ctrl Pts',(1.03384646003587,-1.,1.69623414782769));
#18475=CARTESIAN_POINT('Ctrl Pts',(1.02919977579155,-1.,1.69231840863471));
#18476=CARTESIAN_POINT('Ctrl Pts',(1.02460180535272,-1.,1.68836910178475));
#18477=CARTESIAN_POINT('Ctrl Pts',(1.02006795074222,-1.,1.68440578021739));
#18478=CARTESIAN_POINT('Ctrl Pts',(1.01561026162786,-1.,1.6804428989482));
#18479=CARTESIAN_POINT('Ctrl Pts',(1.01123236493507,-1.,1.67648246776457));
#18480=CARTESIAN_POINT('Ctrl Pts',(1.00692206696387,-1.,1.67250335383248));
#18481=CARTESIAN_POINT('Ctrl Pts',(1.00265091003682,-1.,1.66846059277231));
#18482=CARTESIAN_POINT('Ctrl Pts',(0.998389654952317,-1.,1.66430758030304));
#18483=CARTESIAN_POINT('Ctrl Pts',(0.994121836661115,-1.,1.66001553809916));
#18484=CARTESIAN_POINT('Ctrl Pts',(0.98985562785445,-1.,1.65559044289746));
#18485=CARTESIAN_POINT('Ctrl Pts',(0.985642622921626,-1.,1.6511001661277));
#18486=CARTESIAN_POINT('Ctrl Pts',(0.981562530940574,-1.,1.64665139190834));
#18487=CARTESIAN_POINT('Ctrl Pts',(0.977689794120296,-1.,1.64233990826831));
#18488=CARTESIAN_POINT('Ctrl Pts',(0.974066058287501,-1.,1.63820952658157));
#18489=CARTESIAN_POINT('Ctrl Pts',(0.970669715996356,-1.,1.63420665729609));
#18490=CARTESIAN_POINT('Ctrl Pts',(0.967387853228041,-1.,1.63013849959083));
#18491=CARTESIAN_POINT('Ctrl Pts',(0.964046107037821,-1.,1.6257193066974));
#18492=CARTESIAN_POINT('Ctrl Pts',(0.960438326099958,-1.,1.62061638139929));
#18493=CARTESIAN_POINT('Ctrl Pts',(0.956354422921572,-1.,1.61449324337233));
#18494=CARTESIAN_POINT('Ctrl Pts',(0.951613284361247,-1.,1.60706069897794));
#18495=CARTESIAN_POINT('Ctrl Pts',(0.946078063325795,-1.,1.59810042045408));
#18496=CARTESIAN_POINT('Ctrl Pts',(0.939646377909319,-1.,1.58744937489796));
#18497=CARTESIAN_POINT('Ctrl Pts',(0.932246680128848,-1.,1.57499388385561));
#18498=CARTESIAN_POINT('Ctrl Pts',(0.923832188966322,-1.,1.56065988582509));
#18499=CARTESIAN_POINT('Ctrl Pts',(0.914375919046579,-1.,1.54440491152808));
#18500=CARTESIAN_POINT('Ctrl Pts',(0.905967409640498,-1.,1.52984849890434));
#18501=CARTESIAN_POINT('Ctrl Pts',(0.89918504749193,-1.,1.51805569591479));
#18502=CARTESIAN_POINT('Ctrl Pts',(0.894452006967538,-1.,1.50980486807181));
#18503=CARTESIAN_POINT('Ctrl Pts',(0.892032620296855,-1.,1.5055822144029));
#18504=CARTESIAN_POINT('',(0.693717979106305,-1.,1.60662857109684));
#18505=CARTESIAN_POINT('Origin',(0.,-1.,0.));
#18506=CARTESIAN_POINT('',(0.7455743247944,-1.,2.0698113262342));
#18507=CARTESIAN_POINT('Ctrl Pts',(0.693717979106305,-1.,1.60662857109684));
#18508=CARTESIAN_POINT('Ctrl Pts',(0.69571209787897,-1.,1.61106790957619));
#18509=CARTESIAN_POINT('Ctrl Pts',(0.699605146398836,-1.,1.61974673471117));
#18510=CARTESIAN_POINT('Ctrl Pts',(0.705159151977294,-1.,1.6321654166204));
#18511=CARTESIAN_POINT('Ctrl Pts',(0.711993139340447,-1.,1.64752408828442));
#18512=CARTESIAN_POINT('Ctrl Pts',(0.719585433787949,-1.,1.66472880551777));
#18513=CARTESIAN_POINT('Ctrl Pts',(0.726235967982445,-1.,1.67996158451922));
#18514=CARTESIAN_POINT('Ctrl Pts',(0.731963238685357,-1.,1.69326921972915));
#18515=CARTESIAN_POINT('Ctrl Pts',(0.736799665716932,-1.,1.70473309004249));
#18516=CARTESIAN_POINT('Ctrl Pts',(0.74079516202821,-1.,1.71447789751001));
#18517=CARTESIAN_POINT('Ctrl Pts',(0.744021445433093,-1.,1.72268229916769));
#18518=CARTESIAN_POINT('Ctrl Pts',(0.746574710097752,-1.,1.72958533647714));
#18519=CARTESIAN_POINT('Ctrl Pts',(0.74858246295687,-1.,1.7355035168033));
#18520=CARTESIAN_POINT('Ctrl Pts',(0.750193435981249,-1.,1.74080458267114));
#18521=CARTESIAN_POINT('Ctrl Pts',(0.751555614164482,-1.,1.74585086852502));
#18522=CARTESIAN_POINT('Ctrl Pts',(0.752797683531314,-1.,1.75095139468794));
#18523=CARTESIAN_POINT('Ctrl Pts',(0.754009254027828,-1.,1.75631083600019));
#18524=CARTESIAN_POINT('Ctrl Pts',(0.755220979974461,-1.,1.76197817240128));
#18525=CARTESIAN_POINT('Ctrl Pts',(0.75642189602781,-1.,1.76789396002998));
#18526=CARTESIAN_POINT('Ctrl Pts',(0.757578264077028,-1.,1.77394167108292));
#18527=CARTESIAN_POINT('Ctrl Pts',(0.758650626677518,-1.,1.77999411220945));
#18528=CARTESIAN_POINT('Ctrl Pts',(0.759614401110189,-1.,1.78596964884604));
#18529=CARTESIAN_POINT('Ctrl Pts',(0.760469555880749,-1.,1.7918581561088));
#18530=CARTESIAN_POINT('Ctrl Pts',(0.761229695230558,-1.,1.79768986997783));
#18531=CARTESIAN_POINT('Ctrl Pts',(0.761915336443547,-1.,1.80351583877342));
#18532=CARTESIAN_POINT('Ctrl Pts',(0.762546129463938,-1.,1.80938551463965));
#18533=CARTESIAN_POINT('Ctrl Pts',(0.763132003836634,-1.,1.8153211840553));
#18534=CARTESIAN_POINT('Ctrl Pts',(0.763673465462726,-1.,1.82131873145266));
#18535=CARTESIAN_POINT('Ctrl Pts',(0.764165902605995,-1.,1.82735991200065));
#18536=CARTESIAN_POINT('Ctrl Pts',(0.764602549687853,-1.,1.83342077227142));
#18537=CARTESIAN_POINT('Ctrl Pts',(0.764978057881737,-1.,1.83948181064835));
#18538=CARTESIAN_POINT('Ctrl Pts',(0.765291664862029,-1.,1.84553698875924));
#18539=CARTESIAN_POINT('Ctrl Pts',(0.765545710619062,-1.,1.85158945130063));
#18540=CARTESIAN_POINT('Ctrl Pts',(0.765744212909318,-1.,1.85764741390394));
#18541=CARTESIAN_POINT('Ctrl Pts',(0.765891519092547,-1.,1.86372027063312));
#18542=CARTESIAN_POINT('Ctrl Pts',(0.765990708546091,-1.,1.86981398314341));
#18543=CARTESIAN_POINT('Ctrl Pts',(0.766042837036744,-1.,1.87592888967883));
#18544=CARTESIAN_POINT('Ctrl Pts',(0.766047794851864,-1.,1.88206215302561));
#18545=CARTESIAN_POINT('Ctrl Pts',(0.766004837062091,-1.,1.88820926433409));
#18546=CARTESIAN_POINT('Ctrl Pts',(0.765913193856978,-1.,1.89436577771388));
#18547=CARTESIAN_POINT('Ctrl Pts',(0.765772772593386,-1.,1.90052930393596));
#18548=CARTESIAN_POINT('Ctrl Pts',(0.765584196937919,-1.,1.90669961402356));
#18549=CARTESIAN_POINT('Ctrl Pts',(0.765348465884722,-1.,1.91287765805169));
#18550=CARTESIAN_POINT('Ctrl Pts',(0.765066729667088,-1.,1.91906491634196));
#18551=CARTESIAN_POINT('Ctrl Pts',(0.764740025488211,-1.,1.92526263537048));
#18552=CARTESIAN_POINT('Ctrl Pts',(0.76436901067394,-1.,1.93147105496382));
#18553=CARTESIAN_POINT('Ctrl Pts',(0.763954049121458,-1.,1.93768964875886));
#18554=CARTESIAN_POINT('Ctrl Pts',(0.763495333538629,-1.,1.9439174661764));
#18555=CARTESIAN_POINT('Ctrl Pts',(0.762992990878769,-1.,1.95015342590024));
#18556=CARTESIAN_POINT('Ctrl Pts',(0.762447203806178,-1.,1.95639665309869));
#18557=CARTESIAN_POINT('Ctrl Pts',(0.761858300014423,-1.,1.96264672744186));
#18558=CARTESIAN_POINT('Ctrl Pts',(0.76122669048382,-1.,1.96890351582499));
#18559=CARTESIAN_POINT('Ctrl Pts',(0.760552825409757,-1.,1.97516705321494));
#18560=CARTESIAN_POINT('Ctrl Pts',(0.75983714745219,-1.,1.98143741418172));
#18561=CARTESIAN_POINT('Ctrl Pts',(0.759080037802488,-1.,1.98771456680874));
#18562=CARTESIAN_POINT('Ctrl Pts',(0.758281796766761,-1.,1.99399831098817));
#18563=CARTESIAN_POINT('Ctrl Pts',(0.757442676862724,-1.,2.00028834739178));
#18564=CARTESIAN_POINT('Ctrl Pts',(0.75656290464667,-1.,2.0065843158773));
#18565=CARTESIAN_POINT('Ctrl Pts',(0.755642704957865,-1.,2.01288584328084));
#18566=CARTESIAN_POINT('Ctrl Pts',(0.754682330722816,-1.,2.01919259405809));
#18567=CARTESIAN_POINT('Ctrl Pts',(0.753682061112768,-1.,2.02550428623313));
#18568=CARTESIAN_POINT('Ctrl Pts',(0.75264218048721,-1.,2.03182068456221));
#18569=CARTESIAN_POINT('Ctrl Pts',(0.751562963361115,-1.,2.03814160092099));
#18570=CARTESIAN_POINT('Ctrl Pts',(0.750444657875575,-1.,2.04446689147979));
#18571=CARTESIAN_POINT('Ctrl Pts',(0.749287468665046,-1.,2.05079645592154));
#18572=CARTESIAN_POINT('Ctrl Pts',(0.748091554183802,-1.,2.05713023031007));
#18573=CARTESIAN_POINT('Ctrl Pts',(0.747103932787919,-1.,2.06220058927826));
#18574=CARTESIAN_POINT('Ctrl Pts',(0.7463458715442,-1.,2.06600523016815));
#18575=CARTESIAN_POINT('Ctrl Pts',(0.745832791378367,-1.,2.06854248895728));
#18576=CARTESIAN_POINT('Ctrl Pts',(0.7455743247944,-1.,2.0698113262342));
#18577=CARTESIAN_POINT('',(0.61342227326009,-1.,2.11275013067528));
#18578=CARTESIAN_POINT('',(0.7455743247944,-1.,2.0698113262342));
#18579=CARTESIAN_POINT('',(0.383122945602004,-1.,1.7075470150345));
#18580=CARTESIAN_POINT('Ctrl Pts',(0.61342227326009,-1.,2.11275013067528));
#18581=CARTESIAN_POINT('Ctrl Pts',(0.6124673655618,-1.,2.11187554259986));
#18582=CARTESIAN_POINT('Ctrl Pts',(0.610560911689898,-1.,2.11012443807238));
#18583=CARTESIAN_POINT('Ctrl Pts',(0.607711315454876,-1.,2.1074919961518));
#18584=CARTESIAN_POINT('Ctrl Pts',(0.60393203073603,-1.,2.10397049886949));
#18585=CARTESIAN_POINT('Ctrl Pts',(0.599241616420533,-1.,2.0995493086477));
#18586=CARTESIAN_POINT('Ctrl Pts',(0.594585006052162,-1.,2.0951087622027));
#18587=CARTESIAN_POINT('Ctrl Pts',(0.589962365403406,-1.,2.09064881812129));
#18588=CARTESIAN_POINT('Ctrl Pts',(0.585373918991617,-1.,2.08616943727951));
#18589=CARTESIAN_POINT('Ctrl Pts',(0.580819952108063,-1.,2.08167059018418));
#18590=CARTESIAN_POINT('Ctrl Pts',(0.576300797416844,-1.,2.07715226767559));
#18591=CARTESIAN_POINT('Ctrl Pts',(0.571816823242602,-1.,2.07261449292824));
#18592=CARTESIAN_POINT('Ctrl Pts',(0.567368421181087,-1.,2.06805732997334));
#18593=CARTESIAN_POINT('Ctrl Pts',(0.562955993082261,-1.,2.06348090160589));
#18594=CARTESIAN_POINT('Ctrl Pts',(0.558579940185151,-1.,2.05888537756462));
#18595=CARTESIAN_POINT('Ctrl Pts',(0.554240657463906,-1.,2.05427091604413));
#18596=CARTESIAN_POINT('Ctrl Pts',(0.549938525150295,-1.,2.04963761077958));
#18597=CARTESIAN_POINT('Ctrl Pts',(0.54567390381743,-1.,2.04498544714588));
#18598=CARTESIAN_POINT('Ctrl Pts',(0.541447120615659,-1.,2.04031422690527));
#18599=CARTESIAN_POINT('Ctrl Pts',(0.537258489833262,-1.,2.03562362954037));
#18600=CARTESIAN_POINT('Ctrl Pts',(0.533108355132976,-1.,2.03091336214426));
#18601=CARTESIAN_POINT('Ctrl Pts',(0.528997127241914,-1.,2.0261832908329));
#18602=CARTESIAN_POINT('Ctrl Pts',(0.524925318333476,-1.,2.02143356304698));
#18603=CARTESIAN_POINT('Ctrl Pts',(0.52089359039937,-1.,2.01666477917286));
#18604=CARTESIAN_POINT('Ctrl Pts',(0.516902681728687,-1.,2.01187773939242));
#18605=CARTESIAN_POINT('Ctrl Pts',(0.512953306961792,-1.,2.00707309946949));
#18606=CARTESIAN_POINT('Ctrl Pts',(0.509046069886157,-1.,2.00225107134734));
#18607=CARTESIAN_POINT('Ctrl Pts',(0.505181361323026,-1.,1.99741107463572));
#18608=CARTESIAN_POINT('Ctrl Pts',(0.501359287727146,-1.,1.99255149126155));
#18609=CARTESIAN_POINT('Ctrl Pts',(0.497579909545574,-1.,1.98767044752932));
#18610=CARTESIAN_POINT('Ctrl Pts',(0.493843476541494,-1.,1.98276658761821));
#18611=CARTESIAN_POINT('Ctrl Pts',(0.490150627860952,-1.,1.97783973019229));
#18612=CARTESIAN_POINT('Ctrl Pts',(0.486502692907658,-1.,1.97289186263272));
#18613=CARTESIAN_POINT('Ctrl Pts',(0.48290166212069,-1.,1.96792703422362));
#18614=CARTESIAN_POINT('Ctrl Pts',(0.479349583074855,-1.,1.96294933055943));
#18615=CARTESIAN_POINT('Ctrl Pts',(0.475848034683176,-1.,1.95796111148177));
#18616=CARTESIAN_POINT('Ctrl Pts',(0.472397672264072,-1.,1.95296148278133));
#18617=CARTESIAN_POINT('Ctrl Pts',(0.468997482913135,-1.,1.94794381136514));
#18618=CARTESIAN_POINT('Ctrl Pts',(0.46564546202603,-1.,1.9428979419619));
#18619=CARTESIAN_POINT('Ctrl Pts',(0.462340031009056,-1.,1.93781486640821));
#18620=CARTESIAN_POINT('Ctrl Pts',(0.459081234547926,-1.,1.93269066517934));
#18621=CARTESIAN_POINT('Ctrl Pts',(0.45587200517437,-1.,1.92753067150476));
#18622=CARTESIAN_POINT('Ctrl Pts',(0.452719478359432,-1.,1.92235380648502));
#18623=CARTESIAN_POINT('Ctrl Pts',(0.449632260106662,-1.,1.91718342555755));
#18624=CARTESIAN_POINT('Ctrl Pts',(0.446617343485711,-1.,1.9120369998112));
#18625=CARTESIAN_POINT('Ctrl Pts',(0.44367755684915,-1.,1.90691756144898));
#18626=CARTESIAN_POINT('Ctrl Pts',(0.440807833704038,-1.,1.90180124389086));
#18627=CARTESIAN_POINT('Ctrl Pts',(0.437995003948244,-1.,1.89663648956466));
#18628=CARTESIAN_POINT('Ctrl Pts',(0.435225660963383,-1.,1.89136993975504));
#18629=CARTESIAN_POINT('Ctrl Pts',(0.432493038548748,-1.,1.88596913666793));
#18630=CARTESIAN_POINT('Ctrl Pts',(0.429803062482344,-1.,1.88044229001832));
#18631=CARTESIAN_POINT('Ctrl Pts',(0.427183828519102,-1.,1.87486989291484));
#18632=CARTESIAN_POINT('Ctrl Pts',(0.424678177291358,-1.,1.86937803944323));
#18633=CARTESIAN_POINT('Ctrl Pts',(0.422327307418275,-1.,1.86408083334028));
#18634=CARTESIAN_POINT('Ctrl Pts',(0.420157287975619,-1.,1.85903281096686));
#18635=CARTESIAN_POINT('Ctrl Pts',(0.418164129143534,-1.,1.85417632856234));
#18636=CARTESIAN_POINT('Ctrl Pts',(0.416300022038864,-1.,1.84929312929882));
#18637=CARTESIAN_POINT('Ctrl Pts',(0.41448743825434,-1.,1.8440575707371));
#18638=CARTESIAN_POINT('Ctrl Pts',(0.412633125322161,-1.,1.83808953475839));
#18639=CARTESIAN_POINT('Ctrl Pts',(0.410641256301674,-1.,1.83100408895216));
#18640=CARTESIAN_POINT('Ctrl Pts',(0.408428948108533,-1.,1.8224702267854));
#18641=CARTESIAN_POINT('Ctrl Pts',(0.405933518411838,-1.,1.81223801813988));
#18642=CARTESIAN_POINT('Ctrl Pts',(0.403107976170441,-1.,1.80012077176221));
#18643=CARTESIAN_POINT('Ctrl Pts',(0.39991940378308,-1.,1.78598826347533));
#18644=CARTESIAN_POINT('Ctrl Pts',(0.39634619612042,-1.,1.7697556004756));
#18645=CARTESIAN_POINT('Ctrl Pts',(0.392375812294307,-1.,1.75137405313962));
#18646=CARTESIAN_POINT('Ctrl Pts',(0.388877023509191,-1.,1.7349317097561));
#18647=CARTESIAN_POINT('Ctrl Pts',(0.38607079032701,-1.,1.72162022246158));
#18648=CARTESIAN_POINT('Ctrl Pts',(0.384119047315541,-1.,1.71231062891958));
#18649=CARTESIAN_POINT('Ctrl Pts',(0.383122945602004,-1.,1.7075470150345));
#18650=CARTESIAN_POINT('',(0.163289472382896,-1.,1.74236521665491));
#18651=CARTESIAN_POINT('Origin',(0.,-1.,0.));
#18652=CARTESIAN_POINT('',(0.0694764450219578,-1.,2.19890268624765));
#18653=CARTESIAN_POINT('Ctrl Pts',(0.163289472382896,-1.,1.74236521665491));
#18654=CARTESIAN_POINT('Ctrl Pts',(0.163814161002002,-1.,1.7472034950333));
#18655=CARTESIAN_POINT('Ctrl Pts',(0.164834765707158,-1.,1.75666056638427));
#18656=CARTESIAN_POINT('Ctrl Pts',(0.1662793551464,-1.,1.77018771684844));
#18657=CARTESIAN_POINT('Ctrl Pts',(0.168032772805197,-1.,1.7869064998507));
#18658=CARTESIAN_POINT('Ctrl Pts',(0.169936923904608,-1.,1.80561530629706));
#18659=CARTESIAN_POINT('Ctrl Pts',(0.171554770204119,-1.,1.82215766811545));
#18660=CARTESIAN_POINT('Ctrl Pts',(0.1728894428919,-1.,1.83658380527692));
#18661=CARTESIAN_POINT('Ctrl Pts',(0.173946627587731,-1.,1.8489811319852));
#18662=CARTESIAN_POINT('Ctrl Pts',(0.17473525927603,-1.,1.85948367088837));
#18663=CARTESIAN_POINT('Ctrl Pts',(0.175268337590757,-1.,1.86828349694799));
#18664=CARTESIAN_POINT('Ctrl Pts',(0.175563480746485,-1.,1.87563767773588));
#18665=CARTESIAN_POINT('Ctrl Pts',(0.175644148889698,-1.,1.88188663145367));
#18666=CARTESIAN_POINT('Ctrl Pts',(0.175538155840648,-1.,1.88742606273259));
#18667=CARTESIAN_POINT('Ctrl Pts',(0.175274276190844,-1.,1.892646301985));
#18668=CARTESIAN_POINT('Ctrl Pts',(0.174879405091263,-1.,1.89788101117132));
#18669=CARTESIAN_POINT('Ctrl Pts',(0.174375518661085,-1.,1.90335253862834));
#18670=CARTESIAN_POINT('Ctrl Pts',(0.173776635257816,-1.,1.90911693975267));
#18671=CARTESIAN_POINT('Ctrl Pts',(0.173090695383496,-1.,1.91511429159527));
#18672=CARTESIAN_POINT('Ctrl Pts',(0.172321621259513,-1.,1.9212233439798));
#18673=CARTESIAN_POINT('Ctrl Pts',(0.171471191532988,-1.,1.92731093582036));
#18674=CARTESIAN_POINT('Ctrl Pts',(0.170541253116201,-1.,1.93329183155539));
#18675=CARTESIAN_POINT('Ctrl Pts',(0.16953490481749,-1.,1.93915639211581));
#18676=CARTESIAN_POINT('Ctrl Pts',(0.168455741607556,-1.,1.94493757756931));
#18677=CARTESIAN_POINT('Ctrl Pts',(0.167307501784475,-1.,1.95069027794294));
#18678=CARTESIAN_POINT('Ctrl Pts',(0.166093592002812,-1.,1.9564675971873));
#18679=CARTESIAN_POINT('Ctrl Pts',(0.164816568920269,-1.,1.96229379940136));
#18680=CARTESIAN_POINT('Ctrl Pts',(0.163478185457734,-1.,1.96816512677967));
#18681=CARTESIAN_POINT('Ctrl Pts',(0.162079693556288,-1.,1.97406280235188));
#18682=CARTESIAN_POINT('Ctrl Pts',(0.160622060784611,-1.,1.97996195437559));
#18683=CARTESIAN_POINT('Ctrl Pts',(0.159106226437299,-1.,1.98584238283292));
#18684=CARTESIAN_POINT('Ctrl Pts',(0.157533331459227,-1.,1.99169810931908));
#18685=CARTESIAN_POINT('Ctrl Pts',(0.155904629548783,-1.,1.99753284771497));
#18686=CARTESIAN_POINT('Ctrl Pts',(0.154221403049722,-1.,2.00335565310543));
#18687=CARTESIAN_POINT('Ctrl Pts',(0.152484883621449,-1.,2.00917680318424));
#18688=CARTESIAN_POINT('Ctrl Pts',(0.150696157673078,-1.,2.01500291940238));
#18689=CARTESIAN_POINT('Ctrl Pts',(0.148856124775337,-1.,2.02083464969894));
#18690=CARTESIAN_POINT('Ctrl Pts',(0.146965557332583,-1.,2.02666926182017));
#18691=CARTESIAN_POINT('Ctrl Pts',(0.145025140186057,-1.,2.03250223739942));
#18692=CARTESIAN_POINT('Ctrl Pts',(0.143035515058208,-1.,2.03832911025912));
#18693=CARTESIAN_POINT('Ctrl Pts',(0.140997332152546,-1.,2.04414757947916));
#18694=CARTESIAN_POINT('Ctrl Pts',(0.138911255368966,-1.,2.04995762001328));
#18695=CARTESIAN_POINT('Ctrl Pts',(0.136777941218043,-1.,2.05576044414264));
#18696=CARTESIAN_POINT('Ctrl Pts',(0.134598026192106,-1.,2.06155781517842));
#18697=CARTESIAN_POINT('Ctrl Pts',(0.13237211154771,-1.,2.06735123910326));
#18698=CARTESIAN_POINT('Ctrl Pts',(0.130100748328403,-1.,2.07314114713063));
#18699=CARTESIAN_POINT('Ctrl Pts',(0.12778444527612,-1.,2.07892715110987));
#18700=CARTESIAN_POINT('Ctrl Pts',(0.125423679412061,-1.,2.08470840653643));
#18701=CARTESIAN_POINT('Ctrl Pts',(0.123018905621083,-1.,2.09048392424825));
#18702=CARTESIAN_POINT('Ctrl Pts',(0.120570567965122,-1.,2.0962529286773));
#18703=CARTESIAN_POINT('Ctrl Pts',(0.118079107988355,-1.,2.102015121329));
#18704=CARTESIAN_POINT('Ctrl Pts',(0.115544957687926,-1.,2.10777050261309));
#18705=CARTESIAN_POINT('Ctrl Pts',(0.112968534419737,-1.,2.11351924490306));
#18706=CARTESIAN_POINT('Ctrl Pts',(0.110350236135025,-1.,2.11926155590865));
#18707=CARTESIAN_POINT('Ctrl Pts',(0.10769043523109,-1.,2.12499752307));
#18708=CARTESIAN_POINT('Ctrl Pts',(0.104989479152739,-1.,2.13072704887293));
#18709=CARTESIAN_POINT('Ctrl Pts',(0.1022477005561,-1.,2.13644992667165));
#18710=CARTESIAN_POINT('Ctrl Pts',(0.0994654261990913,-1.,2.14216588396025));
#18711=CARTESIAN_POINT('Ctrl Pts',(0.0966429852305456,-1.,2.14787463531795));
#18712=CARTESIAN_POINT('Ctrl Pts',(0.0937807218867641,-1.,2.1535759397817));
#18713=CARTESIAN_POINT('Ctrl Pts',(0.0908789888107263,-1.,2.15926961544516));
#18714=CARTESIAN_POINT('Ctrl Pts',(0.087938129138692,-1.,2.16495552645014));
#18715=CARTESIAN_POINT('Ctrl Pts',(0.084958462083537,-1.,2.17063357870952));
#18716=CARTESIAN_POINT('Ctrl Pts',(0.0819402680872763,-1.,2.176303712113));
#18717=CARTESIAN_POINT('Ctrl Pts',(0.078883772768524,-1.,2.18196589448887));
#18718=CARTESIAN_POINT('Ctrl Pts',(0.0757891465836145,-1.,2.1876201139953));
#18719=CARTESIAN_POINT('Ctrl Pts',(0.0732830357306722,-1.,2.19213712013662));
#18720=CARTESIAN_POINT('Ctrl Pts',(0.0713863779526151,-1.,2.19552129484002));
#18721=CARTESIAN_POINT('Ctrl Pts',(0.0701143536325487,-1.,2.19777582085423));
#18722=CARTESIAN_POINT('Ctrl Pts',(0.0694764450219578,-1.,2.19890268624765));
#18723=CARTESIAN_POINT('',(-0.0694764450219586,-1.,2.19890268624765));
#18724=CARTESIAN_POINT('',(0.0694764450219578,-1.,2.19890268624765));
#18725=CARTESIAN_POINT('',(-0.163289472382896,-1.,1.74236521665491));
#18726=CARTESIAN_POINT('Ctrl Pts',(-0.0694764450219586,-1.,2.19890268624765));
#18727=CARTESIAN_POINT('Ctrl Pts',(-0.0701143536324929,-1.,2.19777582085261));
#18728=CARTESIAN_POINT('Ctrl Pts',(-0.071386377952463,-1.,2.19552129483562));
#18729=CARTESIAN_POINT('Ctrl Pts',(-0.0732830357304279,-1.,2.19213712012956));
#18730=CARTESIAN_POINT('Ctrl Pts',(-0.0757891465833414,-1.,2.1876201139874));
#18731=CARTESIAN_POINT('Ctrl Pts',(-0.078883772768323,-1.,2.18196589448304));
#18732=CARTESIAN_POINT('Ctrl Pts',(-0.0819402680871942,-1.,2.1763037121106));
#18733=CARTESIAN_POINT('Ctrl Pts',(-0.0849584620835646,-1.,2.17063357871031));
#18734=CARTESIAN_POINT('Ctrl Pts',(-0.0879381291387825,-1.,2.16495552645275));
#18735=CARTESIAN_POINT('Ctrl Pts',(-0.0908789888108269,-1.,2.15926961544808));
#18736=CARTESIAN_POINT('Ctrl Pts',(-0.0937807218868348,-1.,2.15357593978377));
#18737=CARTESIAN_POINT('Ctrl Pts',(-0.0966429852305691,-1.,2.14787463531864));
#18738=CARTESIAN_POINT('Ctrl Pts',(-0.0994654261990745,-1.,2.14216588395974));
#18739=CARTESIAN_POINT('Ctrl Pts',(-0.102247700556064,-1.,2.13644992667052));
#18740=CARTESIAN_POINT('Ctrl Pts',(-0.104989479152703,-1.,2.1307270488718));
#18741=CARTESIAN_POINT('Ctrl Pts',(-0.107690435231068,-1.,2.12499752306927));
#18742=CARTESIAN_POINT('Ctrl Pts',(-0.11035023613502,-1.,2.11926155590849));
#18743=CARTESIAN_POINT('Ctrl Pts',(-0.112968534419746,-1.,2.11351924490335));
#18744=CARTESIAN_POINT('Ctrl Pts',(-0.115544957687941,-1.,2.10777050261359));
#18745=CARTESIAN_POINT('Ctrl Pts',(-0.118079107988368,-1.,2.10201512132945));
#18746=CARTESIAN_POINT('Ctrl Pts',(-0.120570567965129,-1.,2.09625292867756));
#18747=CARTESIAN_POINT('Ctrl Pts',(-0.123018905621083,-1.,2.09048392424826));
#18748=CARTESIAN_POINT('Ctrl Pts',(-0.125423679412058,-1.,2.08470840653628));
#18749=CARTESIAN_POINT('Ctrl Pts',(-0.127784445276116,-1.,2.07892715110967));
#18750=CARTESIAN_POINT('Ctrl Pts',(-0.130100748328401,-1.,2.07314114713047));
#18751=CARTESIAN_POINT('Ctrl Pts',(-0.13237211154771,-1.,2.06735123910319));
#18752=CARTESIAN_POINT('Ctrl Pts',(-0.134598026192107,-1.,2.06155781517844));
#18753=CARTESIAN_POINT('Ctrl Pts',(-0.136777941218044,-1.,2.0557604441427));
#18754=CARTESIAN_POINT('Ctrl Pts',(-0.138911255368966,-1.,2.04995762001333));
#18755=CARTESIAN_POINT('Ctrl Pts',(-0.140997332152546,-1.,2.04414757947919));
#18756=CARTESIAN_POINT('Ctrl Pts',(-0.143035515058208,-1.,2.03832911025913));
#18757=CARTESIAN_POINT('Ctrl Pts',(-0.145025140186058,-1.,2.03250223739941));
#18758=CARTESIAN_POINT('Ctrl Pts',(-0.146965557332586,-1.,2.02666926182017));
#18759=CARTESIAN_POINT('Ctrl Pts',(-0.148856124775343,-1.,2.02083464969897));
#18760=CARTESIAN_POINT('Ctrl Pts',(-0.150696157673084,-1.,2.01500291940243));
#18761=CARTESIAN_POINT('Ctrl Pts',(-0.152484883621452,-1.,2.00917680318426));
#18762=CARTESIAN_POINT('Ctrl Pts',(-0.154221403049719,-1.,2.00335565310539));
#18763=CARTESIAN_POINT('Ctrl Pts',(-0.155904629548775,-1.,1.99753284771487));
#18764=CARTESIAN_POINT('Ctrl Pts',(-0.157533331459215,-1.,1.99169810931893));
#18765=CARTESIAN_POINT('Ctrl Pts',(-0.159106226437289,-1.,1.98584238283279));
#18766=CARTESIAN_POINT('Ctrl Pts',(-0.16062206078461,-1.,1.97996195437557));
#18767=CARTESIAN_POINT('Ctrl Pts',(-0.162079693556302,-1.,1.97406280235204));
#18768=CARTESIAN_POINT('Ctrl Pts',(-0.16347818545776,-1.,1.96816512678));
#18769=CARTESIAN_POINT('Ctrl Pts',(-0.1648165689203,-1.,1.96229379940174));
#18770=CARTESIAN_POINT('Ctrl Pts',(-0.166093592002833,-1.,1.95646759718755));
#18771=CARTESIAN_POINT('Ctrl Pts',(-0.167307501784469,-1.,1.95069027794286));
#18772=CARTESIAN_POINT('Ctrl Pts',(-0.168455741607516,-1.,1.94493757756879));
#18773=CARTESIAN_POINT('Ctrl Pts',(-0.169534904817425,-1.,1.93915639211497));
#18774=CARTESIAN_POINT('Ctrl Pts',(-0.170541253116136,-1.,1.93329183155455));
#18775=CARTESIAN_POINT('Ctrl Pts',(-0.17147119153296,-1.,1.92731093582));
#18776=CARTESIAN_POINT('Ctrl Pts',(-0.172321621259557,-1.,1.92122334398034));
#18777=CARTESIAN_POINT('Ctrl Pts',(-0.173090695383619,-1.,1.91511429159681));
#18778=CARTESIAN_POINT('Ctrl Pts',(-0.173776635257984,-1.,1.90911693975475));
#18779=CARTESIAN_POINT('Ctrl Pts',(-0.174375518661222,-1.,1.90335253863003));
#18780=CARTESIAN_POINT('Ctrl Pts',(-0.174879405091277,-1.,1.89788101117148));
#18781=CARTESIAN_POINT('Ctrl Pts',(-0.175274276190664,-1.,1.89264630198279));
#18782=CARTESIAN_POINT('Ctrl Pts',(-0.175538155840286,-1.,1.88742606272818));
#18783=CARTESIAN_POINT('Ctrl Pts',(-0.175644148889271,-1.,1.88188663144846));
#18784=CARTESIAN_POINT('Ctrl Pts',(-0.175563480746206,-1.,1.87563767773249));
#18785=CARTESIAN_POINT('Ctrl Pts',(-0.175268337590901,-1.,1.86828349694972));
#18786=CARTESIAN_POINT('Ctrl Pts',(-0.174735259276856,-1.,1.85948367089838));
#18787=CARTESIAN_POINT('Ctrl Pts',(-0.173946627589401,-1.,1.84898113200543));
#18788=CARTESIAN_POINT('Ctrl Pts',(-0.17288944289442,-1.,1.83658380530747));
#18789=CARTESIAN_POINT('Ctrl Pts',(-0.171554770207306,-1.,1.82215766815414));
#18790=CARTESIAN_POINT('Ctrl Pts',(-0.169936923908078,-1.,1.80561530633924));
#18791=CARTESIAN_POINT('Ctrl Pts',(-0.16803277280837,-1.,1.78690649988931));
#18792=CARTESIAN_POINT('Ctrl Pts',(-0.166279355148738,-1.,1.77018771687692));
#18793=CARTESIAN_POINT('Ctrl Pts',(-0.164834765708484,-1.,1.75666056640041));
#18794=CARTESIAN_POINT('Ctrl Pts',(-0.163814161002474,-1.,1.74720349503904));
#18795=CARTESIAN_POINT('Ctrl Pts',(-0.163289472382896,-1.,1.74236521665491));
#18796=CARTESIAN_POINT('',(-0.383122945602004,-1.,1.7075470150345));
#18797=CARTESIAN_POINT('Origin',(0.,-1.,0.));
#18798=CARTESIAN_POINT('',(-0.61342227326009,-1.,2.11275013067528));
#18799=CARTESIAN_POINT('Ctrl Pts',(-0.383122945602004,-1.,1.7075470150345));
#18800=CARTESIAN_POINT('Ctrl Pts',(-0.384119047314215,-1.,1.71231062891398));
#18801=CARTESIAN_POINT('Ctrl Pts',(-0.386070790323281,-1.,1.72162022244582));
#18802=CARTESIAN_POINT('Ctrl Pts',(-0.388877023502615,-1.,1.73493170972829));
#18803=CARTESIAN_POINT('Ctrl Pts',(-0.392375812285395,-1.,1.75137405310193));
#18804=CARTESIAN_POINT('Ctrl Pts',(-0.396346196110688,-1.,1.76975560043442));
#18805=CARTESIAN_POINT('Ctrl Pts',(-0.399919403774155,-1.,1.78598826343754));
#18806=CARTESIAN_POINT('Ctrl Pts',(-0.403107976163396,-1.,1.80012077173238));
#18807=CARTESIAN_POINT('Ctrl Pts',(-0.405933518407175,-1.,1.81223801812013));
#18808=CARTESIAN_POINT('Ctrl Pts',(-0.408428948106227,-1.,1.82247022677562));
#18809=CARTESIAN_POINT('Ctrl Pts',(-0.410641256301276,-1.,1.83100408895047));
#18810=CARTESIAN_POINT('Ctrl Pts',(-0.412633125322945,-1.,1.8380895347617));
#18811=CARTESIAN_POINT('Ctrl Pts',(-0.414487438255542,-1.,1.84405757074218));
#18812=CARTESIAN_POINT('Ctrl Pts',(-0.416300022039885,-1.,1.84929312930314));
#18813=CARTESIAN_POINT('Ctrl Pts',(-0.418164129144045,-1.,1.8541763285645));
#18814=CARTESIAN_POINT('Ctrl Pts',(-0.420157287975583,-1.,1.8590328109667));
#18815=CARTESIAN_POINT('Ctrl Pts',(-0.422327307417885,-1.,1.86408083333863));
#18816=CARTESIAN_POINT('Ctrl Pts',(-0.424678177290876,-1.,1.8693780394412));
#18817=CARTESIAN_POINT('Ctrl Pts',(-0.427183828518743,-1.,1.87486989291333));
#18818=CARTESIAN_POINT('Ctrl Pts',(-0.429803062482217,-1.,1.88044229001778));
#18819=CARTESIAN_POINT('Ctrl Pts',(-0.432493038548833,-1.,1.88596913666828));
#18820=CARTESIAN_POINT('Ctrl Pts',(-0.43522566096358,-1.,1.89136993975585));
#18821=CARTESIAN_POINT('Ctrl Pts',(-0.437995003948443,-1.,1.89663648956549));
#18822=CARTESIAN_POINT('Ctrl Pts',(-0.440807833704161,-1.,1.90180124389137));
#18823=CARTESIAN_POINT('Ctrl Pts',(-0.44367755684917,-1.,1.90691756144906));
#18824=CARTESIAN_POINT('Ctrl Pts',(-0.446617343485651,-1.,1.91203699981095));
#18825=CARTESIAN_POINT('Ctrl Pts',(-0.449632260106572,-1.,1.91718342555717));
#18826=CARTESIAN_POINT('Ctrl Pts',(-0.452719478359356,-1.,1.9223538064847));
#18827=CARTESIAN_POINT('Ctrl Pts',(-0.455872005174335,-1.,1.92753067150461));
#18828=CARTESIAN_POINT('Ctrl Pts',(-0.459081234547931,-1.,1.93269066517936));
#18829=CARTESIAN_POINT('Ctrl Pts',(-0.462340031009087,-1.,1.93781486640834));
#18830=CARTESIAN_POINT('Ctrl Pts',(-0.465645462026065,-1.,1.94289794196205));
#18831=CARTESIAN_POINT('Ctrl Pts',(-0.468997482913158,-1.,1.94794381136524));
#18832=CARTESIAN_POINT('Ctrl Pts',(-0.47239767226408,-1.,1.95296148278136));
#18833=CARTESIAN_POINT('Ctrl Pts',(-0.475848034683172,-1.,1.95796111148175));
#18834=CARTESIAN_POINT('Ctrl Pts',(-0.479349583074846,-1.,1.96294933055938));
#18835=CARTESIAN_POINT('Ctrl Pts',(-0.482901662120687,-1.,1.96792703422358));
#18836=CARTESIAN_POINT('Ctrl Pts',(-0.486502692907661,-1.,1.97289186263272));
#18837=CARTESIAN_POINT('Ctrl Pts',(-0.490150627860955,-1.,1.97783973019229));
#18838=CARTESIAN_POINT('Ctrl Pts',(-0.493843476541492,-1.,1.9827665876182));
#18839=CARTESIAN_POINT('Ctrl Pts',(-0.497579909545564,-1.,1.98767044752929));
#18840=CARTESIAN_POINT('Ctrl Pts',(-0.501359287727129,-1.,1.9925514912615));
#18841=CARTESIAN_POINT('Ctrl Pts',(-0.505181361323011,-1.,1.99741107463567));
#18842=CARTESIAN_POINT('Ctrl Pts',(-0.509046069886152,-1.,2.00225107134733));
#18843=CARTESIAN_POINT('Ctrl Pts',(-0.512953306961814,-1.,2.00707309946955));
#18844=CARTESIAN_POINT('Ctrl Pts',(-0.516902681728733,-1.,2.01187773939257));
#18845=CARTESIAN_POINT('Ctrl Pts',(-0.520893590399428,-1.,2.01666477917305));
#18846=CARTESIAN_POINT('Ctrl Pts',(-0.524925318333518,-1.,2.02143356304712));
#18847=CARTESIAN_POINT('Ctrl Pts',(-0.528997127241911,-1.,2.02618329083289));
#18848=CARTESIAN_POINT('Ctrl Pts',(-0.533108355132905,-1.,2.03091336214401));
#18849=CARTESIAN_POINT('Ctrl Pts',(-0.537258489833134,-1.,2.03562362953993));
#18850=CARTESIAN_POINT('Ctrl Pts',(-0.54144712061552,-1.,2.0403142269048));
#18851=CARTESIAN_POINT('Ctrl Pts',(-0.545673903817348,-1.,2.0449854471456));
#18852=CARTESIAN_POINT('Ctrl Pts',(-0.549938525150342,-1.,2.04963761077974));
#18853=CARTESIAN_POINT('Ctrl Pts',(-0.55424065746411,-1.,2.05427091604482));
#18854=CARTESIAN_POINT('Ctrl Pts',(-0.558579940185467,-1.,2.05888537756571));
#18855=CARTESIAN_POINT('Ctrl Pts',(-0.562955993082574,-1.,2.06348090160697));
#18856=CARTESIAN_POINT('Ctrl Pts',(-0.567368421181229,-1.,2.06805732997383));
#18857=CARTESIAN_POINT('Ctrl Pts',(-0.571816823242411,-1.,2.07261449292757));
#18858=CARTESIAN_POINT('Ctrl Pts',(-0.576300797416275,-1.,2.07715226767361));
#18859=CARTESIAN_POINT('Ctrl Pts',(-0.580819952107257,-1.,2.08167059018138));
#18860=CARTESIAN_POINT('Ctrl Pts',(-0.585373918990895,-1.,2.086169437277));
#18861=CARTESIAN_POINT('Ctrl Pts',(-0.589962365403189,-1.,2.09064881812053));
#18862=CARTESIAN_POINT('Ctrl Pts',(-0.594585006052824,-1.,2.09510876220501));
#18863=CARTESIAN_POINT('Ctrl Pts',(-0.599241616422144,-1.,2.09954930865331));
#18864=CARTESIAN_POINT('Ctrl Pts',(-0.603932030738212,-1.,2.10397049887709));
#18865=CARTESIAN_POINT('Ctrl Pts',(-0.607711315456826,-1.,2.10749199615859));
#18866=CARTESIAN_POINT('Ctrl Pts',(-0.610560911691113,-1.,2.11012443807661));
#18867=CARTESIAN_POINT('Ctrl Pts',(-0.61246736556225,-1.,2.11187554260142));
#18868=CARTESIAN_POINT('Ctrl Pts',(-0.61342227326009,-1.,2.11275013067528));
#18869=CARTESIAN_POINT('',(-0.745574324794401,-1.,2.0698113262342));
#18870=CARTESIAN_POINT('',(-0.61342227326009,-1.,2.11275013067528));
#18871=CARTESIAN_POINT('',(-0.693717979106306,-1.,1.60662857109684));
#18872=CARTESIAN_POINT('Ctrl Pts',(-0.745574324794401,-1.,2.0698113262342));
#18873=CARTESIAN_POINT('Ctrl Pts',(-0.74583279137781,-1.,2.06854248895575));
#18874=CARTESIAN_POINT('Ctrl Pts',(-0.746345871542696,-1.,2.06600523016401));
#18875=CARTESIAN_POINT('Ctrl Pts',(-0.747103932785504,-1.,2.06220058927162));
#18876=CARTESIAN_POINT('Ctrl Pts',(-0.748091554181101,-1.,2.05713023030263));
#18877=CARTESIAN_POINT('Ctrl Pts',(-0.749287468663053,-1.,2.05079645591606));
#18878=CARTESIAN_POINT('Ctrl Pts',(-0.750444657874758,-1.,2.04446689147754));
#18879=CARTESIAN_POINT('Ctrl Pts',(-0.751562963361384,-1.,2.03814160092173));
#18880=CARTESIAN_POINT('Ctrl Pts',(-0.752642180488104,-1.,2.03182068456467));
#18881=CARTESIAN_POINT('Ctrl Pts',(-0.753682061113766,-1.,2.02550428623587));
#18882=CARTESIAN_POINT('Ctrl Pts',(-0.75468233072352,-1.,2.01919259406003));
#18883=CARTESIAN_POINT('Ctrl Pts',(-0.7556427049581,-1.,2.01288584328149));
#18884=CARTESIAN_POINT('Ctrl Pts',(-0.756562904646496,-1.,2.00658431587682));
#18885=CARTESIAN_POINT('Ctrl Pts',(-0.757442676862341,-1.,2.00028834739072));
#18886=CARTESIAN_POINT('Ctrl Pts',(-0.758281796766377,-1.,1.9939983109871));
#18887=CARTESIAN_POINT('Ctrl Pts',(-0.759080037802243,-1.,1.98771456680806));
#18888=CARTESIAN_POINT('Ctrl Pts',(-0.759837147452135,-1.,1.98143741418156));
#18889=CARTESIAN_POINT('Ctrl Pts',(-0.760552825409855,-1.,1.97516705321521));
#18890=CARTESIAN_POINT('Ctrl Pts',(-0.761226690483986,-1.,1.96890351582545));
#18891=CARTESIAN_POINT('Ctrl Pts',(-0.761858300014575,-1.,1.96264672744229));
#18892=CARTESIAN_POINT('Ctrl Pts',(-0.762447203806263,-1.,1.95639665309893));
#18893=CARTESIAN_POINT('Ctrl Pts',(-0.762992990878774,-1.,1.95015342590025));
#18894=CARTESIAN_POINT('Ctrl Pts',(-0.76349533353858,-1.,1.94391746617626));
#18895=CARTESIAN_POINT('Ctrl Pts',(-0.763954049121393,-1.,1.93768964875867));
#18896=CARTESIAN_POINT('Ctrl Pts',(-0.764369010673889,-1.,1.93147105496367));
#18897=CARTESIAN_POINT('Ctrl Pts',(-0.764740025488189,-1.,1.92526263537041));
#18898=CARTESIAN_POINT('Ctrl Pts',(-0.765066729667095,-1.,1.91906491634197));
#18899=CARTESIAN_POINT('Ctrl Pts',(-0.765348465884739,-1.,1.91287765805174));
#18900=CARTESIAN_POINT('Ctrl Pts',(-0.765584196937936,-1.,1.90669961402362));
#18901=CARTESIAN_POINT('Ctrl Pts',(-0.765772772593395,-1.,1.90052930393599));
#18902=CARTESIAN_POINT('Ctrl Pts',(-0.765913193856979,-1.,1.89436577771389));
#18903=CARTESIAN_POINT('Ctrl Pts',(-0.76600483706209,-1.,1.88820926433409));
#18904=CARTESIAN_POINT('Ctrl Pts',(-0.766047794851869,-1.,1.88206215302561));
#18905=CARTESIAN_POINT('Ctrl Pts',(-0.766042837036759,-1.,1.87592888967886));
#18906=CARTESIAN_POINT('Ctrl Pts',(-0.765990708546111,-1.,1.86981398314345));
#18907=CARTESIAN_POINT('Ctrl Pts',(-0.765891519092557,-1.,1.86372027063314));
#18908=CARTESIAN_POINT('Ctrl Pts',(-0.765744212909305,-1.,1.85764741390391));
#18909=CARTESIAN_POINT('Ctrl Pts',(-0.765545710619023,-1.,1.85158945130054));
#18910=CARTESIAN_POINT('Ctrl Pts',(-0.765291664861971,-1.,1.8455369887591));
#18911=CARTESIAN_POINT('Ctrl Pts',(-0.764978057881687,-1.,1.83948181064823));
#18912=CARTESIAN_POINT('Ctrl Pts',(-0.764602549687845,-1.,1.8334207722714));
#18913=CARTESIAN_POINT('Ctrl Pts',(-0.764165902606055,-1.,1.8273599120008));
#18914=CARTESIAN_POINT('Ctrl Pts',(-0.763673465462854,-1.,1.82131873145297));
#18915=CARTESIAN_POINT('Ctrl Pts',(-0.763132003836783,-1.,1.81532118405566));
#18916=CARTESIAN_POINT('Ctrl Pts',(-0.762546129464036,-1.,1.80938551463989));
#18917=CARTESIAN_POINT('Ctrl Pts',(-0.761915336443516,-1.,1.80351583877334));
#18918=CARTESIAN_POINT('Ctrl Pts',(-0.761229695230359,-1.,1.79768986997735));
#18919=CARTESIAN_POINT('Ctrl Pts',(-0.760469555880425,-1.,1.79185815610802));
#18920=CARTESIAN_POINT('Ctrl Pts',(-0.759614401109868,-1.,1.78596964884526));
#18921=CARTESIAN_POINT('Ctrl Pts',(-0.75865062667738,-1.,1.77999411220912));
#18922=CARTESIAN_POINT('Ctrl Pts',(-0.757578264077238,-1.,1.77394167108342));
#18923=CARTESIAN_POINT('Ctrl Pts',(-0.756421896028403,-1.,1.76789396003141));
#18924=CARTESIAN_POINT('Ctrl Pts',(-0.755220979975262,-1.,1.7619781724032));
#18925=CARTESIAN_POINT('Ctrl Pts',(-0.75400925402848,-1.,1.75631083600175));
#18926=CARTESIAN_POINT('Ctrl Pts',(-0.752797683531377,-1.,1.75095139468809));
#18927=CARTESIAN_POINT('Ctrl Pts',(-0.751555614163629,-1.,1.74585086852298));
#18928=CARTESIAN_POINT('Ctrl Pts',(-0.75019343597954,-1.,1.74080458266705));
#18929=CARTESIAN_POINT('Ctrl Pts',(-0.748582462954855,-1.,1.73550351679848));
#18930=CARTESIAN_POINT('Ctrl Pts',(-0.746574710096436,-1.,1.72958533647399));
#18931=CARTESIAN_POINT('Ctrl Pts',(-0.744021445433764,-1.,1.7226822991693));
#18932=CARTESIAN_POINT('Ctrl Pts',(-0.740795162032088,-1.,1.71447789751927));
#18933=CARTESIAN_POINT('Ctrl Pts',(-0.736799665724771,-1.,1.70473309006121));
#18934=CARTESIAN_POINT('Ctrl Pts',(-0.731963238697195,-1.,1.69326921975743));
#18935=CARTESIAN_POINT('Ctrl Pts',(-0.726235967997433,-1.,1.67996158455503));
#18936=CARTESIAN_POINT('Ctrl Pts',(-0.719585433804282,-1.,1.6647288055568));
#18937=CARTESIAN_POINT('Ctrl Pts',(-0.711993139355394,-1.,1.64752408832016));
#18938=CARTESIAN_POINT('Ctrl Pts',(-0.705159151988319,-1.,1.63216541664676));
#18939=CARTESIAN_POINT('Ctrl Pts',(-0.699605146405088,-1.,1.61974673472612));
#18940=CARTESIAN_POINT('Ctrl Pts',(-0.695712097881194,-1.,1.61106790958151));
#18941=CARTESIAN_POINT('Ctrl Pts',(-0.693717979106306,-1.,1.60662857109684));
#18942=CARTESIAN_POINT('',(-0.892032620296855,-1.,1.5055822144029));
#18943=CARTESIAN_POINT('Origin',(0.,-1.,0.));
#18944=CARTESIAN_POINT('',(-1.23627494547115,-1.,1.81978687191668));
#18945=CARTESIAN_POINT('Ctrl Pts',(-0.892032620296855,-1.,1.5055822144029));
#18946=CARTESIAN_POINT('Ctrl Pts',(-0.894452006964543,-1.,1.50980486806688));
#18947=CARTESIAN_POINT('Ctrl Pts',(-0.899185047483511,-1.,1.51805569590094));
#18948=CARTESIAN_POINT('Ctrl Pts',(-0.905967409625651,-1.,1.52984849887993));
#18949=CARTESIAN_POINT('Ctrl Pts',(-0.914375919026456,-1.,1.54440491149498));
#18950=CARTESIAN_POINT('Ctrl Pts',(-0.923832188944341,-1.,1.56065988578893));
#18951=CARTESIAN_POINT('Ctrl Pts',(-0.932246680108685,-1.,1.57499388382243));
#18952=CARTESIAN_POINT('Ctrl Pts',(-0.939646377893399,-1.,1.58744937487176));
#18953=CARTESIAN_POINT('Ctrl Pts',(-0.946078063315257,-1.,1.59810042043673));
#18954=CARTESIAN_POINT('Ctrl Pts',(-0.951613284356035,-1.,1.60706069896936));
#18955=CARTESIAN_POINT('Ctrl Pts',(-0.956354422920671,-1.,1.61449324337085));
#18956=CARTESIAN_POINT('Ctrl Pts',(-0.960438326101729,-1.,1.62061638140221));
#18957=CARTESIAN_POINT('Ctrl Pts',(-0.964046107040536,-1.,1.62571930670187));
#18958=CARTESIAN_POINT('Ctrl Pts',(-0.967387853230345,-1.,1.63013849959461));
#18959=CARTESIAN_POINT('Ctrl Pts',(-0.970669715997509,-1.,1.63420665729798));
#18960=CARTESIAN_POINT('Ctrl Pts',(-0.974066058287418,-1.,1.63820952658144));
#18961=CARTESIAN_POINT('Ctrl Pts',(-0.977689794119416,-1.,1.64233990826687));
#18962=CARTESIAN_POINT('Ctrl Pts',(-0.981562530939489,-1.,1.64665139190656));
#18963=CARTESIAN_POINT('Ctrl Pts',(-0.985642622920821,-1.,1.65110016612638));
#18964=CARTESIAN_POINT('Ctrl Pts',(-0.989855627854165,-1.,1.65559044289699));
#18965=CARTESIAN_POINT('Ctrl Pts',(-0.994121836661306,-1.,1.66001553809947));
#18966=CARTESIAN_POINT('Ctrl Pts',(-0.998389654952758,-1.,1.66430758030376));
#18967=CARTESIAN_POINT('Ctrl Pts',(-1.00265091003727,-1.,1.66846059277303));
#18968=CARTESIAN_POINT('Ctrl Pts',(-1.00692206696414,-1.,1.67250335383293));
#18969=CARTESIAN_POINT('Ctrl Pts',(-1.01123236493511,-1.,1.67648246776464));
#18970=CARTESIAN_POINT('Ctrl Pts',(-1.01561026162773,-1.,1.68044289894798));
#18971=CARTESIAN_POINT('Ctrl Pts',(-1.02006795074201,-1.,1.68440578021706));
#18972=CARTESIAN_POINT('Ctrl Pts',(-1.02460180535255,-1.,1.68836910178447));
#18973=CARTESIAN_POINT('Ctrl Pts',(-1.02919977579147,-1.,1.69231840863458));
#18974=CARTESIAN_POINT('Ctrl Pts',(-1.03384646003588,-1.,1.69623414782771));
#18975=CARTESIAN_POINT('Ctrl Pts',(-1.03852922490789,-1.,1.70010052930962));
#18976=CARTESIAN_POINT('Ctrl Pts',(-1.04324363334554,-1.,1.70391338707982));
#18977=CARTESIAN_POINT('Ctrl Pts',(-1.04799085404995,-1.,1.70767646263649));
#18978=CARTESIAN_POINT('Ctrl Pts',(-1.05277517202855,-1.,1.71139783543989));
#18979=CARTESIAN_POINT('Ctrl Pts',(-1.05760163192479,-1.,1.7150865442702));
#18980=CARTESIAN_POINT('Ctrl Pts',(-1.06247324680647,-1.,1.71874858456904));
#18981=CARTESIAN_POINT('Ctrl Pts',(-1.06738966975462,-1.,1.72238500928453));
#18982=CARTESIAN_POINT('Ctrl Pts',(-1.07234866990252,-1.,1.72599406198488));
#18983=CARTESIAN_POINT('Ctrl Pts',(-1.0773470373727,-1.,1.72957248977424));
#18984=CARTESIAN_POINT('Ctrl Pts',(-1.08238162784749,-1.,1.73311705663407));
#18985=CARTESIAN_POINT('Ctrl Pts',(-1.08745056285427,-1.,1.73662628326091));
#18986=CARTESIAN_POINT('Ctrl Pts',(-1.09255329056493,-1.,1.74010053962247));
#18987=CARTESIAN_POINT('Ctrl Pts',(-1.09768999241225,-1.,1.74354119236208));
#18988=CARTESIAN_POINT('Ctrl Pts',(-1.10286118991143,-1.,1.74695004214923));
#18989=CARTESIAN_POINT('Ctrl Pts',(-1.10806728183007,-1.,1.7503286607592));
#18990=CARTESIAN_POINT('Ctrl Pts',(-1.11330807582551,-1.,1.7536777209463));
#18991=CARTESIAN_POINT('Ctrl Pts',(-1.11858293216763,-1.,1.75699720772105));
#18992=CARTESIAN_POINT('Ctrl Pts',(-1.12389096855086,-1.,1.76028671825096));
#18993=CARTESIAN_POINT('Ctrl Pts',(-1.12923123555075,-1.,1.7635457196617));
#18994=CARTESIAN_POINT('Ctrl Pts',(-1.1346029180462,-1.,1.76677384551862));
#18995=CARTESIAN_POINT('Ctrl Pts',(-1.14000548336975,-1.,1.76997111386769));
#18996=CARTESIAN_POINT('Ctrl Pts',(-1.1454385822692,-1.,1.77313777896194));
#18997=CARTESIAN_POINT('Ctrl Pts',(-1.15090197841515,-1.,1.7762742255701));
#18998=CARTESIAN_POINT('Ctrl Pts',(-1.15639547194698,-1.,1.77938085564275));
#18999=CARTESIAN_POINT('Ctrl Pts',(-1.16191881298499,-1.,1.78245795881009));
#19000=CARTESIAN_POINT('Ctrl Pts',(-1.16747166312303,-1.,1.78550566040443));
#19001=CARTESIAN_POINT('Ctrl Pts',(-1.17305363177328,-1.,1.78852398877616));
#19002=CARTESIAN_POINT('Ctrl Pts',(-1.17866429440809,-1.,1.79151291552689));
#19003=CARTESIAN_POINT('Ctrl Pts',(-1.18430321697432,-1.,1.79447240321515));
#19004=CARTESIAN_POINT('Ctrl Pts',(-1.18996997934445,-1.,1.79740245923478));
#19005=CARTESIAN_POINT('Ctrl Pts',(-1.19566418930242,-1.,1.80030314369879));
#19006=CARTESIAN_POINT('Ctrl Pts',(-1.20138548938974,-1.,1.80317454838603));
#19007=CARTESIAN_POINT('Ctrl Pts',(-1.20713356605475,-1.,1.80601678480707));
#19008=CARTESIAN_POINT('Ctrl Pts',(-1.21290815708314,-1.,1.80882996917129));
#19009=CARTESIAN_POINT('Ctrl Pts',(-1.21870906103557,-1.,1.81161420806656));
#19010=CARTESIAN_POINT('Ctrl Pts',(-1.2245361330495,-1.,1.81436959210434));
#19011=CARTESIAN_POINT('Ctrl Pts',(-1.2292186489137,-1.,1.8165508718364));
#19012=CARTESIAN_POINT('Ctrl Pts',(-1.2327422452705,-1.,1.81817389921279));
#19013=CARTESIAN_POINT('Ctrl Pts',(-1.23509651170476,-1.,1.81925017193666));
#19014=CARTESIAN_POINT('Ctrl Pts',(-1.23627494547115,-1.,1.81978687191668));
#19015=CARTESIAN_POINT('',(-1.34869019493419,-1.,1.73811241238545));
#19016=CARTESIAN_POINT('',(-1.23627494547115,-1.,1.81978687191668));
#19017=CARTESIAN_POINT('',(-1.15624053661742,-1.,1.31362392696032));
#19018=CARTESIAN_POINT('Ctrl Pts',(-1.34869019493419,-1.,1.73811241238545));
#19019=CARTESIAN_POINT('Ctrl Pts',(-1.34854391898045,-1.,1.73682580585691));
#19020=CARTESIAN_POINT('Ctrl Pts',(-1.34824783112887,-1.,1.73425417885907));
#19021=CARTESIAN_POINT('Ctrl Pts',(-1.34779309152035,-1.,1.7304014965394));
#19022=CARTESIAN_POINT('Ctrl Pts',(-1.34716554819527,-1.,1.72527410680674));
#19023=CARTESIAN_POINT('Ctrl Pts',(-1.34634568653227,-1.,1.7188807715049));
#19024=CARTESIAN_POINT('Ctrl Pts',(-1.34549029589416,-1.,1.71250340686822));
#19025=CARTESIAN_POINT('Ctrl Pts',(-1.34459924533831,-1.,1.70614212266738));
#19026=CARTESIAN_POINT('Ctrl Pts',(-1.34367237124483,-1.,1.69979707754427));
#19027=CARTESIAN_POINT('Ctrl Pts',(-1.34270948206319,-1.,1.6934684849687));
#19028=CARTESIAN_POINT('Ctrl Pts',(-1.341710374848,-1.,1.68715660868764));
#19029=CARTESIAN_POINT('Ctrl Pts',(-1.34067485185203,-1.,1.68086176030362));
#19030=CARTESIAN_POINT('Ctrl Pts',(-1.3396027347034,-1.,1.67458429426086));
#19031=CARTESIAN_POINT('Ctrl Pts',(-1.33849388654388,-1.,1.66832460783989));
#19032=CARTESIAN_POINT('Ctrl Pts',(-1.33734820885262,-1.,1.66208312541983));
#19033=CARTESIAN_POINT('Ctrl Pts',(-1.33616559745172,-1.,1.65586025952593));
#19034=CARTESIAN_POINT('Ctrl Pts',(-1.33494590467993,-1.,1.6496563728683));
#19035=CARTESIAN_POINT('Ctrl Pts',(-1.33368890676572,-1.,1.6434717485603));
#19036=CARTESIAN_POINT('Ctrl Pts',(-1.33239425103724,-1.,1.63730653475089));
#19037=CARTESIAN_POINT('Ctrl Pts',(-1.33106149345645,-1.,1.63116079730923));
#19038=CARTESIAN_POINT('Ctrl Pts',(-1.3296901950568,-1.,1.62503464209797));
#19039=CARTESIAN_POINT('Ctrl Pts',(-1.32828000610449,-1.,1.61892832270724));
#19040=CARTESIAN_POINT('Ctrl Pts',(-1.32683074483356,-1.,1.6128423401575));
#19041=CARTESIAN_POINT('Ctrl Pts',(-1.32534250785782,-1.,1.60677758290954));
#19042=CARTESIAN_POINT('Ctrl Pts',(-1.32381550858256,-1.,1.60073511858687));
#19043=CARTESIAN_POINT('Ctrl Pts',(-1.32224985747682,-1.,1.59471591079403));
#19044=CARTESIAN_POINT('Ctrl Pts',(-1.32064537110892,-1.,1.58872057258245));
#19045=CARTESIAN_POINT('Ctrl Pts',(-1.31900135021432,-1.,1.58274907898834));
#19046=CARTESIAN_POINT('Ctrl Pts',(-1.31731642317187,-1.,1.5768005650559));
#19047=CARTESIAN_POINT('Ctrl Pts',(-1.31558903860016,-1.,1.57087397835723));
#19048=CARTESIAN_POINT('Ctrl Pts',(-1.31381795281002,-1.,1.56496872402353));
#19049=CARTESIAN_POINT('Ctrl Pts',(-1.31200264341696,-1.,1.55908521254821));
#19050=CARTESIAN_POINT('Ctrl Pts',(-1.31014393684222,-1.,1.55322568759481));
#19051=CARTESIAN_POINT('Ctrl Pts',(-1.30824393907473,-1.,1.54739413957185));
#19052=CARTESIAN_POINT('Ctrl Pts',(-1.30630475189556,-1.,1.54159462645432));
#19053=CARTESIAN_POINT('Ctrl Pts',(-1.30432735639489,-1.,1.53582981268977));
#19054=CARTESIAN_POINT('Ctrl Pts',(-1.30231064395568,-1.,1.53009970283891));
#19055=CARTESIAN_POINT('Ctrl Pts',(-1.30024984366328,-1.,1.52439957861062));
#19056=CARTESIAN_POINT('Ctrl Pts',(-1.29813791800747,-1.,1.51872184912724));
#19057=CARTESIAN_POINT('Ctrl Pts',(-1.29596850710509,-1.,1.51305994241402));
#19058=CARTESIAN_POINT('Ctrl Pts',(-1.29373841372842,-1.,1.50741159078365));
#19059=CARTESIAN_POINT('Ctrl Pts',(-1.29145022885181,-1.,1.50178230149776));
#19060=CARTESIAN_POINT('Ctrl Pts',(-1.28911506584254,-1.,1.49618896881754));
#19061=CARTESIAN_POINT('Ctrl Pts',(-1.2867467611644,-1.,1.4906522831278));
#19062=CARTESIAN_POINT('Ctrl Pts',(-1.28435533880201,-1.,1.4851881711891));
#19063=CARTESIAN_POINT('Ctrl Pts',(-1.28194158939517,-1.,1.47980070347095));
#19064=CARTESIAN_POINT('Ctrl Pts',(-1.2794891824849,-1.,1.4744717526707));
#19065=CARTESIAN_POINT('Ctrl Pts',(-1.27696414831089,-1.,1.46916035917133));
#19066=CARTESIAN_POINT('Ctrl Pts',(-1.27433119897822,-1.,1.46382431332476));
#19067=CARTESIAN_POINT('Ctrl Pts',(-1.27156805265289,-1.,1.45843906294697));
#19068=CARTESIAN_POINT('Ctrl Pts',(-1.2686778680489,-1.,1.45301422764247));
#19069=CARTESIAN_POINT('Ctrl Pts',(-1.26570925118868,-1.,1.44761985001662));
#19070=CARTESIAN_POINT('Ctrl Pts',(-1.26273903323859,-1.,1.44236470511303));
#19071=CARTESIAN_POINT('Ctrl Pts',(-1.25983531012005,-1.,1.43734919180848));
#19072=CARTESIAN_POINT('Ctrl Pts',(-1.25702687965755,-1.,1.43262645609691));
#19073=CARTESIAN_POINT('Ctrl Pts',(-1.25426945222639,-1.,1.42815938799387));
#19074=CARTESIAN_POINT('Ctrl Pts',(-1.2514145557001,-1.,1.42378102115575));
#19075=CARTESIAN_POINT('Ctrl Pts',(-1.24824430986571,-1.,1.41923722596025));
#19076=CARTESIAN_POINT('Ctrl Pts',(-1.24450600513056,-1.,1.41422913175179));
#19077=CARTESIAN_POINT('Ctrl Pts',(-1.23994455029534,-1.,1.40845295531283));
#19078=CARTESIAN_POINT('Ctrl Pts',(-1.23434087290423,-1.,1.40164708206106));
#19079=CARTESIAN_POINT('Ctrl Pts',(-1.22752961899387,-1.,1.39361389568796));
#19080=CARTESIAN_POINT('Ctrl Pts',(-1.21938737280852,-1.,1.38420564527715));
#19081=CARTESIAN_POINT('Ctrl Pts',(-1.20982812925645,-1.,1.37331915607905));
#19082=CARTESIAN_POINT('Ctrl Pts',(-1.1987959077932,-1.,1.36088705043885));
#19083=CARTESIAN_POINT('Ctrl Pts',(-1.18625865667441,-1.,1.34687054001093));
#19084=CARTESIAN_POINT('Ctrl Pts',(-1.17501305789857,-1.,1.33437539347008));
#19085=CARTESIAN_POINT('Ctrl Pts',(-1.16589330093588,-1.,1.32428080721772));
#19086=CARTESIAN_POINT('Ctrl Pts',(-1.15950888730809,-1.,1.31722977216397));
#19087=CARTESIAN_POINT('Ctrl Pts',(-1.15624053661742,-1.,1.31362392696032));
#19088=CARTESIAN_POINT('',(-1.31362392696033,-1.,1.15624053661742));
#19089=CARTESIAN_POINT('Origin',(0.,-1.,0.));
#19090=CARTESIAN_POINT('',(-1.73811241238545,-1.,1.34869019493419));
#19091=CARTESIAN_POINT('Ctrl Pts',(-1.31362392696033,-1.,1.15624053661742));
#19092=CARTESIAN_POINT('Ctrl Pts',(-1.3172297721596,-1.,1.15950888730433));
#19093=CARTESIAN_POINT('Ctrl Pts',(-1.32428080720544,-1.,1.16589330092532));
#19094=CARTESIAN_POINT('Ctrl Pts',(-1.33437539344842,-1.,1.17501305787994));
#19095=CARTESIAN_POINT('Ctrl Pts',(-1.34687053998157,-1.,1.18625865664915));
#19096=CARTESIAN_POINT('Ctrl Pts',(-1.36088705040677,-1.,1.1987959077656));
#19097=CARTESIAN_POINT('Ctrl Pts',(-1.37331915604962,-1.,1.20982812923113));
#19098=CARTESIAN_POINT('Ctrl Pts',(-1.38420564525391,-1.,1.21938737278853));
#19099=CARTESIAN_POINT('Ctrl Pts',(-1.39361389567257,-1.,1.22752961898063));
#19100=CARTESIAN_POINT('Ctrl Pts',(-1.40164708205345,-1.,1.23434087289768));
#19101=CARTESIAN_POINT('Ctrl Pts',(-1.40845295531151,-1.,1.23994455029421));
#19102=CARTESIAN_POINT('Ctrl Pts',(-1.41422913175437,-1.,1.24450600513278));
#19103=CARTESIAN_POINT('Ctrl Pts',(-1.41923722596421,-1.,1.24824430986911));
#19104=CARTESIAN_POINT('Ctrl Pts',(-1.42378102115911,-1.,1.25141455570299));
#19105=CARTESIAN_POINT('Ctrl Pts',(-1.42815938799555,-1.,1.25426945222783));
#19106=CARTESIAN_POINT('Ctrl Pts',(-1.43262645609679,-1.,1.25702687965744));
#19107=CARTESIAN_POINT('Ctrl Pts',(-1.43734919180719,-1.,1.25983531011894));
#19108=CARTESIAN_POINT('Ctrl Pts',(-1.44236470511145,-1.,1.26273903323723));
#19109=CARTESIAN_POINT('Ctrl Pts',(-1.44761985001544,-1.,1.26570925118767));
#19110=CARTESIAN_POINT('Ctrl Pts',(-1.45301422764205,-1.,1.26867786804854));
#19111=CARTESIAN_POINT('Ctrl Pts',(-1.45843906294725,-1.,1.27156805265312));
#19112=CARTESIAN_POINT('Ctrl Pts',(-1.4638243133254,-1.,1.27433119897877));
#19113=CARTESIAN_POINT('Ctrl Pts',(-1.46916035917197,-1.,1.27696414831144));
#19114=CARTESIAN_POINT('Ctrl Pts',(-1.4744717526711,-1.,1.27948918248524));
#19115=CARTESIAN_POINT('Ctrl Pts',(-1.47980070347102,-1.,1.28194158939522));
#19116=CARTESIAN_POINT('Ctrl Pts',(-1.48518817118891,-1.,1.28435533880184));
#19117=CARTESIAN_POINT('Ctrl Pts',(-1.4906522831275,-1.,1.28674676116415));
#19118=CARTESIAN_POINT('Ctrl Pts',(-1.49618896881729,-1.,1.28911506584232));
#19119=CARTESIAN_POINT('Ctrl Pts',(-1.50178230149764,-1.,1.29145022885171));
#19120=CARTESIAN_POINT('Ctrl Pts',(-1.50741159078367,-1.,1.29373841372843));
#19121=CARTESIAN_POINT('Ctrl Pts',(-1.51305994241412,-1.,1.29596850710518));
#19122=CARTESIAN_POINT('Ctrl Pts',(-1.51872184912735,-1.,1.29813791800757));
#19123=CARTESIAN_POINT('Ctrl Pts',(-1.5243995786107,-1.,1.30024984366334));
#19124=CARTESIAN_POINT('Ctrl Pts',(-1.53009970283893,-1.,1.3023106439557));
#19125=CARTESIAN_POINT('Ctrl Pts',(-1.53582981268976,-1.,1.30432735639487));
#19126=CARTESIAN_POINT('Ctrl Pts',(-1.54159462645428,-1.,1.30630475189553));
#19127=CARTESIAN_POINT('Ctrl Pts',(-1.54739413957183,-1.,1.30824393907471));
#19128=CARTESIAN_POINT('Ctrl Pts',(-1.55322568759481,-1.,1.31014393684221));
#19129=CARTESIAN_POINT('Ctrl Pts',(-1.55908521254822,-1.,1.31200264341696));
#19130=CARTESIAN_POINT('Ctrl Pts',(-1.56496872402352,-1.,1.31381795281002));
#19131=CARTESIAN_POINT('Ctrl Pts',(-1.57087397835721,-1.,1.31558903860015));
#19132=CARTESIAN_POINT('Ctrl Pts',(-1.57680056505585,-1.,1.31731642317183));
#19133=CARTESIAN_POINT('Ctrl Pts',(-1.58274907898829,-1.,1.31900135021428));
#19134=CARTESIAN_POINT('Ctrl Pts',(-1.58872057258244,-1.,1.32064537110891));
#19135=CARTESIAN_POINT('Ctrl Pts',(-1.59471591079408,-1.,1.32224985747686));
#19136=CARTESIAN_POINT('Ctrl Pts',(-1.600735118587,-1.,1.32381550858266));
#19137=CARTESIAN_POINT('Ctrl Pts',(-1.6067775829097,-1.,1.32534250785794));
#19138=CARTESIAN_POINT('Ctrl Pts',(-1.61284234015762,-1.,1.32683074483365));
#19139=CARTESIAN_POINT('Ctrl Pts',(-1.61892832270723,-1.,1.32828000610448));
#19140=CARTESIAN_POINT('Ctrl Pts',(-1.62503464209777,-1.,1.32969019505665));
#19141=CARTESIAN_POINT('Ctrl Pts',(-1.63116079730887,-1.,1.33106149345618));
#19142=CARTESIAN_POINT('Ctrl Pts',(-1.6373065347505,-1.,1.33239425103694));
#19143=CARTESIAN_POINT('Ctrl Pts',(-1.64347174856007,-1.,1.33368890676554));
#19144=CARTESIAN_POINT('Ctrl Pts',(-1.64965637286843,-1.,1.33494590468003));
#19145=CARTESIAN_POINT('Ctrl Pts',(-1.65586025952651,-1.,1.33616559745217));
#19146=CARTESIAN_POINT('Ctrl Pts',(-1.66208312542073,-1.,1.33734820885331));
#19147=CARTESIAN_POINT('Ctrl Pts',(-1.66832460784078,-1.,1.33849388654458));
#19148=CARTESIAN_POINT('Ctrl Pts',(-1.67458429426126,-1.,1.33960273470372));
#19149=CARTESIAN_POINT('Ctrl Pts',(-1.68086176030308,-1.,1.3406748518516));
#19150=CARTESIAN_POINT('Ctrl Pts',(-1.68715660868602,-1.,1.34171037484673));
#19151=CARTESIAN_POINT('Ctrl Pts',(-1.6934684849664,-1.,1.34270948206139));
#19152=CARTESIAN_POINT('Ctrl Pts',(-1.69979707754221,-1.,1.34367237124322));
#19153=CARTESIAN_POINT('Ctrl Pts',(-1.70614212266676,-1.,1.34459924533783));
#19154=CARTESIAN_POINT('Ctrl Pts',(-1.71250340687011,-1.,1.34549029589563));
#19155=CARTESIAN_POINT('Ctrl Pts',(-1.7188807715095,-1.,1.34634568653586));
#19156=CARTESIAN_POINT('Ctrl Pts',(-1.72527410681298,-1.,1.34716554820013));
#19157=CARTESIAN_POINT('Ctrl Pts',(-1.73040149654497,-1.,1.3477930915247));
#19158=CARTESIAN_POINT('Ctrl Pts',(-1.73425417886255,-1.,1.34824783113158));
#19159=CARTESIAN_POINT('Ctrl Pts',(-1.73682580585819,-1.,1.34854391898145));
#19160=CARTESIAN_POINT('Ctrl Pts',(-1.73811241238545,-1.,1.34869019493419));
#19161=CARTESIAN_POINT('',(-1.81978687191668,-1.,1.23627494547115));
#19162=CARTESIAN_POINT('',(-1.73811241238545,-1.,1.34869019493419));
#19163=CARTESIAN_POINT('',(-1.5055822144029,-1.,0.892032620296855));
#19164=CARTESIAN_POINT('Ctrl Pts',(-1.81978687191668,-1.,1.23627494547115));
#19165=CARTESIAN_POINT('Ctrl Pts',(-1.81925017193531,-1.,1.23509651170384));
#19166=CARTESIAN_POINT('Ctrl Pts',(-1.81817389920914,-1.,1.23274224526804));
#19167=CARTESIAN_POINT('Ctrl Pts',(-1.81655087183054,-1.,1.22921864890975));
#19168=CARTESIAN_POINT('Ctrl Pts',(-1.81436959209778,-1.,1.22453613304507));
#19169=CARTESIAN_POINT('Ctrl Pts',(-1.81161420806172,-1.,1.2187090610323));
#19170=CARTESIAN_POINT('Ctrl Pts',(-1.80882996916931,-1.,1.2129081570818));
#19171=CARTESIAN_POINT('Ctrl Pts',(-1.80601678480772,-1.,1.20713356605519));
#19172=CARTESIAN_POINT('Ctrl Pts',(-1.8031745483882,-1.,1.2013854893912));
#19173=CARTESIAN_POINT('Ctrl Pts',(-1.80030314370121,-1.,1.19566418930405));
#19174=CARTESIAN_POINT('Ctrl Pts',(-1.79740245923649,-1.,1.1899699793456));
#19175=CARTESIAN_POINT('Ctrl Pts',(-1.79447240321572,-1.,1.18430321697471));
#19176=CARTESIAN_POINT('Ctrl Pts',(-1.79151291552646,-1.,1.17866429440781));
#19177=CARTESIAN_POINT('Ctrl Pts',(-1.78852398877523,-1.,1.17305363177265));
#19178=CARTESIAN_POINT('Ctrl Pts',(-1.78550566040349,-1.,1.16747166312239));
#19179=CARTESIAN_POINT('Ctrl Pts',(-1.78245795880949,-1.,1.16191881298458));
#19180=CARTESIAN_POINT('Ctrl Pts',(-1.77938085564261,-1.,1.15639547194689));
#19181=CARTESIAN_POINT('Ctrl Pts',(-1.77627422557034,-1.,1.15090197841531));
#19182=CARTESIAN_POINT('Ctrl Pts',(-1.77313777896234,-1.,1.14543858226948));
#19183=CARTESIAN_POINT('Ctrl Pts',(-1.76997111386806,-1.,1.14000548337));
#19184=CARTESIAN_POINT('Ctrl Pts',(-1.76677384551883,-1.,1.13460291804635));
#19185=CARTESIAN_POINT('Ctrl Pts',(-1.76354571966171,-1.,1.12923123555076));
#19186=CARTESIAN_POINT('Ctrl Pts',(-1.76028671825084,-1.,1.12389096855078));
#19187=CARTESIAN_POINT('Ctrl Pts',(-1.75699720772089,-1.,1.11858293216752));
#19188=CARTESIAN_POINT('Ctrl Pts',(-1.75367772094617,-1.,1.11330807582542));
#19189=CARTESIAN_POINT('Ctrl Pts',(-1.75032866075914,-1.,1.10806728183003));
#19190=CARTESIAN_POINT('Ctrl Pts',(-1.74695004214924,-1.,1.10286118991144));
#19191=CARTESIAN_POINT('Ctrl Pts',(-1.74354119236212,-1.,1.09768999241229));
#19192=CARTESIAN_POINT('Ctrl Pts',(-1.74010053962252,-1.,1.09255329056496));
#19193=CARTESIAN_POINT('Ctrl Pts',(-1.73662628326093,-1.,1.08745056285429));
#19194=CARTESIAN_POINT('Ctrl Pts',(-1.73311705663407,-1.,1.08238162784749));
#19195=CARTESIAN_POINT('Ctrl Pts',(-1.72957248977424,-1.,1.0773470373727));
#19196=CARTESIAN_POINT('Ctrl Pts',(-1.72599406198489,-1.,1.07234866990252));
#19197=CARTESIAN_POINT('Ctrl Pts',(-1.72238500928456,-1.,1.06738966975463));
#19198=CARTESIAN_POINT('Ctrl Pts',(-1.71874858456908,-1.,1.0624732468065));
#19199=CARTESIAN_POINT('Ctrl Pts',(-1.71508654427022,-1.,1.05760163192481));
#19200=CARTESIAN_POINT('Ctrl Pts',(-1.71139783543986,-1.,1.05277517202854));
#19201=CARTESIAN_POINT('Ctrl Pts',(-1.70767646263641,-1.,1.0479908540499));
#19202=CARTESIAN_POINT('Ctrl Pts',(-1.70391338707969,-1.,1.04324363334546));
#19203=CARTESIAN_POINT('Ctrl Pts',(-1.70010052930951,-1.,1.03852922490782));
#19204=CARTESIAN_POINT('Ctrl Pts',(-1.69623414782769,-1.,1.03384646003587));
#19205=CARTESIAN_POINT('Ctrl Pts',(-1.69231840863471,-1.,1.02919977579155));
#19206=CARTESIAN_POINT('Ctrl Pts',(-1.68836910178475,-1.,1.02460180535272));
#19207=CARTESIAN_POINT('Ctrl Pts',(-1.68440578021739,-1.,1.02006795074222));
#19208=CARTESIAN_POINT('Ctrl Pts',(-1.6804428989482,-1.,1.01561026162787));
#19209=CARTESIAN_POINT('Ctrl Pts',(-1.67648246776457,-1.,1.01123236493507));
#19210=CARTESIAN_POINT('Ctrl Pts',(-1.67250335383248,-1.,1.00692206696387));
#19211=CARTESIAN_POINT('Ctrl Pts',(-1.66846059277231,-1.,1.00265091003682));
#19212=CARTESIAN_POINT('Ctrl Pts',(-1.66430758030304,-1.,0.998389654952317));
#19213=CARTESIAN_POINT('Ctrl Pts',(-1.66001553809916,-1.,0.994121836661116));
#19214=CARTESIAN_POINT('Ctrl Pts',(-1.65559044289746,-1.,0.98985562785445));
#19215=CARTESIAN_POINT('Ctrl Pts',(-1.6511001661277,-1.,0.985642622921626));
#19216=CARTESIAN_POINT('Ctrl Pts',(-1.64665139190834,-1.,0.981562530940574));
#19217=CARTESIAN_POINT('Ctrl Pts',(-1.64233990826831,-1.,0.977689794120297));
#19218=CARTESIAN_POINT('Ctrl Pts',(-1.63820952658157,-1.,0.974066058287501));
#19219=CARTESIAN_POINT('Ctrl Pts',(-1.63420665729609,-1.,0.970669715996356));
#19220=CARTESIAN_POINT('Ctrl Pts',(-1.63013849959083,-1.,0.967387853228041));
#19221=CARTESIAN_POINT('Ctrl Pts',(-1.6257193066974,-1.,0.964046107037821));
#19222=CARTESIAN_POINT('Ctrl Pts',(-1.62061638139929,-1.,0.960438326099958));
#19223=CARTESIAN_POINT('Ctrl Pts',(-1.61449324337233,-1.,0.956354422921573));
#19224=CARTESIAN_POINT('Ctrl Pts',(-1.60706069897794,-1.,0.951613284361248));
#19225=CARTESIAN_POINT('Ctrl Pts',(-1.59810042045408,-1.,0.946078063325796));
#19226=CARTESIAN_POINT('Ctrl Pts',(-1.58744937489796,-1.,0.939646377909319));
#19227=CARTESIAN_POINT('Ctrl Pts',(-1.57499388385561,-1.,0.932246680128849));
#19228=CARTESIAN_POINT('Ctrl Pts',(-1.56065988582509,-1.,0.923832188966322));
#19229=CARTESIAN_POINT('Ctrl Pts',(-1.54440491152808,-1.,0.91437591904658));
#19230=CARTESIAN_POINT('Ctrl Pts',(-1.52984849890434,-1.,0.905967409640499));
#19231=CARTESIAN_POINT('Ctrl Pts',(-1.51805569591479,-1.,0.89918504749193));
#19232=CARTESIAN_POINT('Ctrl Pts',(-1.50980486807181,-1.,0.894452006967538));
#19233=CARTESIAN_POINT('Ctrl Pts',(-1.5055822144029,-1.,0.892032620296855));
#19234=CARTESIAN_POINT('',(-1.60662857109684,-1.,0.693717979106305));
#19235=CARTESIAN_POINT('Origin',(0.,-1.,0.));
#19236=CARTESIAN_POINT('',(-2.0698113262342,-1.,0.7455743247944));
#19237=CARTESIAN_POINT('Ctrl Pts',(-1.60662857109684,-1.,0.693717979106305));
#19238=CARTESIAN_POINT('Ctrl Pts',(-1.61106790957619,-1.,0.69571209787897));
#19239=CARTESIAN_POINT('Ctrl Pts',(-1.61974673471117,-1.,0.699605146398837));
#19240=CARTESIAN_POINT('Ctrl Pts',(-1.6321654166204,-1.,0.705159151977294));
#19241=CARTESIAN_POINT('Ctrl Pts',(-1.64752408828442,-1.,0.711993139340447));
#19242=CARTESIAN_POINT('Ctrl Pts',(-1.66472880551777,-1.,0.71958543378795));
#19243=CARTESIAN_POINT('Ctrl Pts',(-1.67996158451922,-1.,0.726235967982445));
#19244=CARTESIAN_POINT('Ctrl Pts',(-1.69326921972915,-1.,0.731963238685357));
#19245=CARTESIAN_POINT('Ctrl Pts',(-1.70473309004249,-1.,0.736799665716932));
#19246=CARTESIAN_POINT('Ctrl Pts',(-1.71447789751001,-1.,0.74079516202821));
#19247=CARTESIAN_POINT('Ctrl Pts',(-1.72268229916769,-1.,0.744021445433093));
#19248=CARTESIAN_POINT('Ctrl Pts',(-1.72958533647714,-1.,0.746574710097752));
#19249=CARTESIAN_POINT('Ctrl Pts',(-1.7355035168033,-1.,0.74858246295687));
#19250=CARTESIAN_POINT('Ctrl Pts',(-1.74080458267114,-1.,0.750193435981249));
#19251=CARTESIAN_POINT('Ctrl Pts',(-1.74585086852502,-1.,0.751555614164482));
#19252=CARTESIAN_POINT('Ctrl Pts',(-1.75095139468794,-1.,0.752797683531314));
#19253=CARTESIAN_POINT('Ctrl Pts',(-1.75631083600019,-1.,0.754009254027829));
#19254=CARTESIAN_POINT('Ctrl Pts',(-1.76197817240128,-1.,0.755220979974461));
#19255=CARTESIAN_POINT('Ctrl Pts',(-1.76789396002998,-1.,0.75642189602781));
#19256=CARTESIAN_POINT('Ctrl Pts',(-1.77394167108292,-1.,0.757578264077029));
#19257=CARTESIAN_POINT('Ctrl Pts',(-1.77999411220945,-1.,0.758650626677518));
#19258=CARTESIAN_POINT('Ctrl Pts',(-1.78596964884604,-1.,0.759614401110189));
#19259=CARTESIAN_POINT('Ctrl Pts',(-1.7918581561088,-1.,0.760469555880749));
#19260=CARTESIAN_POINT('Ctrl Pts',(-1.79768986997783,-1.,0.761229695230558));
#19261=CARTESIAN_POINT('Ctrl Pts',(-1.80351583877342,-1.,0.761915336443547));
#19262=CARTESIAN_POINT('Ctrl Pts',(-1.80938551463965,-1.,0.762546129463938));
#19263=CARTESIAN_POINT('Ctrl Pts',(-1.8153211840553,-1.,0.763132003836634));
#19264=CARTESIAN_POINT('Ctrl Pts',(-1.82131873145266,-1.,0.763673465462726));
#19265=CARTESIAN_POINT('Ctrl Pts',(-1.82735991200065,-1.,0.764165902605995));
#19266=CARTESIAN_POINT('Ctrl Pts',(-1.83342077227142,-1.,0.764602549687853));
#19267=CARTESIAN_POINT('Ctrl Pts',(-1.83948181064835,-1.,0.764978057881737));
#19268=CARTESIAN_POINT('Ctrl Pts',(-1.84553698875924,-1.,0.765291664862029));
#19269=CARTESIAN_POINT('Ctrl Pts',(-1.85158945130063,-1.,0.765545710619062));
#19270=CARTESIAN_POINT('Ctrl Pts',(-1.85764741390394,-1.,0.765744212909318));
#19271=CARTESIAN_POINT('Ctrl Pts',(-1.86372027063312,-1.,0.765891519092547));
#19272=CARTESIAN_POINT('Ctrl Pts',(-1.86981398314341,-1.,0.765990708546091));
#19273=CARTESIAN_POINT('Ctrl Pts',(-1.87592888967883,-1.,0.766042837036744));
#19274=CARTESIAN_POINT('Ctrl Pts',(-1.88206215302561,-1.,0.766047794851864));
#19275=CARTESIAN_POINT('Ctrl Pts',(-1.88820926433409,-1.,0.766004837062091));
#19276=CARTESIAN_POINT('Ctrl Pts',(-1.89436577771388,-1.,0.765913193856978));
#19277=CARTESIAN_POINT('Ctrl Pts',(-1.90052930393596,-1.,0.765772772593386));
#19278=CARTESIAN_POINT('Ctrl Pts',(-1.90669961402356,-1.,0.765584196937919));
#19279=CARTESIAN_POINT('Ctrl Pts',(-1.91287765805169,-1.,0.765348465884722));
#19280=CARTESIAN_POINT('Ctrl Pts',(-1.91906491634196,-1.,0.765066729667088));
#19281=CARTESIAN_POINT('Ctrl Pts',(-1.92526263537048,-1.,0.764740025488211));
#19282=CARTESIAN_POINT('Ctrl Pts',(-1.93147105496382,-1.,0.76436901067394));
#19283=CARTESIAN_POINT('Ctrl Pts',(-1.93768964875886,-1.,0.763954049121458));
#19284=CARTESIAN_POINT('Ctrl Pts',(-1.9439174661764,-1.,0.763495333538629));
#19285=CARTESIAN_POINT('Ctrl Pts',(-1.95015342590024,-1.,0.762992990878769));
#19286=CARTESIAN_POINT('Ctrl Pts',(-1.95639665309869,-1.,0.762447203806179));
#19287=CARTESIAN_POINT('Ctrl Pts',(-1.96264672744186,-1.,0.761858300014423));
#19288=CARTESIAN_POINT('Ctrl Pts',(-1.96890351582499,-1.,0.76122669048382));
#19289=CARTESIAN_POINT('Ctrl Pts',(-1.97516705321494,-1.,0.760552825409757));
#19290=CARTESIAN_POINT('Ctrl Pts',(-1.98143741418172,-1.,0.75983714745219));
#19291=CARTESIAN_POINT('Ctrl Pts',(-1.98771456680874,-1.,0.759080037802488));
#19292=CARTESIAN_POINT('Ctrl Pts',(-1.99399831098817,-1.,0.758281796766761));
#19293=CARTESIAN_POINT('Ctrl Pts',(-2.00028834739178,-1.,0.757442676862724));
#19294=CARTESIAN_POINT('Ctrl Pts',(-2.0065843158773,-1.,0.75656290464667));
#19295=CARTESIAN_POINT('Ctrl Pts',(-2.01288584328084,-1.,0.755642704957865));
#19296=CARTESIAN_POINT('Ctrl Pts',(-2.01919259405809,-1.,0.754682330722816));
#19297=CARTESIAN_POINT('Ctrl Pts',(-2.02550428623313,-1.,0.753682061112768));
#19298=CARTESIAN_POINT('Ctrl Pts',(-2.03182068456221,-1.,0.752642180487211));
#19299=CARTESIAN_POINT('Ctrl Pts',(-2.03814160092099,-1.,0.751562963361115));
#19300=CARTESIAN_POINT('Ctrl Pts',(-2.04446689147979,-1.,0.750444657875576));
#19301=CARTESIAN_POINT('Ctrl Pts',(-2.05079645592154,-1.,0.749287468665046));
#19302=CARTESIAN_POINT('Ctrl Pts',(-2.05713023031006,-1.,0.748091554183802));
#19303=CARTESIAN_POINT('Ctrl Pts',(-2.06220058927826,-1.,0.747103932787919));
#19304=CARTESIAN_POINT('Ctrl Pts',(-2.06600523016815,-1.,0.7463458715442));
#19305=CARTESIAN_POINT('Ctrl Pts',(-2.06854248895728,-1.,0.745832791378367));
#19306=CARTESIAN_POINT('Ctrl Pts',(-2.0698113262342,-1.,0.7455743247944));
#19307=CARTESIAN_POINT('',(-2.11275013067528,-1.,0.61342227326009));
#19308=CARTESIAN_POINT('',(-2.0698113262342,-1.,0.7455743247944));
#19309=CARTESIAN_POINT('',(-1.7075470150345,-1.,0.383122945602004));
#19310=CARTESIAN_POINT('Ctrl Pts',(-2.11275013067528,-1.,0.61342227326009));
#19311=CARTESIAN_POINT('Ctrl Pts',(-2.11187554259986,-1.,0.6124673655618));
#19312=CARTESIAN_POINT('Ctrl Pts',(-2.11012443807238,-1.,0.610560911689899));
#19313=CARTESIAN_POINT('Ctrl Pts',(-2.1074919961518,-1.,0.607711315454876));
#19314=CARTESIAN_POINT('Ctrl Pts',(-2.10397049886949,-1.,0.60393203073603));
#19315=CARTESIAN_POINT('Ctrl Pts',(-2.0995493086477,-1.,0.599241616420533));
#19316=CARTESIAN_POINT('Ctrl Pts',(-2.0951087622027,-1.,0.594585006052162));
#19317=CARTESIAN_POINT('Ctrl Pts',(-2.09064881812129,-1.,0.589962365403406));
#19318=CARTESIAN_POINT('Ctrl Pts',(-2.08616943727951,-1.,0.585373918991617));
#19319=CARTESIAN_POINT('Ctrl Pts',(-2.08167059018418,-1.,0.580819952108063));
#19320=CARTESIAN_POINT('Ctrl Pts',(-2.07715226767559,-1.,0.576300797416844));
#19321=CARTESIAN_POINT('Ctrl Pts',(-2.07261449292824,-1.,0.571816823242603));
#19322=CARTESIAN_POINT('Ctrl Pts',(-2.06805732997334,-1.,0.567368421181087));
#19323=CARTESIAN_POINT('Ctrl Pts',(-2.06348090160589,-1.,0.562955993082261));
#19324=CARTESIAN_POINT('Ctrl Pts',(-2.05888537756462,-1.,0.558579940185151));
#19325=CARTESIAN_POINT('Ctrl Pts',(-2.05427091604413,-1.,0.554240657463906));
#19326=CARTESIAN_POINT('Ctrl Pts',(-2.04963761077958,-1.,0.549938525150295));
#19327=CARTESIAN_POINT('Ctrl Pts',(-2.04498544714588,-1.,0.54567390381743));
#19328=CARTESIAN_POINT('Ctrl Pts',(-2.04031422690527,-1.,0.541447120615659));
#19329=CARTESIAN_POINT('Ctrl Pts',(-2.03562362954037,-1.,0.537258489833262));
#19330=CARTESIAN_POINT('Ctrl Pts',(-2.03091336214426,-1.,0.533108355132976));
#19331=CARTESIAN_POINT('Ctrl Pts',(-2.0261832908329,-1.,0.528997127241914));
#19332=CARTESIAN_POINT('Ctrl Pts',(-2.02143356304698,-1.,0.524925318333476));
#19333=CARTESIAN_POINT('Ctrl Pts',(-2.01666477917286,-1.,0.52089359039937));
#19334=CARTESIAN_POINT('Ctrl Pts',(-2.01187773939242,-1.,0.516902681728687));
#19335=CARTESIAN_POINT('Ctrl Pts',(-2.00707309946949,-1.,0.512953306961792));
#19336=CARTESIAN_POINT('Ctrl Pts',(-2.00225107134734,-1.,0.509046069886157));
#19337=CARTESIAN_POINT('Ctrl Pts',(-1.99741107463572,-1.,0.505181361323026));
#19338=CARTESIAN_POINT('Ctrl Pts',(-1.99255149126155,-1.,0.501359287727146));
#19339=CARTESIAN_POINT('Ctrl Pts',(-1.98767044752932,-1.,0.497579909545574));
#19340=CARTESIAN_POINT('Ctrl Pts',(-1.98276658761821,-1.,0.493843476541494));
#19341=CARTESIAN_POINT('Ctrl Pts',(-1.97783973019229,-1.,0.490150627860952));
#19342=CARTESIAN_POINT('Ctrl Pts',(-1.97289186263272,-1.,0.486502692907659));
#19343=CARTESIAN_POINT('Ctrl Pts',(-1.96792703422362,-1.,0.48290166212069));
#19344=CARTESIAN_POINT('Ctrl Pts',(-1.96294933055943,-1.,0.479349583074855));
#19345=CARTESIAN_POINT('Ctrl Pts',(-1.95796111148177,-1.,0.475848034683176));
#19346=CARTESIAN_POINT('Ctrl Pts',(-1.95296148278133,-1.,0.472397672264072));
#19347=CARTESIAN_POINT('Ctrl Pts',(-1.94794381136514,-1.,0.468997482913135));
#19348=CARTESIAN_POINT('Ctrl Pts',(-1.9428979419619,-1.,0.46564546202603));
#19349=CARTESIAN_POINT('Ctrl Pts',(-1.93781486640821,-1.,0.462340031009056));
#19350=CARTESIAN_POINT('Ctrl Pts',(-1.93269066517934,-1.,0.459081234547926));
#19351=CARTESIAN_POINT('Ctrl Pts',(-1.92753067150476,-1.,0.455872005174371));
#19352=CARTESIAN_POINT('Ctrl Pts',(-1.92235380648502,-1.,0.452719478359432));
#19353=CARTESIAN_POINT('Ctrl Pts',(-1.91718342555755,-1.,0.449632260106662));
#19354=CARTESIAN_POINT('Ctrl Pts',(-1.9120369998112,-1.,0.446617343485711));
#19355=CARTESIAN_POINT('Ctrl Pts',(-1.90691756144898,-1.,0.44367755684915));
#19356=CARTESIAN_POINT('Ctrl Pts',(-1.90180124389086,-1.,0.440807833704038));
#19357=CARTESIAN_POINT('Ctrl Pts',(-1.89663648956466,-1.,0.437995003948244));
#19358=CARTESIAN_POINT('Ctrl Pts',(-1.89136993975504,-1.,0.435225660963383));
#19359=CARTESIAN_POINT('Ctrl Pts',(-1.88596913666793,-1.,0.432493038548748));
#19360=CARTESIAN_POINT('Ctrl Pts',(-1.88044229001832,-1.,0.429803062482344));
#19361=CARTESIAN_POINT('Ctrl Pts',(-1.87486989291484,-1.,0.427183828519102));
#19362=CARTESIAN_POINT('Ctrl Pts',(-1.86937803944323,-1.,0.424678177291359));
#19363=CARTESIAN_POINT('Ctrl Pts',(-1.86408083334028,-1.,0.422327307418275));
#19364=CARTESIAN_POINT('Ctrl Pts',(-1.85903281096686,-1.,0.420157287975619));
#19365=CARTESIAN_POINT('Ctrl Pts',(-1.85417632856234,-1.,0.418164129143534));
#19366=CARTESIAN_POINT('Ctrl Pts',(-1.84929312929882,-1.,0.416300022038864));
#19367=CARTESIAN_POINT('Ctrl Pts',(-1.8440575707371,-1.,0.41448743825434));
#19368=CARTESIAN_POINT('Ctrl Pts',(-1.83808953475839,-1.,0.412633125322161));
#19369=CARTESIAN_POINT('Ctrl Pts',(-1.83100408895216,-1.,0.410641256301675));
#19370=CARTESIAN_POINT('Ctrl Pts',(-1.8224702267854,-1.,0.408428948108533));
#19371=CARTESIAN_POINT('Ctrl Pts',(-1.81223801813988,-1.,0.405933518411838));
#19372=CARTESIAN_POINT('Ctrl Pts',(-1.80012077176221,-1.,0.403107976170441));
#19373=CARTESIAN_POINT('Ctrl Pts',(-1.78598826347533,-1.,0.39991940378308));
#19374=CARTESIAN_POINT('Ctrl Pts',(-1.7697556004756,-1.,0.39634619612042));
#19375=CARTESIAN_POINT('Ctrl Pts',(-1.75137405313962,-1.,0.392375812294307));
#19376=CARTESIAN_POINT('Ctrl Pts',(-1.7349317097561,-1.,0.388877023509191));
#19377=CARTESIAN_POINT('Ctrl Pts',(-1.72162022246158,-1.,0.38607079032701));
#19378=CARTESIAN_POINT('Ctrl Pts',(-1.71231062891958,-1.,0.384119047315542));
#19379=CARTESIAN_POINT('Ctrl Pts',(-1.7075470150345,-1.,0.383122945602004));
#19380=CARTESIAN_POINT('',(-1.74236521665491,-1.,0.163289472382896));
#19381=CARTESIAN_POINT('Origin',(0.,-1.,0.));
#19382=CARTESIAN_POINT('',(-2.19890268624765,-1.,0.069476445021958));
#19383=CARTESIAN_POINT('Ctrl Pts',(-1.74236521665491,-1.,0.163289472382896));
#19384=CARTESIAN_POINT('Ctrl Pts',(-1.7472034950333,-1.,0.163814161002002));
#19385=CARTESIAN_POINT('Ctrl Pts',(-1.75666056638427,-1.,0.164834765707158));
#19386=CARTESIAN_POINT('Ctrl Pts',(-1.77018771684844,-1.,0.1662793551464));
#19387=CARTESIAN_POINT('Ctrl Pts',(-1.7869064998507,-1.,0.168032772805197));
#19388=CARTESIAN_POINT('Ctrl Pts',(-1.80561530629706,-1.,0.169936923904608));
#19389=CARTESIAN_POINT('Ctrl Pts',(-1.82215766811545,-1.,0.171554770204119));
#19390=CARTESIAN_POINT('Ctrl Pts',(-1.83658380527692,-1.,0.1728894428919));
#19391=CARTESIAN_POINT('Ctrl Pts',(-1.8489811319852,-1.,0.173946627587731));
#19392=CARTESIAN_POINT('Ctrl Pts',(-1.85948367088837,-1.,0.17473525927603));
#19393=CARTESIAN_POINT('Ctrl Pts',(-1.86828349694799,-1.,0.175268337590758));
#19394=CARTESIAN_POINT('Ctrl Pts',(-1.87563767773588,-1.,0.175563480746485));
#19395=CARTESIAN_POINT('Ctrl Pts',(-1.88188663145367,-1.,0.175644148889698));
#19396=CARTESIAN_POINT('Ctrl Pts',(-1.88742606273259,-1.,0.175538155840648));
#19397=CARTESIAN_POINT('Ctrl Pts',(-1.892646301985,-1.,0.175274276190844));
#19398=CARTESIAN_POINT('Ctrl Pts',(-1.89788101117132,-1.,0.174879405091263));
#19399=CARTESIAN_POINT('Ctrl Pts',(-1.90335253862834,-1.,0.174375518661085));
#19400=CARTESIAN_POINT('Ctrl Pts',(-1.90911693975267,-1.,0.173776635257817));
#19401=CARTESIAN_POINT('Ctrl Pts',(-1.91511429159527,-1.,0.173090695383496));
#19402=CARTESIAN_POINT('Ctrl Pts',(-1.9212233439798,-1.,0.172321621259514));
#19403=CARTESIAN_POINT('Ctrl Pts',(-1.92731093582036,-1.,0.171471191532988));
#19404=CARTESIAN_POINT('Ctrl Pts',(-1.93329183155539,-1.,0.170541253116201));
#19405=CARTESIAN_POINT('Ctrl Pts',(-1.93915639211581,-1.,0.169534904817491));
#19406=CARTESIAN_POINT('Ctrl Pts',(-1.94493757756931,-1.,0.168455741607556));
#19407=CARTESIAN_POINT('Ctrl Pts',(-1.95069027794294,-1.,0.167307501784475));
#19408=CARTESIAN_POINT('Ctrl Pts',(-1.9564675971873,-1.,0.166093592002812));
#19409=CARTESIAN_POINT('Ctrl Pts',(-1.96229379940136,-1.,0.164816568920269));
#19410=CARTESIAN_POINT('Ctrl Pts',(-1.96816512677967,-1.,0.163478185457734));
#19411=CARTESIAN_POINT('Ctrl Pts',(-1.97406280235188,-1.,0.162079693556288));
#19412=CARTESIAN_POINT('Ctrl Pts',(-1.97996195437559,-1.,0.160622060784611));
#19413=CARTESIAN_POINT('Ctrl Pts',(-1.98584238283292,-1.,0.159106226437299));
#19414=CARTESIAN_POINT('Ctrl Pts',(-1.99169810931908,-1.,0.157533331459227));
#19415=CARTESIAN_POINT('Ctrl Pts',(-1.99753284771497,-1.,0.155904629548783));
#19416=CARTESIAN_POINT('Ctrl Pts',(-2.00335565310543,-1.,0.154221403049722));
#19417=CARTESIAN_POINT('Ctrl Pts',(-2.00917680318424,-1.,0.15248488362145));
#19418=CARTESIAN_POINT('Ctrl Pts',(-2.01500291940238,-1.,0.150696157673078));
#19419=CARTESIAN_POINT('Ctrl Pts',(-2.02083464969894,-1.,0.148856124775337));
#19420=CARTESIAN_POINT('Ctrl Pts',(-2.02666926182017,-1.,0.146965557332583));
#19421=CARTESIAN_POINT('Ctrl Pts',(-2.03250223739942,-1.,0.145025140186057));
#19422=CARTESIAN_POINT('Ctrl Pts',(-2.03832911025912,-1.,0.143035515058209));
#19423=CARTESIAN_POINT('Ctrl Pts',(-2.04414757947916,-1.,0.140997332152546));
#19424=CARTESIAN_POINT('Ctrl Pts',(-2.04995762001328,-1.,0.138911255368966));
#19425=CARTESIAN_POINT('Ctrl Pts',(-2.05576044414264,-1.,0.136777941218043));
#19426=CARTESIAN_POINT('Ctrl Pts',(-2.06155781517842,-1.,0.134598026192106));
#19427=CARTESIAN_POINT('Ctrl Pts',(-2.06735123910326,-1.,0.13237211154771));
#19428=CARTESIAN_POINT('Ctrl Pts',(-2.07314114713063,-1.,0.130100748328403));
#19429=CARTESIAN_POINT('Ctrl Pts',(-2.07892715110987,-1.,0.12778444527612));
#19430=CARTESIAN_POINT('Ctrl Pts',(-2.08470840653643,-1.,0.125423679412061));
#19431=CARTESIAN_POINT('Ctrl Pts',(-2.09048392424825,-1.,0.123018905621083));
#19432=CARTESIAN_POINT('Ctrl Pts',(-2.0962529286773,-1.,0.120570567965122));
#19433=CARTESIAN_POINT('Ctrl Pts',(-2.102015121329,-1.,0.118079107988355));
#19434=CARTESIAN_POINT('Ctrl Pts',(-2.10777050261309,-1.,0.115544957687926));
#19435=CARTESIAN_POINT('Ctrl Pts',(-2.11351924490306,-1.,0.112968534419737));
#19436=CARTESIAN_POINT('Ctrl Pts',(-2.11926155590865,-1.,0.110350236135025));
#19437=CARTESIAN_POINT('Ctrl Pts',(-2.12499752307,-1.,0.10769043523109));
#19438=CARTESIAN_POINT('Ctrl Pts',(-2.13072704887293,-1.,0.104989479152739));
#19439=CARTESIAN_POINT('Ctrl Pts',(-2.13644992667165,-1.,0.1022477005561));
#19440=CARTESIAN_POINT('Ctrl Pts',(-2.14216588396025,-1.,0.0994654261990914));
#19441=CARTESIAN_POINT('Ctrl Pts',(-2.14787463531795,-1.,0.0966429852305457));
#19442=CARTESIAN_POINT('Ctrl Pts',(-2.1535759397817,-1.,0.0937807218867642));
#19443=CARTESIAN_POINT('Ctrl Pts',(-2.15926961544516,-1.,0.0908789888107264));
#19444=CARTESIAN_POINT('Ctrl Pts',(-2.16495552645014,-1.,0.0879381291386921));
#19445=CARTESIAN_POINT('Ctrl Pts',(-2.17063357870952,-1.,0.0849584620835371));
#19446=CARTESIAN_POINT('Ctrl Pts',(-2.176303712113,-1.,0.0819402680872764));
#19447=CARTESIAN_POINT('Ctrl Pts',(-2.18196589448887,-1.,0.0788837727685241));
#19448=CARTESIAN_POINT('Ctrl Pts',(-2.1876201139953,-1.,0.0757891465836146));
#19449=CARTESIAN_POINT('Ctrl Pts',(-2.19213712013662,-1.,0.0732830357306724));
#19450=CARTESIAN_POINT('Ctrl Pts',(-2.19552129484002,-1.,0.0713863779526153));
#19451=CARTESIAN_POINT('Ctrl Pts',(-2.19777582085423,-1.,0.0701143536325489));
#19452=CARTESIAN_POINT('Ctrl Pts',(-2.19890268624765,-1.,0.069476445021958));
#19453=CARTESIAN_POINT('',(-2.19890268624765,-1.,-0.0694764450219585));
#19454=CARTESIAN_POINT('',(-2.19890268624765,-1.,0.069476445021958));
#19455=CARTESIAN_POINT('',(-1.74236521665491,-1.,-0.163289472382896));
#19456=CARTESIAN_POINT('Ctrl Pts',(-2.19890268624765,-1.,-0.0694764450219585));
#19457=CARTESIAN_POINT('Ctrl Pts',(-2.19777582085261,-1.,-0.0701143536324927));
#19458=CARTESIAN_POINT('Ctrl Pts',(-2.19552129483562,-1.,-0.0713863779524629));
#19459=CARTESIAN_POINT('Ctrl Pts',(-2.19213712012956,-1.,-0.0732830357304277));
#19460=CARTESIAN_POINT('Ctrl Pts',(-2.1876201139874,-1.,-0.0757891465833413));
#19461=CARTESIAN_POINT('Ctrl Pts',(-2.18196589448304,-1.,-0.0788837727683229));
#19462=CARTESIAN_POINT('Ctrl Pts',(-2.1763037121106,-1.,-0.0819402680871941));
#19463=CARTESIAN_POINT('Ctrl Pts',(-2.17063357871031,-1.,-0.0849584620835644));
#19464=CARTESIAN_POINT('Ctrl Pts',(-2.16495552645275,-1.,-0.0879381291387824));
#19465=CARTESIAN_POINT('Ctrl Pts',(-2.15926961544808,-1.,-0.0908789888108267));
#19466=CARTESIAN_POINT('Ctrl Pts',(-2.15357593978377,-1.,-0.0937807218868346));
#19467=CARTESIAN_POINT('Ctrl Pts',(-2.14787463531864,-1.,-0.096642985230569));
#19468=CARTESIAN_POINT('Ctrl Pts',(-2.14216588395974,-1.,-0.0994654261990744));
#19469=CARTESIAN_POINT('Ctrl Pts',(-2.13644992667052,-1.,-0.102247700556064));
#19470=CARTESIAN_POINT('Ctrl Pts',(-2.1307270488718,-1.,-0.104989479152703));
#19471=CARTESIAN_POINT('Ctrl Pts',(-2.12499752306927,-1.,-0.107690435231068));
#19472=CARTESIAN_POINT('Ctrl Pts',(-2.11926155590849,-1.,-0.11035023613502));
#19473=CARTESIAN_POINT('Ctrl Pts',(-2.11351924490335,-1.,-0.112968534419746));
#19474=CARTESIAN_POINT('Ctrl Pts',(-2.10777050261359,-1.,-0.11554495768794));
#19475=CARTESIAN_POINT('Ctrl Pts',(-2.10201512132945,-1.,-0.118079107988368));
#19476=CARTESIAN_POINT('Ctrl Pts',(-2.09625292867756,-1.,-0.120570567965129));
#19477=CARTESIAN_POINT('Ctrl Pts',(-2.09048392424826,-1.,-0.123018905621083));
#19478=CARTESIAN_POINT('Ctrl Pts',(-2.08470840653628,-1.,-0.125423679412058));
#19479=CARTESIAN_POINT('Ctrl Pts',(-2.07892715110967,-1.,-0.127784445276116));
#19480=CARTESIAN_POINT('Ctrl Pts',(-2.07314114713047,-1.,-0.130100748328401));
#19481=CARTESIAN_POINT('Ctrl Pts',(-2.06735123910319,-1.,-0.13237211154771));
#19482=CARTESIAN_POINT('Ctrl Pts',(-2.06155781517844,-1.,-0.134598026192107));
#19483=CARTESIAN_POINT('Ctrl Pts',(-2.0557604441427,-1.,-0.136777941218044));
#19484=CARTESIAN_POINT('Ctrl Pts',(-2.04995762001333,-1.,-0.138911255368966));
#19485=CARTESIAN_POINT('Ctrl Pts',(-2.04414757947919,-1.,-0.140997332152545));
#19486=CARTESIAN_POINT('Ctrl Pts',(-2.03832911025913,-1.,-0.143035515058208));
#19487=CARTESIAN_POINT('Ctrl Pts',(-2.03250223739941,-1.,-0.145025140186058));
#19488=CARTESIAN_POINT('Ctrl Pts',(-2.02666926182017,-1.,-0.146965557332586));
#19489=CARTESIAN_POINT('Ctrl Pts',(-2.02083464969897,-1.,-0.148856124775343));
#19490=CARTESIAN_POINT('Ctrl Pts',(-2.01500291940243,-1.,-0.150696157673084));
#19491=CARTESIAN_POINT('Ctrl Pts',(-2.00917680318426,-1.,-0.152484883621452));
#19492=CARTESIAN_POINT('Ctrl Pts',(-2.00335565310539,-1.,-0.154221403049719));
#19493=CARTESIAN_POINT('Ctrl Pts',(-1.99753284771487,-1.,-0.155904629548775));
#19494=CARTESIAN_POINT('Ctrl Pts',(-1.99169810931893,-1.,-0.157533331459215));
#19495=CARTESIAN_POINT('Ctrl Pts',(-1.98584238283279,-1.,-0.159106226437289));
#19496=CARTESIAN_POINT('Ctrl Pts',(-1.97996195437557,-1.,-0.16062206078461));
#19497=CARTESIAN_POINT('Ctrl Pts',(-1.97406280235204,-1.,-0.162079693556302));
#19498=CARTESIAN_POINT('Ctrl Pts',(-1.96816512678,-1.,-0.16347818545776));
#19499=CARTESIAN_POINT('Ctrl Pts',(-1.96229379940174,-1.,-0.1648165689203));
#19500=CARTESIAN_POINT('Ctrl Pts',(-1.95646759718755,-1.,-0.166093592002833));
#19501=CARTESIAN_POINT('Ctrl Pts',(-1.95069027794286,-1.,-0.167307501784469));
#19502=CARTESIAN_POINT('Ctrl Pts',(-1.94493757756879,-1.,-0.168455741607516));
#19503=CARTESIAN_POINT('Ctrl Pts',(-1.93915639211497,-1.,-0.169534904817425));
#19504=CARTESIAN_POINT('Ctrl Pts',(-1.93329183155455,-1.,-0.170541253116136));
#19505=CARTESIAN_POINT('Ctrl Pts',(-1.92731093582,-1.,-0.17147119153296));
#19506=CARTESIAN_POINT('Ctrl Pts',(-1.92122334398034,-1.,-0.172321621259557));
#19507=CARTESIAN_POINT('Ctrl Pts',(-1.91511429159681,-1.,-0.173090695383619));
#19508=CARTESIAN_POINT('Ctrl Pts',(-1.90911693975475,-1.,-0.173776635257984));
#19509=CARTESIAN_POINT('Ctrl Pts',(-1.90335253863003,-1.,-0.174375518661222));
#19510=CARTESIAN_POINT('Ctrl Pts',(-1.89788101117148,-1.,-0.174879405091277));
#19511=CARTESIAN_POINT('Ctrl Pts',(-1.89264630198279,-1.,-0.175274276190664));
#19512=CARTESIAN_POINT('Ctrl Pts',(-1.88742606272818,-1.,-0.175538155840286));
#19513=CARTESIAN_POINT('Ctrl Pts',(-1.88188663144846,-1.,-0.175644148889271));
#19514=CARTESIAN_POINT('Ctrl Pts',(-1.87563767773249,-1.,-0.175563480746205));
#19515=CARTESIAN_POINT('Ctrl Pts',(-1.86828349694972,-1.,-0.175268337590901));
#19516=CARTESIAN_POINT('Ctrl Pts',(-1.85948367089838,-1.,-0.174735259276856));
#19517=CARTESIAN_POINT('Ctrl Pts',(-1.84898113200543,-1.,-0.173946627589401));
#19518=CARTESIAN_POINT('Ctrl Pts',(-1.83658380530747,-1.,-0.17288944289442));
#19519=CARTESIAN_POINT('Ctrl Pts',(-1.82215766815414,-1.,-0.171554770207306));
#19520=CARTESIAN_POINT('Ctrl Pts',(-1.80561530633924,-1.,-0.169936923908078));
#19521=CARTESIAN_POINT('Ctrl Pts',(-1.78690649988931,-1.,-0.16803277280837));
#19522=CARTESIAN_POINT('Ctrl Pts',(-1.77018771687692,-1.,-0.166279355148738));
#19523=CARTESIAN_POINT('Ctrl Pts',(-1.75666056640041,-1.,-0.164834765708484));
#19524=CARTESIAN_POINT('Ctrl Pts',(-1.74720349503904,-1.,-0.163814161002474));
#19525=CARTESIAN_POINT('Ctrl Pts',(-1.74236521665491,-1.,-0.163289472382896));
#19526=CARTESIAN_POINT('',(-1.7075470150345,-1.,-0.383122945602004));
#19527=CARTESIAN_POINT('Origin',(0.,-1.,0.));
#19528=CARTESIAN_POINT('',(-2.11275013067528,-1.,-0.61342227326009));
#19529=CARTESIAN_POINT('Ctrl Pts',(-1.7075470150345,-1.,-0.383122945602004));
#19530=CARTESIAN_POINT('Ctrl Pts',(-1.71231062891398,-1.,-0.384119047314215));
#19531=CARTESIAN_POINT('Ctrl Pts',(-1.72162022244582,-1.,-0.386070790323281));
#19532=CARTESIAN_POINT('Ctrl Pts',(-1.73493170972829,-1.,-0.388877023502615));
#19533=CARTESIAN_POINT('Ctrl Pts',(-1.75137405310193,-1.,-0.392375812285395));
#19534=CARTESIAN_POINT('Ctrl Pts',(-1.76975560043442,-1.,-0.396346196110688));
#19535=CARTESIAN_POINT('Ctrl Pts',(-1.78598826343754,-1.,-0.399919403774155));
#19536=CARTESIAN_POINT('Ctrl Pts',(-1.80012077173238,-1.,-0.403107976163396));
#19537=CARTESIAN_POINT('Ctrl Pts',(-1.81223801812013,-1.,-0.405933518407175));
#19538=CARTESIAN_POINT('Ctrl Pts',(-1.82247022677562,-1.,-0.408428948106227));
#19539=CARTESIAN_POINT('Ctrl Pts',(-1.83100408895047,-1.,-0.410641256301276));
#19540=CARTESIAN_POINT('Ctrl Pts',(-1.8380895347617,-1.,-0.412633125322945));
#19541=CARTESIAN_POINT('Ctrl Pts',(-1.84405757074218,-1.,-0.414487438255542));
#19542=CARTESIAN_POINT('Ctrl Pts',(-1.84929312930314,-1.,-0.416300022039885));
#19543=CARTESIAN_POINT('Ctrl Pts',(-1.8541763285645,-1.,-0.418164129144045));
#19544=CARTESIAN_POINT('Ctrl Pts',(-1.8590328109667,-1.,-0.420157287975583));
#19545=CARTESIAN_POINT('Ctrl Pts',(-1.86408083333863,-1.,-0.422327307417884));
#19546=CARTESIAN_POINT('Ctrl Pts',(-1.8693780394412,-1.,-0.424678177290876));
#19547=CARTESIAN_POINT('Ctrl Pts',(-1.87486989291333,-1.,-0.427183828518743));
#19548=CARTESIAN_POINT('Ctrl Pts',(-1.88044229001778,-1.,-0.429803062482217));
#19549=CARTESIAN_POINT('Ctrl Pts',(-1.88596913666828,-1.,-0.432493038548833));
#19550=CARTESIAN_POINT('Ctrl Pts',(-1.89136993975585,-1.,-0.43522566096358));
#19551=CARTESIAN_POINT('Ctrl Pts',(-1.89663648956549,-1.,-0.437995003948443));
#19552=CARTESIAN_POINT('Ctrl Pts',(-1.90180124389137,-1.,-0.44080783370416));
#19553=CARTESIAN_POINT('Ctrl Pts',(-1.90691756144906,-1.,-0.44367755684917));
#19554=CARTESIAN_POINT('Ctrl Pts',(-1.91203699981095,-1.,-0.446617343485651));
#19555=CARTESIAN_POINT('Ctrl Pts',(-1.91718342555717,-1.,-0.449632260106572));
#19556=CARTESIAN_POINT('Ctrl Pts',(-1.9223538064847,-1.,-0.452719478359356));
#19557=CARTESIAN_POINT('Ctrl Pts',(-1.92753067150461,-1.,-0.455872005174335));
#19558=CARTESIAN_POINT('Ctrl Pts',(-1.93269066517936,-1.,-0.459081234547931));
#19559=CARTESIAN_POINT('Ctrl Pts',(-1.93781486640834,-1.,-0.462340031009087));
#19560=CARTESIAN_POINT('Ctrl Pts',(-1.94289794196205,-1.,-0.465645462026064));
#19561=CARTESIAN_POINT('Ctrl Pts',(-1.94794381136524,-1.,-0.468997482913158));
#19562=CARTESIAN_POINT('Ctrl Pts',(-1.95296148278136,-1.,-0.472397672264079));
#19563=CARTESIAN_POINT('Ctrl Pts',(-1.95796111148175,-1.,-0.475848034683171));
#19564=CARTESIAN_POINT('Ctrl Pts',(-1.96294933055938,-1.,-0.479349583074846));
#19565=CARTESIAN_POINT('Ctrl Pts',(-1.96792703422358,-1.,-0.482901662120686));
#19566=CARTESIAN_POINT('Ctrl Pts',(-1.97289186263272,-1.,-0.486502692907661));
#19567=CARTESIAN_POINT('Ctrl Pts',(-1.97783973019229,-1.,-0.490150627860955));
#19568=CARTESIAN_POINT('Ctrl Pts',(-1.9827665876182,-1.,-0.493843476541492));
#19569=CARTESIAN_POINT('Ctrl Pts',(-1.98767044752929,-1.,-0.497579909545564));
#19570=CARTESIAN_POINT('Ctrl Pts',(-1.9925514912615,-1.,-0.501359287727129));
#19571=CARTESIAN_POINT('Ctrl Pts',(-1.99741107463567,-1.,-0.505181361323011));
#19572=CARTESIAN_POINT('Ctrl Pts',(-2.00225107134733,-1.,-0.509046069886152));
#19573=CARTESIAN_POINT('Ctrl Pts',(-2.00707309946955,-1.,-0.512953306961813));
#19574=CARTESIAN_POINT('Ctrl Pts',(-2.01187773939257,-1.,-0.516902681728733));
#19575=CARTESIAN_POINT('Ctrl Pts',(-2.01666477917305,-1.,-0.520893590399428));
#19576=CARTESIAN_POINT('Ctrl Pts',(-2.02143356304712,-1.,-0.524925318333518));
#19577=CARTESIAN_POINT('Ctrl Pts',(-2.02618329083289,-1.,-0.52899712724191));
#19578=CARTESIAN_POINT('Ctrl Pts',(-2.03091336214401,-1.,-0.533108355132905));
#19579=CARTESIAN_POINT('Ctrl Pts',(-2.03562362953993,-1.,-0.537258489833134));
#19580=CARTESIAN_POINT('Ctrl Pts',(-2.0403142269048,-1.,-0.54144712061552));
#19581=CARTESIAN_POINT('Ctrl Pts',(-2.0449854471456,-1.,-0.545673903817348));
#19582=CARTESIAN_POINT('Ctrl Pts',(-2.04963761077974,-1.,-0.549938525150342));
#19583=CARTESIAN_POINT('Ctrl Pts',(-2.05427091604482,-1.,-0.554240657464109));
#19584=CARTESIAN_POINT('Ctrl Pts',(-2.05888537756571,-1.,-0.558579940185467));
#19585=CARTESIAN_POINT('Ctrl Pts',(-2.06348090160697,-1.,-0.562955993082574));
#19586=CARTESIAN_POINT('Ctrl Pts',(-2.06805732997383,-1.,-0.567368421181229));
#19587=CARTESIAN_POINT('Ctrl Pts',(-2.07261449292757,-1.,-0.571816823242411));
#19588=CARTESIAN_POINT('Ctrl Pts',(-2.07715226767361,-1.,-0.576300797416274));
#19589=CARTESIAN_POINT('Ctrl Pts',(-2.08167059018138,-1.,-0.580819952107257));
#19590=CARTESIAN_POINT('Ctrl Pts',(-2.086169437277,-1.,-0.585373918990895));
#19591=CARTESIAN_POINT('Ctrl Pts',(-2.09064881812053,-1.,-0.589962365403189));
#19592=CARTESIAN_POINT('Ctrl Pts',(-2.09510876220501,-1.,-0.594585006052823));
#19593=CARTESIAN_POINT('Ctrl Pts',(-2.09954930865331,-1.,-0.599241616422144));
#19594=CARTESIAN_POINT('Ctrl Pts',(-2.10397049887709,-1.,-0.603932030738212));
#19595=CARTESIAN_POINT('Ctrl Pts',(-2.10749199615859,-1.,-0.607711315456826));
#19596=CARTESIAN_POINT('Ctrl Pts',(-2.11012443807661,-1.,-0.610560911691113));
#19597=CARTESIAN_POINT('Ctrl Pts',(-2.11187554260142,-1.,-0.61246736556225));
#19598=CARTESIAN_POINT('Ctrl Pts',(-2.11275013067528,-1.,-0.61342227326009));
#19599=CARTESIAN_POINT('',(-2.0698113262342,-1.,-0.745574324794401));
#19600=CARTESIAN_POINT('',(-2.11275013067528,-1.,-0.61342227326009));
#19601=CARTESIAN_POINT('',(-1.60662857109684,-1.,-0.693717979106306));
#19602=CARTESIAN_POINT('Ctrl Pts',(-2.0698113262342,-1.,-0.745574324794401));
#19603=CARTESIAN_POINT('Ctrl Pts',(-2.06854248895575,-1.,-0.74583279137781));
#19604=CARTESIAN_POINT('Ctrl Pts',(-2.06600523016401,-1.,-0.746345871542695));
#19605=CARTESIAN_POINT('Ctrl Pts',(-2.06220058927162,-1.,-0.747103932785504));
#19606=CARTESIAN_POINT('Ctrl Pts',(-2.05713023030263,-1.,-0.748091554181101));
#19607=CARTESIAN_POINT('Ctrl Pts',(-2.05079645591606,-1.,-0.749287468663053));
#19608=CARTESIAN_POINT('Ctrl Pts',(-2.04446689147754,-1.,-0.750444657874758));
#19609=CARTESIAN_POINT('Ctrl Pts',(-2.03814160092173,-1.,-0.751562963361383));
#19610=CARTESIAN_POINT('Ctrl Pts',(-2.03182068456467,-1.,-0.752642180488104));
#19611=CARTESIAN_POINT('Ctrl Pts',(-2.02550428623587,-1.,-0.753682061113765));
#19612=CARTESIAN_POINT('Ctrl Pts',(-2.01919259406003,-1.,-0.75468233072352));
#19613=CARTESIAN_POINT('Ctrl Pts',(-2.01288584328149,-1.,-0.7556427049581));
#19614=CARTESIAN_POINT('Ctrl Pts',(-2.00658431587682,-1.,-0.756562904646496));
#19615=CARTESIAN_POINT('Ctrl Pts',(-2.00028834739072,-1.,-0.757442676862341));
#19616=CARTESIAN_POINT('Ctrl Pts',(-1.9939983109871,-1.,-0.758281796766377));
#19617=CARTESIAN_POINT('Ctrl Pts',(-1.98771456680806,-1.,-0.759080037802242));
#19618=CARTESIAN_POINT('Ctrl Pts',(-1.98143741418156,-1.,-0.759837147452135));
#19619=CARTESIAN_POINT('Ctrl Pts',(-1.97516705321521,-1.,-0.760552825409855));
#19620=CARTESIAN_POINT('Ctrl Pts',(-1.96890351582545,-1.,-0.761226690483986));
#19621=CARTESIAN_POINT('Ctrl Pts',(-1.96264672744229,-1.,-0.761858300014575));
#19622=CARTESIAN_POINT('Ctrl Pts',(-1.95639665309893,-1.,-0.762447203806263));
#19623=CARTESIAN_POINT('Ctrl Pts',(-1.95015342590025,-1.,-0.762992990878774));
#19624=CARTESIAN_POINT('Ctrl Pts',(-1.94391746617626,-1.,-0.76349533353858));
#19625=CARTESIAN_POINT('Ctrl Pts',(-1.93768964875867,-1.,-0.763954049121393));
#19626=CARTESIAN_POINT('Ctrl Pts',(-1.93147105496367,-1.,-0.764369010673889));
#19627=CARTESIAN_POINT('Ctrl Pts',(-1.92526263537041,-1.,-0.764740025488189));
#19628=CARTESIAN_POINT('Ctrl Pts',(-1.91906491634197,-1.,-0.765066729667095));
#19629=CARTESIAN_POINT('Ctrl Pts',(-1.91287765805174,-1.,-0.765348465884739));
#19630=CARTESIAN_POINT('Ctrl Pts',(-1.90669961402362,-1.,-0.765584196937936));
#19631=CARTESIAN_POINT('Ctrl Pts',(-1.90052930393599,-1.,-0.765772772593395));
#19632=CARTESIAN_POINT('Ctrl Pts',(-1.89436577771389,-1.,-0.765913193856979));
#19633=CARTESIAN_POINT('Ctrl Pts',(-1.88820926433409,-1.,-0.76600483706209));
#19634=CARTESIAN_POINT('Ctrl Pts',(-1.88206215302561,-1.,-0.766047794851868));
#19635=CARTESIAN_POINT('Ctrl Pts',(-1.87592888967886,-1.,-0.766042837036759));
#19636=CARTESIAN_POINT('Ctrl Pts',(-1.86981398314345,-1.,-0.765990708546111));
#19637=CARTESIAN_POINT('Ctrl Pts',(-1.86372027063314,-1.,-0.765891519092557));
#19638=CARTESIAN_POINT('Ctrl Pts',(-1.85764741390391,-1.,-0.765744212909305));
#19639=CARTESIAN_POINT('Ctrl Pts',(-1.85158945130054,-1.,-0.765545710619023));
#19640=CARTESIAN_POINT('Ctrl Pts',(-1.8455369887591,-1.,-0.765291664861971));
#19641=CARTESIAN_POINT('Ctrl Pts',(-1.83948181064823,-1.,-0.764978057881687));
#19642=CARTESIAN_POINT('Ctrl Pts',(-1.8334207722714,-1.,-0.764602549687845));
#19643=CARTESIAN_POINT('Ctrl Pts',(-1.8273599120008,-1.,-0.764165902606055));
#19644=CARTESIAN_POINT('Ctrl Pts',(-1.82131873145297,-1.,-0.763673465462854));
#19645=CARTESIAN_POINT('Ctrl Pts',(-1.81532118405566,-1.,-0.763132003836783));
#19646=CARTESIAN_POINT('Ctrl Pts',(-1.80938551463989,-1.,-0.762546129464036));
#19647=CARTESIAN_POINT('Ctrl Pts',(-1.80351583877334,-1.,-0.761915336443515));
#19648=CARTESIAN_POINT('Ctrl Pts',(-1.79768986997735,-1.,-0.761229695230359));
#19649=CARTESIAN_POINT('Ctrl Pts',(-1.79185815610802,-1.,-0.760469555880425));
#19650=CARTESIAN_POINT('Ctrl Pts',(-1.78596964884526,-1.,-0.759614401109868));
#19651=CARTESIAN_POINT('Ctrl Pts',(-1.77999411220912,-1.,-0.75865062667738));
#19652=CARTESIAN_POINT('Ctrl Pts',(-1.77394167108342,-1.,-0.757578264077238));
#19653=CARTESIAN_POINT('Ctrl Pts',(-1.76789396003141,-1.,-0.756421896028403));
#19654=CARTESIAN_POINT('Ctrl Pts',(-1.7619781724032,-1.,-0.755220979975262));
#19655=CARTESIAN_POINT('Ctrl Pts',(-1.75631083600175,-1.,-0.75400925402848));
#19656=CARTESIAN_POINT('Ctrl Pts',(-1.75095139468809,-1.,-0.752797683531377));
#19657=CARTESIAN_POINT('Ctrl Pts',(-1.74585086852298,-1.,-0.751555614163629));
#19658=CARTESIAN_POINT('Ctrl Pts',(-1.74080458266705,-1.,-0.75019343597954));
#19659=CARTESIAN_POINT('Ctrl Pts',(-1.73550351679848,-1.,-0.748582462954854));
#19660=CARTESIAN_POINT('Ctrl Pts',(-1.72958533647399,-1.,-0.746574710096436));
#19661=CARTESIAN_POINT('Ctrl Pts',(-1.7226822991693,-1.,-0.744021445433764));
#19662=CARTESIAN_POINT('Ctrl Pts',(-1.71447789751927,-1.,-0.740795162032087));
#19663=CARTESIAN_POINT('Ctrl Pts',(-1.70473309006121,-1.,-0.736799665724771));
#19664=CARTESIAN_POINT('Ctrl Pts',(-1.69326921975743,-1.,-0.731963238697195));
#19665=CARTESIAN_POINT('Ctrl Pts',(-1.67996158455503,-1.,-0.726235967997433));
#19666=CARTESIAN_POINT('Ctrl Pts',(-1.6647288055568,-1.,-0.719585433804282));
#19667=CARTESIAN_POINT('Ctrl Pts',(-1.64752408832016,-1.,-0.711993139355394));
#19668=CARTESIAN_POINT('Ctrl Pts',(-1.63216541664676,-1.,-0.705159151988319));
#19669=CARTESIAN_POINT('Ctrl Pts',(-1.61974673472612,-1.,-0.699605146405088));
#19670=CARTESIAN_POINT('Ctrl Pts',(-1.61106790958151,-1.,-0.695712097881194));
#19671=CARTESIAN_POINT('Ctrl Pts',(-1.60662857109684,-1.,-0.693717979106306));
#19672=CARTESIAN_POINT('',(-1.5055822144029,-1.,-0.892032620296855));
#19673=CARTESIAN_POINT('Origin',(0.,-1.,0.));
#19674=CARTESIAN_POINT('',(-1.81978687191668,-1.,-1.23627494547115));
#19675=CARTESIAN_POINT('Ctrl Pts',(-1.5055822144029,-1.,-0.892032620296855));
#19676=CARTESIAN_POINT('Ctrl Pts',(-1.50980486806688,-1.,-0.894452006964543));
#19677=CARTESIAN_POINT('Ctrl Pts',(-1.51805569590094,-1.,-0.899185047483511));
#19678=CARTESIAN_POINT('Ctrl Pts',(-1.52984849887993,-1.,-0.905967409625651));
#19679=CARTESIAN_POINT('Ctrl Pts',(-1.54440491149498,-1.,-0.914375919026456));
#19680=CARTESIAN_POINT('Ctrl Pts',(-1.56065988578893,-1.,-0.923832188944341));
#19681=CARTESIAN_POINT('Ctrl Pts',(-1.57499388382243,-1.,-0.932246680108685));
#19682=CARTESIAN_POINT('Ctrl Pts',(-1.58744937487176,-1.,-0.939646377893399));
#19683=CARTESIAN_POINT('Ctrl Pts',(-1.59810042043673,-1.,-0.946078063315257));
#19684=CARTESIAN_POINT('Ctrl Pts',(-1.60706069896936,-1.,-0.951613284356035));
#19685=CARTESIAN_POINT('Ctrl Pts',(-1.61449324337085,-1.,-0.956354422920671));
#19686=CARTESIAN_POINT('Ctrl Pts',(-1.62061638140221,-1.,-0.960438326101729));
#19687=CARTESIAN_POINT('Ctrl Pts',(-1.62571930670187,-1.,-0.964046107040536));
#19688=CARTESIAN_POINT('Ctrl Pts',(-1.63013849959461,-1.,-0.967387853230345));
#19689=CARTESIAN_POINT('Ctrl Pts',(-1.63420665729798,-1.,-0.970669715997509));
#19690=CARTESIAN_POINT('Ctrl Pts',(-1.63820952658144,-1.,-0.974066058287418));
#19691=CARTESIAN_POINT('Ctrl Pts',(-1.64233990826687,-1.,-0.977689794119416));
#19692=CARTESIAN_POINT('Ctrl Pts',(-1.64665139190656,-1.,-0.981562530939489));
#19693=CARTESIAN_POINT('Ctrl Pts',(-1.65110016612638,-1.,-0.985642622920821));
#19694=CARTESIAN_POINT('Ctrl Pts',(-1.65559044289699,-1.,-0.989855627854165));
#19695=CARTESIAN_POINT('Ctrl Pts',(-1.66001553809947,-1.,-0.994121836661306));
#19696=CARTESIAN_POINT('Ctrl Pts',(-1.66430758030376,-1.,-0.998389654952758));
#19697=CARTESIAN_POINT('Ctrl Pts',(-1.66846059277303,-1.,-1.00265091003727));
#19698=CARTESIAN_POINT('Ctrl Pts',(-1.67250335383293,-1.,-1.00692206696414));
#19699=CARTESIAN_POINT('Ctrl Pts',(-1.67648246776464,-1.,-1.01123236493511));
#19700=CARTESIAN_POINT('Ctrl Pts',(-1.68044289894798,-1.,-1.01561026162773));
#19701=CARTESIAN_POINT('Ctrl Pts',(-1.68440578021706,-1.,-1.02006795074201));
#19702=CARTESIAN_POINT('Ctrl Pts',(-1.68836910178447,-1.,-1.02460180535255));
#19703=CARTESIAN_POINT('Ctrl Pts',(-1.69231840863458,-1.,-1.02919977579147));
#19704=CARTESIAN_POINT('Ctrl Pts',(-1.69623414782771,-1.,-1.03384646003588));
#19705=CARTESIAN_POINT('Ctrl Pts',(-1.70010052930962,-1.,-1.03852922490789));
#19706=CARTESIAN_POINT('Ctrl Pts',(-1.70391338707982,-1.,-1.04324363334554));
#19707=CARTESIAN_POINT('Ctrl Pts',(-1.70767646263649,-1.,-1.04799085404995));
#19708=CARTESIAN_POINT('Ctrl Pts',(-1.71139783543989,-1.,-1.05277517202855));
#19709=CARTESIAN_POINT('Ctrl Pts',(-1.7150865442702,-1.,-1.05760163192479));
#19710=CARTESIAN_POINT('Ctrl Pts',(-1.71874858456904,-1.,-1.06247324680647));
#19711=CARTESIAN_POINT('Ctrl Pts',(-1.72238500928453,-1.,-1.06738966975462));
#19712=CARTESIAN_POINT('Ctrl Pts',(-1.72599406198488,-1.,-1.07234866990252));
#19713=CARTESIAN_POINT('Ctrl Pts',(-1.72957248977424,-1.,-1.0773470373727));
#19714=CARTESIAN_POINT('Ctrl Pts',(-1.73311705663407,-1.,-1.08238162784749));
#19715=CARTESIAN_POINT('Ctrl Pts',(-1.73662628326091,-1.,-1.08745056285427));
#19716=CARTESIAN_POINT('Ctrl Pts',(-1.74010053962247,-1.,-1.09255329056493));
#19717=CARTESIAN_POINT('Ctrl Pts',(-1.74354119236208,-1.,-1.09768999241225));
#19718=CARTESIAN_POINT('Ctrl Pts',(-1.74695004214923,-1.,-1.10286118991143));
#19719=CARTESIAN_POINT('Ctrl Pts',(-1.7503286607592,-1.,-1.10806728183007));
#19720=CARTESIAN_POINT('Ctrl Pts',(-1.7536777209463,-1.,-1.11330807582551));
#19721=CARTESIAN_POINT('Ctrl Pts',(-1.75699720772105,-1.,-1.11858293216763));
#19722=CARTESIAN_POINT('Ctrl Pts',(-1.76028671825096,-1.,-1.12389096855086));
#19723=CARTESIAN_POINT('Ctrl Pts',(-1.7635457196617,-1.,-1.12923123555075));
#19724=CARTESIAN_POINT('Ctrl Pts',(-1.76677384551862,-1.,-1.1346029180462));
#19725=CARTESIAN_POINT('Ctrl Pts',(-1.76997111386769,-1.,-1.14000548336975));
#19726=CARTESIAN_POINT('Ctrl Pts',(-1.77313777896194,-1.,-1.1454385822692));
#19727=CARTESIAN_POINT('Ctrl Pts',(-1.7762742255701,-1.,-1.15090197841515));
#19728=CARTESIAN_POINT('Ctrl Pts',(-1.77938085564275,-1.,-1.15639547194698));
#19729=CARTESIAN_POINT('Ctrl Pts',(-1.78245795881009,-1.,-1.16191881298499));
#19730=CARTESIAN_POINT('Ctrl Pts',(-1.78550566040443,-1.,-1.16747166312303));
#19731=CARTESIAN_POINT('Ctrl Pts',(-1.78852398877616,-1.,-1.17305363177328));
#19732=CARTESIAN_POINT('Ctrl Pts',(-1.79151291552689,-1.,-1.17866429440809));
#19733=CARTESIAN_POINT('Ctrl Pts',(-1.79447240321515,-1.,-1.18430321697432));
#19734=CARTESIAN_POINT('Ctrl Pts',(-1.79740245923478,-1.,-1.18996997934445));
#19735=CARTESIAN_POINT('Ctrl Pts',(-1.80030314369879,-1.,-1.19566418930242));
#19736=CARTESIAN_POINT('Ctrl Pts',(-1.80317454838603,-1.,-1.20138548938974));
#19737=CARTESIAN_POINT('Ctrl Pts',(-1.80601678480707,-1.,-1.20713356605475));
#19738=CARTESIAN_POINT('Ctrl Pts',(-1.80882996917129,-1.,-1.21290815708314));
#19739=CARTESIAN_POINT('Ctrl Pts',(-1.81161420806656,-1.,-1.21870906103557));
#19740=CARTESIAN_POINT('Ctrl Pts',(-1.81436959210434,-1.,-1.2245361330495));
#19741=CARTESIAN_POINT('Ctrl Pts',(-1.8165508718364,-1.,-1.2292186489137));
#19742=CARTESIAN_POINT('Ctrl Pts',(-1.81817389921279,-1.,-1.2327422452705));
#19743=CARTESIAN_POINT('Ctrl Pts',(-1.81925017193666,-1.,-1.23509651170476));
#19744=CARTESIAN_POINT('Ctrl Pts',(-1.81978687191668,-1.,-1.23627494547115));
#19745=CARTESIAN_POINT('',(-1.73811241238545,-1.,-1.34869019493419));
#19746=CARTESIAN_POINT('',(-1.81978687191668,-1.,-1.23627494547115));
#19747=CARTESIAN_POINT('',(-1.31362392696032,-1.,-1.15624053661742));
#19748=CARTESIAN_POINT('Ctrl Pts',(-1.73811241238545,-1.,-1.34869019493419));
#19749=CARTESIAN_POINT('Ctrl Pts',(-1.73682580585691,-1.,-1.34854391898045));
#19750=CARTESIAN_POINT('Ctrl Pts',(-1.73425417885907,-1.,-1.34824783112887));
#19751=CARTESIAN_POINT('Ctrl Pts',(-1.7304014965394,-1.,-1.34779309152035));
#19752=CARTESIAN_POINT('Ctrl Pts',(-1.72527410680674,-1.,-1.34716554819527));
#19753=CARTESIAN_POINT('Ctrl Pts',(-1.7188807715049,-1.,-1.34634568653227));
#19754=CARTESIAN_POINT('Ctrl Pts',(-1.71250340686822,-1.,-1.34549029589416));
#19755=CARTESIAN_POINT('Ctrl Pts',(-1.70614212266738,-1.,-1.34459924533831));
#19756=CARTESIAN_POINT('Ctrl Pts',(-1.69979707754427,-1.,-1.34367237124483));
#19757=CARTESIAN_POINT('Ctrl Pts',(-1.6934684849687,-1.,-1.34270948206319));
#19758=CARTESIAN_POINT('Ctrl Pts',(-1.68715660868764,-1.,-1.341710374848));
#19759=CARTESIAN_POINT('Ctrl Pts',(-1.68086176030362,-1.,-1.34067485185203));
#19760=CARTESIAN_POINT('Ctrl Pts',(-1.67458429426086,-1.,-1.3396027347034));
#19761=CARTESIAN_POINT('Ctrl Pts',(-1.66832460783989,-1.,-1.33849388654388));
#19762=CARTESIAN_POINT('Ctrl Pts',(-1.66208312541983,-1.,-1.33734820885262));
#19763=CARTESIAN_POINT('Ctrl Pts',(-1.65586025952593,-1.,-1.33616559745172));
#19764=CARTESIAN_POINT('Ctrl Pts',(-1.6496563728683,-1.,-1.33494590467993));
#19765=CARTESIAN_POINT('Ctrl Pts',(-1.6434717485603,-1.,-1.33368890676572));
#19766=CARTESIAN_POINT('Ctrl Pts',(-1.63730653475089,-1.,-1.33239425103724));
#19767=CARTESIAN_POINT('Ctrl Pts',(-1.63116079730923,-1.,-1.33106149345645));
#19768=CARTESIAN_POINT('Ctrl Pts',(-1.62503464209797,-1.,-1.3296901950568));
#19769=CARTESIAN_POINT('Ctrl Pts',(-1.61892832270724,-1.,-1.32828000610449));
#19770=CARTESIAN_POINT('Ctrl Pts',(-1.6128423401575,-1.,-1.32683074483356));
#19771=CARTESIAN_POINT('Ctrl Pts',(-1.60677758290954,-1.,-1.32534250785782));
#19772=CARTESIAN_POINT('Ctrl Pts',(-1.60073511858687,-1.,-1.32381550858256));
#19773=CARTESIAN_POINT('Ctrl Pts',(-1.59471591079403,-1.,-1.32224985747682));
#19774=CARTESIAN_POINT('Ctrl Pts',(-1.58872057258245,-1.,-1.32064537110892));
#19775=CARTESIAN_POINT('Ctrl Pts',(-1.58274907898834,-1.,-1.31900135021432));
#19776=CARTESIAN_POINT('Ctrl Pts',(-1.5768005650559,-1.,-1.31731642317187));
#19777=CARTESIAN_POINT('Ctrl Pts',(-1.57087397835723,-1.,-1.31558903860016));
#19778=CARTESIAN_POINT('Ctrl Pts',(-1.56496872402353,-1.,-1.31381795281002));
#19779=CARTESIAN_POINT('Ctrl Pts',(-1.55908521254821,-1.,-1.31200264341696));
#19780=CARTESIAN_POINT('Ctrl Pts',(-1.55322568759481,-1.,-1.31014393684222));
#19781=CARTESIAN_POINT('Ctrl Pts',(-1.54739413957185,-1.,-1.30824393907473));
#19782=CARTESIAN_POINT('Ctrl Pts',(-1.54159462645432,-1.,-1.30630475189556));
#19783=CARTESIAN_POINT('Ctrl Pts',(-1.53582981268977,-1.,-1.30432735639489));
#19784=CARTESIAN_POINT('Ctrl Pts',(-1.53009970283891,-1.,-1.30231064395568));
#19785=CARTESIAN_POINT('Ctrl Pts',(-1.52439957861062,-1.,-1.30024984366328));
#19786=CARTESIAN_POINT('Ctrl Pts',(-1.51872184912724,-1.,-1.29813791800747));
#19787=CARTESIAN_POINT('Ctrl Pts',(-1.51305994241402,-1.,-1.29596850710509));
#19788=CARTESIAN_POINT('Ctrl Pts',(-1.50741159078365,-1.,-1.29373841372842));
#19789=CARTESIAN_POINT('Ctrl Pts',(-1.50178230149776,-1.,-1.29145022885181));
#19790=CARTESIAN_POINT('Ctrl Pts',(-1.49618896881754,-1.,-1.28911506584254));
#19791=CARTESIAN_POINT('Ctrl Pts',(-1.4906522831278,-1.,-1.2867467611644));
#19792=CARTESIAN_POINT('Ctrl Pts',(-1.4851881711891,-1.,-1.28435533880201));
#19793=CARTESIAN_POINT('Ctrl Pts',(-1.47980070347095,-1.,-1.28194158939517));
#19794=CARTESIAN_POINT('Ctrl Pts',(-1.4744717526707,-1.,-1.2794891824849));
#19795=CARTESIAN_POINT('Ctrl Pts',(-1.46916035917133,-1.,-1.27696414831089));
#19796=CARTESIAN_POINT('Ctrl Pts',(-1.46382431332476,-1.,-1.27433119897822));
#19797=CARTESIAN_POINT('Ctrl Pts',(-1.45843906294697,-1.,-1.27156805265289));
#19798=CARTESIAN_POINT('Ctrl Pts',(-1.45301422764247,-1.,-1.2686778680489));
#19799=CARTESIAN_POINT('Ctrl Pts',(-1.44761985001662,-1.,-1.26570925118868));
#19800=CARTESIAN_POINT('Ctrl Pts',(-1.44236470511303,-1.,-1.26273903323859));
#19801=CARTESIAN_POINT('Ctrl Pts',(-1.43734919180848,-1.,-1.25983531012005));
#19802=CARTESIAN_POINT('Ctrl Pts',(-1.43262645609691,-1.,-1.25702687965755));
#19803=CARTESIAN_POINT('Ctrl Pts',(-1.42815938799387,-1.,-1.25426945222639));
#19804=CARTESIAN_POINT('Ctrl Pts',(-1.42378102115575,-1.,-1.2514145557001));
#19805=CARTESIAN_POINT('Ctrl Pts',(-1.41923722596025,-1.,-1.24824430986571));
#19806=CARTESIAN_POINT('Ctrl Pts',(-1.41422913175179,-1.,-1.24450600513056));
#19807=CARTESIAN_POINT('Ctrl Pts',(-1.40845295531283,-1.,-1.23994455029534));
#19808=CARTESIAN_POINT('Ctrl Pts',(-1.40164708206106,-1.,-1.23434087290423));
#19809=CARTESIAN_POINT('Ctrl Pts',(-1.39361389568796,-1.,-1.22752961899387));
#19810=CARTESIAN_POINT('Ctrl Pts',(-1.38420564527715,-1.,-1.21938737280852));
#19811=CARTESIAN_POINT('Ctrl Pts',(-1.37331915607905,-1.,-1.20982812925645));
#19812=CARTESIAN_POINT('Ctrl Pts',(-1.36088705043885,-1.,-1.1987959077932));
#19813=CARTESIAN_POINT('Ctrl Pts',(-1.34687054001093,-1.,-1.18625865667441));
#19814=CARTESIAN_POINT('Ctrl Pts',(-1.33437539347008,-1.,-1.17501305789857));
#19815=CARTESIAN_POINT('Ctrl Pts',(-1.32428080721772,-1.,-1.16589330093588));
#19816=CARTESIAN_POINT('Ctrl Pts',(-1.31722977216397,-1.,-1.15950888730809));
#19817=CARTESIAN_POINT('Ctrl Pts',(-1.31362392696032,-1.,-1.15624053661742));
#19818=CARTESIAN_POINT('',(-1.15624053661742,-1.,-1.31362392696033));
#19819=CARTESIAN_POINT('Origin',(0.,-1.,0.));
#19820=CARTESIAN_POINT('',(-1.34869019493419,-1.,-1.73811241238545));
#19821=CARTESIAN_POINT('Ctrl Pts',(-1.15624053661742,-1.,-1.31362392696033));
#19822=CARTESIAN_POINT('Ctrl Pts',(-1.15950888730433,-1.,-1.3172297721596));
#19823=CARTESIAN_POINT('Ctrl Pts',(-1.16589330092532,-1.,-1.32428080720544));
#19824=CARTESIAN_POINT('Ctrl Pts',(-1.17501305787994,-1.,-1.33437539344842));
#19825=CARTESIAN_POINT('Ctrl Pts',(-1.18625865664915,-1.,-1.34687053998157));
#19826=CARTESIAN_POINT('Ctrl Pts',(-1.1987959077656,-1.,-1.36088705040677));
#19827=CARTESIAN_POINT('Ctrl Pts',(-1.20982812923113,-1.,-1.37331915604962));
#19828=CARTESIAN_POINT('Ctrl Pts',(-1.21938737278853,-1.,-1.38420564525391));
#19829=CARTESIAN_POINT('Ctrl Pts',(-1.22752961898063,-1.,-1.39361389567257));
#19830=CARTESIAN_POINT('Ctrl Pts',(-1.23434087289768,-1.,-1.40164708205345));
#19831=CARTESIAN_POINT('Ctrl Pts',(-1.23994455029421,-1.,-1.40845295531151));
#19832=CARTESIAN_POINT('Ctrl Pts',(-1.24450600513278,-1.,-1.41422913175437));
#19833=CARTESIAN_POINT('Ctrl Pts',(-1.24824430986911,-1.,-1.41923722596421));
#19834=CARTESIAN_POINT('Ctrl Pts',(-1.25141455570299,-1.,-1.42378102115911));
#19835=CARTESIAN_POINT('Ctrl Pts',(-1.25426945222783,-1.,-1.42815938799555));
#19836=CARTESIAN_POINT('Ctrl Pts',(-1.25702687965744,-1.,-1.43262645609679));
#19837=CARTESIAN_POINT('Ctrl Pts',(-1.25983531011894,-1.,-1.43734919180719));
#19838=CARTESIAN_POINT('Ctrl Pts',(-1.26273903323723,-1.,-1.44236470511145));
#19839=CARTESIAN_POINT('Ctrl Pts',(-1.26570925118767,-1.,-1.44761985001544));
#19840=CARTESIAN_POINT('Ctrl Pts',(-1.26867786804854,-1.,-1.45301422764205));
#19841=CARTESIAN_POINT('Ctrl Pts',(-1.27156805265312,-1.,-1.45843906294725));
#19842=CARTESIAN_POINT('Ctrl Pts',(-1.27433119897877,-1.,-1.4638243133254));
#19843=CARTESIAN_POINT('Ctrl Pts',(-1.27696414831144,-1.,-1.46916035917197));
#19844=CARTESIAN_POINT('Ctrl Pts',(-1.27948918248524,-1.,-1.4744717526711));
#19845=CARTESIAN_POINT('Ctrl Pts',(-1.28194158939522,-1.,-1.47980070347102));
#19846=CARTESIAN_POINT('Ctrl Pts',(-1.28435533880184,-1.,-1.48518817118891));
#19847=CARTESIAN_POINT('Ctrl Pts',(-1.28674676116415,-1.,-1.4906522831275));
#19848=CARTESIAN_POINT('Ctrl Pts',(-1.28911506584232,-1.,-1.49618896881729));
#19849=CARTESIAN_POINT('Ctrl Pts',(-1.29145022885171,-1.,-1.50178230149764));
#19850=CARTESIAN_POINT('Ctrl Pts',(-1.29373841372843,-1.,-1.50741159078367));
#19851=CARTESIAN_POINT('Ctrl Pts',(-1.29596850710518,-1.,-1.51305994241412));
#19852=CARTESIAN_POINT('Ctrl Pts',(-1.29813791800757,-1.,-1.51872184912735));
#19853=CARTESIAN_POINT('Ctrl Pts',(-1.30024984366334,-1.,-1.5243995786107));
#19854=CARTESIAN_POINT('Ctrl Pts',(-1.3023106439557,-1.,-1.53009970283893));
#19855=CARTESIAN_POINT('Ctrl Pts',(-1.30432735639487,-1.,-1.53582981268976));
#19856=CARTESIAN_POINT('Ctrl Pts',(-1.30630475189553,-1.,-1.54159462645428));
#19857=CARTESIAN_POINT('Ctrl Pts',(-1.30824393907471,-1.,-1.54739413957183));
#19858=CARTESIAN_POINT('Ctrl Pts',(-1.31014393684221,-1.,-1.55322568759481));
#19859=CARTESIAN_POINT('Ctrl Pts',(-1.31200264341696,-1.,-1.55908521254822));
#19860=CARTESIAN_POINT('Ctrl Pts',(-1.31381795281002,-1.,-1.56496872402352));
#19861=CARTESIAN_POINT('Ctrl Pts',(-1.31558903860015,-1.,-1.57087397835721));
#19862=CARTESIAN_POINT('Ctrl Pts',(-1.31731642317183,-1.,-1.57680056505585));
#19863=CARTESIAN_POINT('Ctrl Pts',(-1.31900135021428,-1.,-1.58274907898829));
#19864=CARTESIAN_POINT('Ctrl Pts',(-1.32064537110891,-1.,-1.58872057258244));
#19865=CARTESIAN_POINT('Ctrl Pts',(-1.32224985747686,-1.,-1.59471591079408));
#19866=CARTESIAN_POINT('Ctrl Pts',(-1.32381550858266,-1.,-1.600735118587));
#19867=CARTESIAN_POINT('Ctrl Pts',(-1.32534250785794,-1.,-1.6067775829097));
#19868=CARTESIAN_POINT('Ctrl Pts',(-1.32683074483365,-1.,-1.61284234015762));
#19869=CARTESIAN_POINT('Ctrl Pts',(-1.32828000610448,-1.,-1.61892832270723));
#19870=CARTESIAN_POINT('Ctrl Pts',(-1.32969019505665,-1.,-1.62503464209777));
#19871=CARTESIAN_POINT('Ctrl Pts',(-1.33106149345618,-1.,-1.63116079730887));
#19872=CARTESIAN_POINT('Ctrl Pts',(-1.33239425103694,-1.,-1.6373065347505));
#19873=CARTESIAN_POINT('Ctrl Pts',(-1.33368890676554,-1.,-1.64347174856007));
#19874=CARTESIAN_POINT('Ctrl Pts',(-1.33494590468003,-1.,-1.64965637286843));
#19875=CARTESIAN_POINT('Ctrl Pts',(-1.33616559745217,-1.,-1.65586025952651));
#19876=CARTESIAN_POINT('Ctrl Pts',(-1.33734820885331,-1.,-1.66208312542073));
#19877=CARTESIAN_POINT('Ctrl Pts',(-1.33849388654458,-1.,-1.66832460784078));
#19878=CARTESIAN_POINT('Ctrl Pts',(-1.33960273470372,-1.,-1.67458429426126));
#19879=CARTESIAN_POINT('Ctrl Pts',(-1.3406748518516,-1.,-1.68086176030308));
#19880=CARTESIAN_POINT('Ctrl Pts',(-1.34171037484673,-1.,-1.68715660868602));
#19881=CARTESIAN_POINT('Ctrl Pts',(-1.34270948206139,-1.,-1.6934684849664));
#19882=CARTESIAN_POINT('Ctrl Pts',(-1.34367237124322,-1.,-1.69979707754221));
#19883=CARTESIAN_POINT('Ctrl Pts',(-1.34459924533783,-1.,-1.70614212266676));
#19884=CARTESIAN_POINT('Ctrl Pts',(-1.34549029589563,-1.,-1.71250340687011));
#19885=CARTESIAN_POINT('Ctrl Pts',(-1.34634568653586,-1.,-1.7188807715095));
#19886=CARTESIAN_POINT('Ctrl Pts',(-1.34716554820013,-1.,-1.72527410681298));
#19887=CARTESIAN_POINT('Ctrl Pts',(-1.3477930915247,-1.,-1.73040149654497));
#19888=CARTESIAN_POINT('Ctrl Pts',(-1.34824783113158,-1.,-1.73425417886255));
#19889=CARTESIAN_POINT('Ctrl Pts',(-1.34854391898145,-1.,-1.73682580585819));
#19890=CARTESIAN_POINT('Ctrl Pts',(-1.34869019493419,-1.,-1.73811241238545));
#19891=CARTESIAN_POINT('',(-1.23627494547115,-1.,-1.81978687191668));
#19892=CARTESIAN_POINT('',(-1.34869019493419,-1.,-1.73811241238545));
#19893=CARTESIAN_POINT('',(-0.892032620296855,-1.,-1.5055822144029));
#19894=CARTESIAN_POINT('Ctrl Pts',(-1.23627494547115,-1.,-1.81978687191668));
#19895=CARTESIAN_POINT('Ctrl Pts',(-1.23509651170384,-1.,-1.81925017193531));
#19896=CARTESIAN_POINT('Ctrl Pts',(-1.23274224526804,-1.,-1.81817389920914));
#19897=CARTESIAN_POINT('Ctrl Pts',(-1.22921864890975,-1.,-1.81655087183054));
#19898=CARTESIAN_POINT('Ctrl Pts',(-1.22453613304507,-1.,-1.81436959209778));
#19899=CARTESIAN_POINT('Ctrl Pts',(-1.2187090610323,-1.,-1.81161420806172));
#19900=CARTESIAN_POINT('Ctrl Pts',(-1.2129081570818,-1.,-1.80882996916931));
#19901=CARTESIAN_POINT('Ctrl Pts',(-1.20713356605519,-1.,-1.80601678480772));
#19902=CARTESIAN_POINT('Ctrl Pts',(-1.2013854893912,-1.,-1.8031745483882));
#19903=CARTESIAN_POINT('Ctrl Pts',(-1.19566418930405,-1.,-1.80030314370121));
#19904=CARTESIAN_POINT('Ctrl Pts',(-1.1899699793456,-1.,-1.79740245923649));
#19905=CARTESIAN_POINT('Ctrl Pts',(-1.18430321697471,-1.,-1.79447240321572));
#19906=CARTESIAN_POINT('Ctrl Pts',(-1.17866429440781,-1.,-1.79151291552646));
#19907=CARTESIAN_POINT('Ctrl Pts',(-1.17305363177265,-1.,-1.78852398877523));
#19908=CARTESIAN_POINT('Ctrl Pts',(-1.16747166312239,-1.,-1.78550566040349));
#19909=CARTESIAN_POINT('Ctrl Pts',(-1.16191881298458,-1.,-1.78245795880949));
#19910=CARTESIAN_POINT('Ctrl Pts',(-1.15639547194689,-1.,-1.77938085564261));
#19911=CARTESIAN_POINT('Ctrl Pts',(-1.15090197841531,-1.,-1.77627422557034));
#19912=CARTESIAN_POINT('Ctrl Pts',(-1.14543858226948,-1.,-1.77313777896234));
#19913=CARTESIAN_POINT('Ctrl Pts',(-1.14000548337,-1.,-1.76997111386806));
#19914=CARTESIAN_POINT('Ctrl Pts',(-1.13460291804635,-1.,-1.76677384551883));
#19915=CARTESIAN_POINT('Ctrl Pts',(-1.12923123555076,-1.,-1.76354571966171));
#19916=CARTESIAN_POINT('Ctrl Pts',(-1.12389096855078,-1.,-1.76028671825084));
#19917=CARTESIAN_POINT('Ctrl Pts',(-1.11858293216752,-1.,-1.75699720772089));
#19918=CARTESIAN_POINT('Ctrl Pts',(-1.11330807582542,-1.,-1.75367772094617));
#19919=CARTESIAN_POINT('Ctrl Pts',(-1.10806728183003,-1.,-1.75032866075914));
#19920=CARTESIAN_POINT('Ctrl Pts',(-1.10286118991144,-1.,-1.74695004214924));
#19921=CARTESIAN_POINT('Ctrl Pts',(-1.09768999241229,-1.,-1.74354119236212));
#19922=CARTESIAN_POINT('Ctrl Pts',(-1.09255329056496,-1.,-1.74010053962252));
#19923=CARTESIAN_POINT('Ctrl Pts',(-1.08745056285429,-1.,-1.73662628326093));
#19924=CARTESIAN_POINT('Ctrl Pts',(-1.08238162784749,-1.,-1.73311705663407));
#19925=CARTESIAN_POINT('Ctrl Pts',(-1.0773470373727,-1.,-1.72957248977424));
#19926=CARTESIAN_POINT('Ctrl Pts',(-1.07234866990252,-1.,-1.72599406198489));
#19927=CARTESIAN_POINT('Ctrl Pts',(-1.06738966975463,-1.,-1.72238500928456));
#19928=CARTESIAN_POINT('Ctrl Pts',(-1.0624732468065,-1.,-1.71874858456908));
#19929=CARTESIAN_POINT('Ctrl Pts',(-1.05760163192481,-1.,-1.71508654427022));
#19930=CARTESIAN_POINT('Ctrl Pts',(-1.05277517202854,-1.,-1.71139783543986));
#19931=CARTESIAN_POINT('Ctrl Pts',(-1.0479908540499,-1.,-1.70767646263641));
#19932=CARTESIAN_POINT('Ctrl Pts',(-1.04324363334546,-1.,-1.70391338707969));
#19933=CARTESIAN_POINT('Ctrl Pts',(-1.03852922490782,-1.,-1.70010052930951));
#19934=CARTESIAN_POINT('Ctrl Pts',(-1.03384646003587,-1.,-1.69623414782769));
#19935=CARTESIAN_POINT('Ctrl Pts',(-1.02919977579155,-1.,-1.69231840863471));
#19936=CARTESIAN_POINT('Ctrl Pts',(-1.02460180535272,-1.,-1.68836910178475));
#19937=CARTESIAN_POINT('Ctrl Pts',(-1.02006795074222,-1.,-1.68440578021739));
#19938=CARTESIAN_POINT('Ctrl Pts',(-1.01561026162787,-1.,-1.6804428989482));
#19939=CARTESIAN_POINT('Ctrl Pts',(-1.01123236493507,-1.,-1.67648246776457));
#19940=CARTESIAN_POINT('Ctrl Pts',(-1.00692206696387,-1.,-1.67250335383248));
#19941=CARTESIAN_POINT('Ctrl Pts',(-1.00265091003682,-1.,-1.66846059277231));
#19942=CARTESIAN_POINT('Ctrl Pts',(-0.998389654952317,-1.,-1.66430758030304));
#19943=CARTESIAN_POINT('Ctrl Pts',(-0.994121836661116,-1.,-1.66001553809916));
#19944=CARTESIAN_POINT('Ctrl Pts',(-0.98985562785445,-1.,-1.65559044289746));
#19945=CARTESIAN_POINT('Ctrl Pts',(-0.985642622921626,-1.,-1.6511001661277));
#19946=CARTESIAN_POINT('Ctrl Pts',(-0.981562530940574,-1.,-1.64665139190834));
#19947=CARTESIAN_POINT('Ctrl Pts',(-0.977689794120297,-1.,-1.64233990826831));
#19948=CARTESIAN_POINT('Ctrl Pts',(-0.974066058287501,-1.,-1.63820952658157));
#19949=CARTESIAN_POINT('Ctrl Pts',(-0.970669715996356,-1.,-1.63420665729609));
#19950=CARTESIAN_POINT('Ctrl Pts',(-0.967387853228041,-1.,-1.63013849959083));
#19951=CARTESIAN_POINT('Ctrl Pts',(-0.964046107037821,-1.,-1.6257193066974));
#19952=CARTESIAN_POINT('Ctrl Pts',(-0.960438326099958,-1.,-1.62061638139929));
#19953=CARTESIAN_POINT('Ctrl Pts',(-0.956354422921573,-1.,-1.61449324337233));
#19954=CARTESIAN_POINT('Ctrl Pts',(-0.951613284361248,-1.,-1.60706069897794));
#19955=CARTESIAN_POINT('Ctrl Pts',(-0.946078063325796,-1.,-1.59810042045408));
#19956=CARTESIAN_POINT('Ctrl Pts',(-0.939646377909319,-1.,-1.58744937489796));
#19957=CARTESIAN_POINT('Ctrl Pts',(-0.932246680128849,-1.,-1.57499388385561));
#19958=CARTESIAN_POINT('Ctrl Pts',(-0.923832188966322,-1.,-1.56065988582509));
#19959=CARTESIAN_POINT('Ctrl Pts',(-0.91437591904658,-1.,-1.54440491152808));
#19960=CARTESIAN_POINT('Ctrl Pts',(-0.905967409640499,-1.,-1.52984849890434));
#19961=CARTESIAN_POINT('Ctrl Pts',(-0.89918504749193,-1.,-1.51805569591479));
#19962=CARTESIAN_POINT('Ctrl Pts',(-0.894452006967538,-1.,-1.50980486807181));
#19963=CARTESIAN_POINT('Ctrl Pts',(-0.892032620296855,-1.,-1.5055822144029));
#19964=CARTESIAN_POINT('',(-0.693717979106305,-1.,-1.60662857109684));
#19965=CARTESIAN_POINT('Origin',(0.,-1.,0.));
#19966=CARTESIAN_POINT('',(-0.745574324794401,-1.,-2.0698113262342));
#19967=CARTESIAN_POINT('Ctrl Pts',(-0.693717979106305,-1.,-1.60662857109684));
#19968=CARTESIAN_POINT('Ctrl Pts',(-0.69571209787897,-1.,-1.61106790957619));
#19969=CARTESIAN_POINT('Ctrl Pts',(-0.699605146398837,-1.,-1.61974673471117));
#19970=CARTESIAN_POINT('Ctrl Pts',(-0.705159151977294,-1.,-1.6321654166204));
#19971=CARTESIAN_POINT('Ctrl Pts',(-0.711993139340447,-1.,-1.64752408828442));
#19972=CARTESIAN_POINT('Ctrl Pts',(-0.71958543378795,-1.,-1.66472880551777));
#19973=CARTESIAN_POINT('Ctrl Pts',(-0.726235967982445,-1.,-1.67996158451922));
#19974=CARTESIAN_POINT('Ctrl Pts',(-0.731963238685357,-1.,-1.69326921972915));
#19975=CARTESIAN_POINT('Ctrl Pts',(-0.736799665716932,-1.,-1.70473309004249));
#19976=CARTESIAN_POINT('Ctrl Pts',(-0.74079516202821,-1.,-1.71447789751001));
#19977=CARTESIAN_POINT('Ctrl Pts',(-0.744021445433093,-1.,-1.72268229916769));
#19978=CARTESIAN_POINT('Ctrl Pts',(-0.746574710097752,-1.,-1.72958533647714));
#19979=CARTESIAN_POINT('Ctrl Pts',(-0.74858246295687,-1.,-1.7355035168033));
#19980=CARTESIAN_POINT('Ctrl Pts',(-0.750193435981249,-1.,-1.74080458267114));
#19981=CARTESIAN_POINT('Ctrl Pts',(-0.751555614164482,-1.,-1.74585086852502));
#19982=CARTESIAN_POINT('Ctrl Pts',(-0.752797683531314,-1.,-1.75095139468794));
#19983=CARTESIAN_POINT('Ctrl Pts',(-0.754009254027829,-1.,-1.75631083600019));
#19984=CARTESIAN_POINT('Ctrl Pts',(-0.755220979974461,-1.,-1.76197817240128));
#19985=CARTESIAN_POINT('Ctrl Pts',(-0.75642189602781,-1.,-1.76789396002998));
#19986=CARTESIAN_POINT('Ctrl Pts',(-0.757578264077029,-1.,-1.77394167108292));
#19987=CARTESIAN_POINT('Ctrl Pts',(-0.758650626677518,-1.,-1.77999411220945));
#19988=CARTESIAN_POINT('Ctrl Pts',(-0.759614401110189,-1.,-1.78596964884604));
#19989=CARTESIAN_POINT('Ctrl Pts',(-0.760469555880749,-1.,-1.7918581561088));
#19990=CARTESIAN_POINT('Ctrl Pts',(-0.761229695230558,-1.,-1.79768986997783));
#19991=CARTESIAN_POINT('Ctrl Pts',(-0.761915336443547,-1.,-1.80351583877342));
#19992=CARTESIAN_POINT('Ctrl Pts',(-0.762546129463938,-1.,-1.80938551463965));
#19993=CARTESIAN_POINT('Ctrl Pts',(-0.763132003836634,-1.,-1.8153211840553));
#19994=CARTESIAN_POINT('Ctrl Pts',(-0.763673465462726,-1.,-1.82131873145266));
#19995=CARTESIAN_POINT('Ctrl Pts',(-0.764165902605995,-1.,-1.82735991200065));
#19996=CARTESIAN_POINT('Ctrl Pts',(-0.764602549687853,-1.,-1.83342077227142));
#19997=CARTESIAN_POINT('Ctrl Pts',(-0.764978057881737,-1.,-1.83948181064835));
#19998=CARTESIAN_POINT('Ctrl Pts',(-0.765291664862029,-1.,-1.84553698875924));
#19999=CARTESIAN_POINT('Ctrl Pts',(-0.765545710619062,-1.,-1.85158945130063));
#20000=CARTESIAN_POINT('Ctrl Pts',(-0.765744212909318,-1.,-1.85764741390394));
#20001=CARTESIAN_POINT('Ctrl Pts',(-0.765891519092547,-1.,-1.86372027063312));
#20002=CARTESIAN_POINT('Ctrl Pts',(-0.765990708546091,-1.,-1.86981398314341));
#20003=CARTESIAN_POINT('Ctrl Pts',(-0.766042837036744,-1.,-1.87592888967883));
#20004=CARTESIAN_POINT('Ctrl Pts',(-0.766047794851865,-1.,-1.88206215302561));
#20005=CARTESIAN_POINT('Ctrl Pts',(-0.766004837062091,-1.,-1.88820926433409));
#20006=CARTESIAN_POINT('Ctrl Pts',(-0.765913193856978,-1.,-1.89436577771388));
#20007=CARTESIAN_POINT('Ctrl Pts',(-0.765772772593386,-1.,-1.90052930393596));
#20008=CARTESIAN_POINT('Ctrl Pts',(-0.765584196937919,-1.,-1.90669961402356));
#20009=CARTESIAN_POINT('Ctrl Pts',(-0.765348465884722,-1.,-1.91287765805169));
#20010=CARTESIAN_POINT('Ctrl Pts',(-0.765066729667088,-1.,-1.91906491634196));
#20011=CARTESIAN_POINT('Ctrl Pts',(-0.764740025488211,-1.,-1.92526263537048));
#20012=CARTESIAN_POINT('Ctrl Pts',(-0.764369010673941,-1.,-1.93147105496382));
#20013=CARTESIAN_POINT('Ctrl Pts',(-0.763954049121458,-1.,-1.93768964875886));
#20014=CARTESIAN_POINT('Ctrl Pts',(-0.763495333538629,-1.,-1.9439174661764));
#20015=CARTESIAN_POINT('Ctrl Pts',(-0.762992990878769,-1.,-1.95015342590024));
#20016=CARTESIAN_POINT('Ctrl Pts',(-0.762447203806179,-1.,-1.95639665309869));
#20017=CARTESIAN_POINT('Ctrl Pts',(-0.761858300014423,-1.,-1.96264672744186));
#20018=CARTESIAN_POINT('Ctrl Pts',(-0.76122669048382,-1.,-1.96890351582499));
#20019=CARTESIAN_POINT('Ctrl Pts',(-0.760552825409757,-1.,-1.97516705321494));
#20020=CARTESIAN_POINT('Ctrl Pts',(-0.75983714745219,-1.,-1.98143741418172));
#20021=CARTESIAN_POINT('Ctrl Pts',(-0.759080037802488,-1.,-1.98771456680874));
#20022=CARTESIAN_POINT('Ctrl Pts',(-0.758281796766761,-1.,-1.99399831098817));
#20023=CARTESIAN_POINT('Ctrl Pts',(-0.757442676862724,-1.,-2.00028834739178));
#20024=CARTESIAN_POINT('Ctrl Pts',(-0.75656290464667,-1.,-2.0065843158773));
#20025=CARTESIAN_POINT('Ctrl Pts',(-0.755642704957865,-1.,-2.01288584328084));
#20026=CARTESIAN_POINT('Ctrl Pts',(-0.754682330722816,-1.,-2.01919259405809));
#20027=CARTESIAN_POINT('Ctrl Pts',(-0.753682061112768,-1.,-2.02550428623313));
#20028=CARTESIAN_POINT('Ctrl Pts',(-0.752642180487211,-1.,-2.03182068456221));
#20029=CARTESIAN_POINT('Ctrl Pts',(-0.751562963361115,-1.,-2.03814160092099));
#20030=CARTESIAN_POINT('Ctrl Pts',(-0.750444657875576,-1.,-2.04446689147979));
#20031=CARTESIAN_POINT('Ctrl Pts',(-0.749287468665046,-1.,-2.05079645592154));
#20032=CARTESIAN_POINT('Ctrl Pts',(-0.748091554183802,-1.,-2.05713023031006));
#20033=CARTESIAN_POINT('Ctrl Pts',(-0.747103932787919,-1.,-2.06220058927826));
#20034=CARTESIAN_POINT('Ctrl Pts',(-0.7463458715442,-1.,-2.06600523016815));
#20035=CARTESIAN_POINT('Ctrl Pts',(-0.745832791378367,-1.,-2.06854248895728));
#20036=CARTESIAN_POINT('Ctrl Pts',(-0.745574324794401,-1.,-2.0698113262342));
#20037=CARTESIAN_POINT('',(-0.61342227326009,-1.,-2.11275013067528));
#20038=CARTESIAN_POINT('',(-0.745574324794401,-1.,-2.0698113262342));
#20039=CARTESIAN_POINT('',(-0.383122945602004,-1.,-1.7075470150345));
#20040=CARTESIAN_POINT('Ctrl Pts',(-0.61342227326009,-1.,-2.11275013067528));
#20041=CARTESIAN_POINT('Ctrl Pts',(-0.6124673655618,-1.,-2.11187554259986));
#20042=CARTESIAN_POINT('Ctrl Pts',(-0.610560911689899,-1.,-2.11012443807238));
#20043=CARTESIAN_POINT('Ctrl Pts',(-0.607711315454876,-1.,-2.1074919961518));
#20044=CARTESIAN_POINT('Ctrl Pts',(-0.60393203073603,-1.,-2.10397049886949));
#20045=CARTESIAN_POINT('Ctrl Pts',(-0.599241616420533,-1.,-2.0995493086477));
#20046=CARTESIAN_POINT('Ctrl Pts',(-0.594585006052162,-1.,-2.0951087622027));
#20047=CARTESIAN_POINT('Ctrl Pts',(-0.589962365403406,-1.,-2.09064881812129));
#20048=CARTESIAN_POINT('Ctrl Pts',(-0.585373918991617,-1.,-2.08616943727951));
#20049=CARTESIAN_POINT('Ctrl Pts',(-0.580819952108063,-1.,-2.08167059018418));
#20050=CARTESIAN_POINT('Ctrl Pts',(-0.576300797416844,-1.,-2.07715226767559));
#20051=CARTESIAN_POINT('Ctrl Pts',(-0.571816823242603,-1.,-2.07261449292824));
#20052=CARTESIAN_POINT('Ctrl Pts',(-0.567368421181087,-1.,-2.06805732997334));
#20053=CARTESIAN_POINT('Ctrl Pts',(-0.562955993082261,-1.,-2.06348090160589));
#20054=CARTESIAN_POINT('Ctrl Pts',(-0.558579940185151,-1.,-2.05888537756462));
#20055=CARTESIAN_POINT('Ctrl Pts',(-0.554240657463906,-1.,-2.05427091604413));
#20056=CARTESIAN_POINT('Ctrl Pts',(-0.549938525150295,-1.,-2.04963761077958));
#20057=CARTESIAN_POINT('Ctrl Pts',(-0.54567390381743,-1.,-2.04498544714588));
#20058=CARTESIAN_POINT('Ctrl Pts',(-0.541447120615659,-1.,-2.04031422690527));
#20059=CARTESIAN_POINT('Ctrl Pts',(-0.537258489833262,-1.,-2.03562362954037));
#20060=CARTESIAN_POINT('Ctrl Pts',(-0.533108355132977,-1.,-2.03091336214426));
#20061=CARTESIAN_POINT('Ctrl Pts',(-0.528997127241914,-1.,-2.0261832908329));
#20062=CARTESIAN_POINT('Ctrl Pts',(-0.524925318333476,-1.,-2.02143356304698));
#20063=CARTESIAN_POINT('Ctrl Pts',(-0.52089359039937,-1.,-2.01666477917286));
#20064=CARTESIAN_POINT('Ctrl Pts',(-0.516902681728687,-1.,-2.01187773939242));
#20065=CARTESIAN_POINT('Ctrl Pts',(-0.512953306961792,-1.,-2.00707309946949));
#20066=CARTESIAN_POINT('Ctrl Pts',(-0.509046069886157,-1.,-2.00225107134734));
#20067=CARTESIAN_POINT('Ctrl Pts',(-0.505181361323026,-1.,-1.99741107463572));
#20068=CARTESIAN_POINT('Ctrl Pts',(-0.501359287727146,-1.,-1.99255149126155));
#20069=CARTESIAN_POINT('Ctrl Pts',(-0.497579909545574,-1.,-1.98767044752932));
#20070=CARTESIAN_POINT('Ctrl Pts',(-0.493843476541495,-1.,-1.98276658761821));
#20071=CARTESIAN_POINT('Ctrl Pts',(-0.490150627860952,-1.,-1.97783973019229));
#20072=CARTESIAN_POINT('Ctrl Pts',(-0.486502692907659,-1.,-1.97289186263272));
#20073=CARTESIAN_POINT('Ctrl Pts',(-0.482901662120691,-1.,-1.96792703422362));
#20074=CARTESIAN_POINT('Ctrl Pts',(-0.479349583074855,-1.,-1.96294933055943));
#20075=CARTESIAN_POINT('Ctrl Pts',(-0.475848034683176,-1.,-1.95796111148177));
#20076=CARTESIAN_POINT('Ctrl Pts',(-0.472397672264072,-1.,-1.95296148278133));
#20077=CARTESIAN_POINT('Ctrl Pts',(-0.468997482913135,-1.,-1.94794381136514));
#20078=CARTESIAN_POINT('Ctrl Pts',(-0.46564546202603,-1.,-1.9428979419619));
#20079=CARTESIAN_POINT('Ctrl Pts',(-0.462340031009056,-1.,-1.93781486640821));
#20080=CARTESIAN_POINT('Ctrl Pts',(-0.459081234547926,-1.,-1.93269066517934));
#20081=CARTESIAN_POINT('Ctrl Pts',(-0.455872005174371,-1.,-1.92753067150476));
#20082=CARTESIAN_POINT('Ctrl Pts',(-0.452719478359432,-1.,-1.92235380648502));
#20083=CARTESIAN_POINT('Ctrl Pts',(-0.449632260106662,-1.,-1.91718342555755));
#20084=CARTESIAN_POINT('Ctrl Pts',(-0.446617343485711,-1.,-1.9120369998112));
#20085=CARTESIAN_POINT('Ctrl Pts',(-0.443677556849151,-1.,-1.90691756144898));
#20086=CARTESIAN_POINT('Ctrl Pts',(-0.440807833704038,-1.,-1.90180124389086));
#20087=CARTESIAN_POINT('Ctrl Pts',(-0.437995003948244,-1.,-1.89663648956466));
#20088=CARTESIAN_POINT('Ctrl Pts',(-0.435225660963383,-1.,-1.89136993975504));
#20089=CARTESIAN_POINT('Ctrl Pts',(-0.432493038548748,-1.,-1.88596913666793));
#20090=CARTESIAN_POINT('Ctrl Pts',(-0.429803062482344,-1.,-1.88044229001832));
#20091=CARTESIAN_POINT('Ctrl Pts',(-0.427183828519102,-1.,-1.87486989291484));
#20092=CARTESIAN_POINT('Ctrl Pts',(-0.424678177291359,-1.,-1.86937803944323));
#20093=CARTESIAN_POINT('Ctrl Pts',(-0.422327307418275,-1.,-1.86408083334028));
#20094=CARTESIAN_POINT('Ctrl Pts',(-0.420157287975619,-1.,-1.85903281096686));
#20095=CARTESIAN_POINT('Ctrl Pts',(-0.418164129143534,-1.,-1.85417632856234));
#20096=CARTESIAN_POINT('Ctrl Pts',(-0.416300022038864,-1.,-1.84929312929882));
#20097=CARTESIAN_POINT('Ctrl Pts',(-0.41448743825434,-1.,-1.8440575707371));
#20098=CARTESIAN_POINT('Ctrl Pts',(-0.412633125322162,-1.,-1.83808953475839));
#20099=CARTESIAN_POINT('Ctrl Pts',(-0.410641256301675,-1.,-1.83100408895216));
#20100=CARTESIAN_POINT('Ctrl Pts',(-0.408428948108533,-1.,-1.8224702267854));
#20101=CARTESIAN_POINT('Ctrl Pts',(-0.405933518411838,-1.,-1.81223801813988));
#20102=CARTESIAN_POINT('Ctrl Pts',(-0.403107976170441,-1.,-1.80012077176221));
#20103=CARTESIAN_POINT('Ctrl Pts',(-0.39991940378308,-1.,-1.78598826347533));
#20104=CARTESIAN_POINT('Ctrl Pts',(-0.39634619612042,-1.,-1.7697556004756));
#20105=CARTESIAN_POINT('Ctrl Pts',(-0.392375812294307,-1.,-1.75137405313962));
#20106=CARTESIAN_POINT('Ctrl Pts',(-0.388877023509191,-1.,-1.7349317097561));
#20107=CARTESIAN_POINT('Ctrl Pts',(-0.38607079032701,-1.,-1.72162022246158));
#20108=CARTESIAN_POINT('Ctrl Pts',(-0.384119047315542,-1.,-1.71231062891958));
#20109=CARTESIAN_POINT('Ctrl Pts',(-0.383122945602004,-1.,-1.7075470150345));
#20110=CARTESIAN_POINT('',(-0.163289472382896,-1.,-1.74236521665491));
#20111=CARTESIAN_POINT('Origin',(0.,-1.,0.));
#20112=CARTESIAN_POINT('',(-0.0694764450219581,-1.,-2.19890268624765));
#20113=CARTESIAN_POINT('Ctrl Pts',(-0.163289472382896,-1.,-1.74236521665491));
#20114=CARTESIAN_POINT('Ctrl Pts',(-0.163814161002002,-1.,-1.7472034950333));
#20115=CARTESIAN_POINT('Ctrl Pts',(-0.164834765707158,-1.,-1.75666056638427));
#20116=CARTESIAN_POINT('Ctrl Pts',(-0.1662793551464,-1.,-1.77018771684844));
#20117=CARTESIAN_POINT('Ctrl Pts',(-0.168032772805197,-1.,-1.7869064998507));
#20118=CARTESIAN_POINT('Ctrl Pts',(-0.169936923904608,-1.,-1.80561530629706));
#20119=CARTESIAN_POINT('Ctrl Pts',(-0.171554770204119,-1.,-1.82215766811545));
#20120=CARTESIAN_POINT('Ctrl Pts',(-0.1728894428919,-1.,-1.83658380527692));
#20121=CARTESIAN_POINT('Ctrl Pts',(-0.173946627587731,-1.,-1.8489811319852));
#20122=CARTESIAN_POINT('Ctrl Pts',(-0.17473525927603,-1.,-1.85948367088837));
#20123=CARTESIAN_POINT('Ctrl Pts',(-0.175268337590758,-1.,-1.86828349694799));
#20124=CARTESIAN_POINT('Ctrl Pts',(-0.175563480746485,-1.,-1.87563767773588));
#20125=CARTESIAN_POINT('Ctrl Pts',(-0.175644148889699,-1.,-1.88188663145367));
#20126=CARTESIAN_POINT('Ctrl Pts',(-0.175538155840648,-1.,-1.88742606273259));
#20127=CARTESIAN_POINT('Ctrl Pts',(-0.175274276190844,-1.,-1.892646301985));
#20128=CARTESIAN_POINT('Ctrl Pts',(-0.174879405091263,-1.,-1.89788101117132));
#20129=CARTESIAN_POINT('Ctrl Pts',(-0.174375518661085,-1.,-1.90335253862834));
#20130=CARTESIAN_POINT('Ctrl Pts',(-0.173776635257817,-1.,-1.90911693975267));
#20131=CARTESIAN_POINT('Ctrl Pts',(-0.173090695383496,-1.,-1.91511429159527));
#20132=CARTESIAN_POINT('Ctrl Pts',(-0.172321621259514,-1.,-1.9212233439798));
#20133=CARTESIAN_POINT('Ctrl Pts',(-0.171471191532988,-1.,-1.92731093582036));
#20134=CARTESIAN_POINT('Ctrl Pts',(-0.170541253116202,-1.,-1.93329183155539));
#20135=CARTESIAN_POINT('Ctrl Pts',(-0.169534904817491,-1.,-1.93915639211581));
#20136=CARTESIAN_POINT('Ctrl Pts',(-0.168455741607556,-1.,-1.94493757756931));
#20137=CARTESIAN_POINT('Ctrl Pts',(-0.167307501784475,-1.,-1.95069027794294));
#20138=CARTESIAN_POINT('Ctrl Pts',(-0.166093592002812,-1.,-1.9564675971873));
#20139=CARTESIAN_POINT('Ctrl Pts',(-0.164816568920269,-1.,-1.96229379940136));
#20140=CARTESIAN_POINT('Ctrl Pts',(-0.163478185457734,-1.,-1.96816512677967));
#20141=CARTESIAN_POINT('Ctrl Pts',(-0.162079693556289,-1.,-1.97406280235188));
#20142=CARTESIAN_POINT('Ctrl Pts',(-0.160622060784611,-1.,-1.97996195437559));
#20143=CARTESIAN_POINT('Ctrl Pts',(-0.159106226437299,-1.,-1.98584238283292));
#20144=CARTESIAN_POINT('Ctrl Pts',(-0.157533331459227,-1.,-1.99169810931908));
#20145=CARTESIAN_POINT('Ctrl Pts',(-0.155904629548783,-1.,-1.99753284771497));
#20146=CARTESIAN_POINT('Ctrl Pts',(-0.154221403049722,-1.,-2.00335565310543));
#20147=CARTESIAN_POINT('Ctrl Pts',(-0.15248488362145,-1.,-2.00917680318424));
#20148=CARTESIAN_POINT('Ctrl Pts',(-0.150696157673078,-1.,-2.01500291940238));
#20149=CARTESIAN_POINT('Ctrl Pts',(-0.148856124775337,-1.,-2.02083464969894));
#20150=CARTESIAN_POINT('Ctrl Pts',(-0.146965557332583,-1.,-2.02666926182017));
#20151=CARTESIAN_POINT('Ctrl Pts',(-0.145025140186057,-1.,-2.03250223739942));
#20152=CARTESIAN_POINT('Ctrl Pts',(-0.143035515058209,-1.,-2.03832911025912));
#20153=CARTESIAN_POINT('Ctrl Pts',(-0.140997332152546,-1.,-2.04414757947916));
#20154=CARTESIAN_POINT('Ctrl Pts',(-0.138911255368966,-1.,-2.04995762001328));
#20155=CARTESIAN_POINT('Ctrl Pts',(-0.136777941218044,-1.,-2.05576044414264));
#20156=CARTESIAN_POINT('Ctrl Pts',(-0.134598026192106,-1.,-2.06155781517842));
#20157=CARTESIAN_POINT('Ctrl Pts',(-0.13237211154771,-1.,-2.06735123910326));
#20158=CARTESIAN_POINT('Ctrl Pts',(-0.130100748328403,-1.,-2.07314114713063));
#20159=CARTESIAN_POINT('Ctrl Pts',(-0.12778444527612,-1.,-2.07892715110987));
#20160=CARTESIAN_POINT('Ctrl Pts',(-0.125423679412061,-1.,-2.08470840653643));
#20161=CARTESIAN_POINT('Ctrl Pts',(-0.123018905621083,-1.,-2.09048392424825));
#20162=CARTESIAN_POINT('Ctrl Pts',(-0.120570567965122,-1.,-2.0962529286773));
#20163=CARTESIAN_POINT('Ctrl Pts',(-0.118079107988355,-1.,-2.102015121329));
#20164=CARTESIAN_POINT('Ctrl Pts',(-0.115544957687926,-1.,-2.10777050261309));
#20165=CARTESIAN_POINT('Ctrl Pts',(-0.112968534419737,-1.,-2.11351924490306));
#20166=CARTESIAN_POINT('Ctrl Pts',(-0.110350236135025,-1.,-2.11926155590865));
#20167=CARTESIAN_POINT('Ctrl Pts',(-0.10769043523109,-1.,-2.12499752307));
#20168=CARTESIAN_POINT('Ctrl Pts',(-0.104989479152739,-1.,-2.13072704887293));
#20169=CARTESIAN_POINT('Ctrl Pts',(-0.1022477005561,-1.,-2.13644992667165));
#20170=CARTESIAN_POINT('Ctrl Pts',(-0.0994654261990915,-1.,-2.14216588396025));
#20171=CARTESIAN_POINT('Ctrl Pts',(-0.0966429852305459,-1.,-2.14787463531795));
#20172=CARTESIAN_POINT('Ctrl Pts',(-0.0937807218867643,-1.,-2.1535759397817));
#20173=CARTESIAN_POINT('Ctrl Pts',(-0.0908789888107265,-1.,-2.15926961544516));
#20174=CARTESIAN_POINT('Ctrl Pts',(-0.0879381291386923,-1.,-2.16495552645014));
#20175=CARTESIAN_POINT('Ctrl Pts',(-0.0849584620835372,-1.,-2.17063357870952));
#20176=CARTESIAN_POINT('Ctrl Pts',(-0.0819402680872765,-1.,-2.176303712113));
#20177=CARTESIAN_POINT('Ctrl Pts',(-0.0788837727685243,-1.,-2.18196589448887));
#20178=CARTESIAN_POINT('Ctrl Pts',(-0.0757891465836148,-1.,-2.1876201139953));
#20179=CARTESIAN_POINT('Ctrl Pts',(-0.0732830357306725,-1.,-2.19213712013662));
#20180=CARTESIAN_POINT('Ctrl Pts',(-0.0713863779526154,-1.,-2.19552129484002));
#20181=CARTESIAN_POINT('Ctrl Pts',(-0.070114353632549,-1.,-2.19777582085423));
#20182=CARTESIAN_POINT('Ctrl Pts',(-0.0694764450219581,-1.,-2.19890268624765));
#20183=CARTESIAN_POINT('',(0.0694764450219584,-1.,-2.19890268624765));
#20184=CARTESIAN_POINT('',(-0.0694764450219581,-1.,-2.19890268624765));
#20185=CARTESIAN_POINT('',(0.163289472382896,-1.,-1.74236521665491));
#20186=CARTESIAN_POINT('Ctrl Pts',(0.0694764450219584,-1.,-2.19890268624765));
#20187=CARTESIAN_POINT('Ctrl Pts',(0.0701143536324926,-1.,-2.19777582085261));
#20188=CARTESIAN_POINT('Ctrl Pts',(0.0713863779524627,-1.,-2.19552129483562));
#20189=CARTESIAN_POINT('Ctrl Pts',(0.0732830357304276,-1.,-2.19213712012956));
#20190=CARTESIAN_POINT('Ctrl Pts',(0.0757891465833411,-1.,-2.1876201139874));
#20191=CARTESIAN_POINT('Ctrl Pts',(0.0788837727683228,-1.,-2.18196589448304));
#20192=CARTESIAN_POINT('Ctrl Pts',(0.0819402680871939,-1.,-2.1763037121106));
#20193=CARTESIAN_POINT('Ctrl Pts',(0.0849584620835643,-1.,-2.17063357871031));
#20194=CARTESIAN_POINT('Ctrl Pts',(0.0879381291387823,-1.,-2.16495552645275));
#20195=CARTESIAN_POINT('Ctrl Pts',(0.0908789888108266,-1.,-2.15926961544808));
#20196=CARTESIAN_POINT('Ctrl Pts',(0.0937807218868345,-1.,-2.15357593978377));
#20197=CARTESIAN_POINT('Ctrl Pts',(0.0966429852305689,-1.,-2.14787463531864));
#20198=CARTESIAN_POINT('Ctrl Pts',(0.0994654261990743,-1.,-2.14216588395974));
#20199=CARTESIAN_POINT('Ctrl Pts',(0.102247700556064,-1.,-2.13644992667052));
#20200=CARTESIAN_POINT('Ctrl Pts',(0.104989479152703,-1.,-2.1307270488718));
#20201=CARTESIAN_POINT('Ctrl Pts',(0.107690435231068,-1.,-2.12499752306927));
#20202=CARTESIAN_POINT('Ctrl Pts',(0.11035023613502,-1.,-2.11926155590849));
#20203=CARTESIAN_POINT('Ctrl Pts',(0.112968534419746,-1.,-2.11351924490335));
#20204=CARTESIAN_POINT('Ctrl Pts',(0.11554495768794,-1.,-2.10777050261359));
#20205=CARTESIAN_POINT('Ctrl Pts',(0.118079107988368,-1.,-2.10201512132945));
#20206=CARTESIAN_POINT('Ctrl Pts',(0.120570567965129,-1.,-2.09625292867756));
#20207=CARTESIAN_POINT('Ctrl Pts',(0.123018905621083,-1.,-2.09048392424826));
#20208=CARTESIAN_POINT('Ctrl Pts',(0.125423679412058,-1.,-2.08470840653628));
#20209=CARTESIAN_POINT('Ctrl Pts',(0.127784445276116,-1.,-2.07892715110967));
#20210=CARTESIAN_POINT('Ctrl Pts',(0.1301007483284,-1.,-2.07314114713047));
#20211=CARTESIAN_POINT('Ctrl Pts',(0.13237211154771,-1.,-2.06735123910319));
#20212=CARTESIAN_POINT('Ctrl Pts',(0.134598026192107,-1.,-2.06155781517844));
#20213=CARTESIAN_POINT('Ctrl Pts',(0.136777941218044,-1.,-2.0557604441427));
#20214=CARTESIAN_POINT('Ctrl Pts',(0.138911255368966,-1.,-2.04995762001333));
#20215=CARTESIAN_POINT('Ctrl Pts',(0.140997332152545,-1.,-2.04414757947919));
#20216=CARTESIAN_POINT('Ctrl Pts',(0.143035515058208,-1.,-2.03832911025913));
#20217=CARTESIAN_POINT('Ctrl Pts',(0.145025140186058,-1.,-2.03250223739941));
#20218=CARTESIAN_POINT('Ctrl Pts',(0.146965557332586,-1.,-2.02666926182017));
#20219=CARTESIAN_POINT('Ctrl Pts',(0.148856124775343,-1.,-2.02083464969897));
#20220=CARTESIAN_POINT('Ctrl Pts',(0.150696157673084,-1.,-2.01500291940243));
#20221=CARTESIAN_POINT('Ctrl Pts',(0.152484883621452,-1.,-2.00917680318426));
#20222=CARTESIAN_POINT('Ctrl Pts',(0.154221403049719,-1.,-2.00335565310539));
#20223=CARTESIAN_POINT('Ctrl Pts',(0.155904629548774,-1.,-1.99753284771487));
#20224=CARTESIAN_POINT('Ctrl Pts',(0.157533331459215,-1.,-1.99169810931893));
#20225=CARTESIAN_POINT('Ctrl Pts',(0.159106226437288,-1.,-1.98584238283279));
#20226=CARTESIAN_POINT('Ctrl Pts',(0.16062206078461,-1.,-1.97996195437557));
#20227=CARTESIAN_POINT('Ctrl Pts',(0.162079693556302,-1.,-1.97406280235204));
#20228=CARTESIAN_POINT('Ctrl Pts',(0.16347818545776,-1.,-1.96816512678));
#20229=CARTESIAN_POINT('Ctrl Pts',(0.1648165689203,-1.,-1.96229379940174));
#20230=CARTESIAN_POINT('Ctrl Pts',(0.166093592002833,-1.,-1.95646759718755));
#20231=CARTESIAN_POINT('Ctrl Pts',(0.167307501784469,-1.,-1.95069027794286));
#20232=CARTESIAN_POINT('Ctrl Pts',(0.168455741607516,-1.,-1.94493757756879));
#20233=CARTESIAN_POINT('Ctrl Pts',(0.169534904817425,-1.,-1.93915639211497));
#20234=CARTESIAN_POINT('Ctrl Pts',(0.170541253116136,-1.,-1.93329183155455));
#20235=CARTESIAN_POINT('Ctrl Pts',(0.17147119153296,-1.,-1.92731093582));
#20236=CARTESIAN_POINT('Ctrl Pts',(0.172321621259557,-1.,-1.92122334398034));
#20237=CARTESIAN_POINT('Ctrl Pts',(0.173090695383619,-1.,-1.91511429159681));
#20238=CARTESIAN_POINT('Ctrl Pts',(0.173776635257984,-1.,-1.90911693975475));
#20239=CARTESIAN_POINT('Ctrl Pts',(0.174375518661222,-1.,-1.90335253863003));
#20240=CARTESIAN_POINT('Ctrl Pts',(0.174879405091277,-1.,-1.89788101117148));
#20241=CARTESIAN_POINT('Ctrl Pts',(0.175274276190664,-1.,-1.89264630198279));
#20242=CARTESIAN_POINT('Ctrl Pts',(0.175538155840286,-1.,-1.88742606272818));
#20243=CARTESIAN_POINT('Ctrl Pts',(0.175644148889271,-1.,-1.88188663144846));
#20244=CARTESIAN_POINT('Ctrl Pts',(0.175563480746205,-1.,-1.87563767773249));
#20245=CARTESIAN_POINT('Ctrl Pts',(0.175268337590901,-1.,-1.86828349694972));
#20246=CARTESIAN_POINT('Ctrl Pts',(0.174735259276856,-1.,-1.85948367089838));
#20247=CARTESIAN_POINT('Ctrl Pts',(0.173946627589401,-1.,-1.84898113200543));
#20248=CARTESIAN_POINT('Ctrl Pts',(0.17288944289442,-1.,-1.83658380530747));
#20249=CARTESIAN_POINT('Ctrl Pts',(0.171554770207306,-1.,-1.82215766815414));
#20250=CARTESIAN_POINT('Ctrl Pts',(0.169936923908078,-1.,-1.80561530633924));
#20251=CARTESIAN_POINT('Ctrl Pts',(0.16803277280837,-1.,-1.78690649988931));
#20252=CARTESIAN_POINT('Ctrl Pts',(0.166279355148738,-1.,-1.77018771687692));
#20253=CARTESIAN_POINT('Ctrl Pts',(0.164834765708484,-1.,-1.75666056640041));
#20254=CARTESIAN_POINT('Ctrl Pts',(0.163814161002474,-1.,-1.74720349503904));
#20255=CARTESIAN_POINT('Ctrl Pts',(0.163289472382896,-1.,-1.74236521665491));
#20256=CARTESIAN_POINT('',(0.383122945602004,-1.,-1.7075470150345));
#20257=CARTESIAN_POINT('Origin',(0.,-1.,0.));
#20258=CARTESIAN_POINT('',(0.61342227326009,-1.,-2.11275013067528));
#20259=CARTESIAN_POINT('Ctrl Pts',(0.383122945602004,-1.,-1.7075470150345));
#20260=CARTESIAN_POINT('Ctrl Pts',(0.384119047314215,-1.,-1.71231062891398));
#20261=CARTESIAN_POINT('Ctrl Pts',(0.386070790323281,-1.,-1.72162022244582));
#20262=CARTESIAN_POINT('Ctrl Pts',(0.388877023502615,-1.,-1.73493170972829));
#20263=CARTESIAN_POINT('Ctrl Pts',(0.392375812285395,-1.,-1.75137405310193));
#20264=CARTESIAN_POINT('Ctrl Pts',(0.396346196110688,-1.,-1.76975560043442));
#20265=CARTESIAN_POINT('Ctrl Pts',(0.399919403774155,-1.,-1.78598826343754));
#20266=CARTESIAN_POINT('Ctrl Pts',(0.403107976163396,-1.,-1.80012077173238));
#20267=CARTESIAN_POINT('Ctrl Pts',(0.405933518407175,-1.,-1.81223801812013));
#20268=CARTESIAN_POINT('Ctrl Pts',(0.408428948106227,-1.,-1.82247022677562));
#20269=CARTESIAN_POINT('Ctrl Pts',(0.410641256301276,-1.,-1.83100408895047));
#20270=CARTESIAN_POINT('Ctrl Pts',(0.412633125322945,-1.,-1.8380895347617));
#20271=CARTESIAN_POINT('Ctrl Pts',(0.414487438255542,-1.,-1.84405757074218));
#20272=CARTESIAN_POINT('Ctrl Pts',(0.416300022039885,-1.,-1.84929312930314));
#20273=CARTESIAN_POINT('Ctrl Pts',(0.418164129144045,-1.,-1.8541763285645));
#20274=CARTESIAN_POINT('Ctrl Pts',(0.420157287975583,-1.,-1.8590328109667));
#20275=CARTESIAN_POINT('Ctrl Pts',(0.422327307417884,-1.,-1.86408083333863));
#20276=CARTESIAN_POINT('Ctrl Pts',(0.424678177290876,-1.,-1.8693780394412));
#20277=CARTESIAN_POINT('Ctrl Pts',(0.427183828518743,-1.,-1.87486989291334));
#20278=CARTESIAN_POINT('Ctrl Pts',(0.429803062482217,-1.,-1.88044229001779));
#20279=CARTESIAN_POINT('Ctrl Pts',(0.432493038548833,-1.,-1.88596913666828));
#20280=CARTESIAN_POINT('Ctrl Pts',(0.43522566096358,-1.,-1.89136993975585));
#20281=CARTESIAN_POINT('Ctrl Pts',(0.437995003948443,-1.,-1.89663648956549));
#20282=CARTESIAN_POINT('Ctrl Pts',(0.44080783370416,-1.,-1.90180124389137));
#20283=CARTESIAN_POINT('Ctrl Pts',(0.44367755684917,-1.,-1.90691756144906));
#20284=CARTESIAN_POINT('Ctrl Pts',(0.446617343485651,-1.,-1.91203699981095));
#20285=CARTESIAN_POINT('Ctrl Pts',(0.449632260106572,-1.,-1.91718342555717));
#20286=CARTESIAN_POINT('Ctrl Pts',(0.452719478359356,-1.,-1.9223538064847));
#20287=CARTESIAN_POINT('Ctrl Pts',(0.455872005174335,-1.,-1.92753067150461));
#20288=CARTESIAN_POINT('Ctrl Pts',(0.459081234547931,-1.,-1.93269066517936));
#20289=CARTESIAN_POINT('Ctrl Pts',(0.462340031009087,-1.,-1.93781486640834));
#20290=CARTESIAN_POINT('Ctrl Pts',(0.465645462026064,-1.,-1.94289794196205));
#20291=CARTESIAN_POINT('Ctrl Pts',(0.468997482913158,-1.,-1.94794381136524));
#20292=CARTESIAN_POINT('Ctrl Pts',(0.472397672264079,-1.,-1.95296148278136));
#20293=CARTESIAN_POINT('Ctrl Pts',(0.475848034683171,-1.,-1.95796111148175));
#20294=CARTESIAN_POINT('Ctrl Pts',(0.479349583074846,-1.,-1.96294933055938));
#20295=CARTESIAN_POINT('Ctrl Pts',(0.482901662120686,-1.,-1.96792703422358));
#20296=CARTESIAN_POINT('Ctrl Pts',(0.486502692907661,-1.,-1.97289186263272));
#20297=CARTESIAN_POINT('Ctrl Pts',(0.490150627860955,-1.,-1.97783973019229));
#20298=CARTESIAN_POINT('Ctrl Pts',(0.493843476541492,-1.,-1.9827665876182));
#20299=CARTESIAN_POINT('Ctrl Pts',(0.497579909545564,-1.,-1.98767044752929));
#20300=CARTESIAN_POINT('Ctrl Pts',(0.501359287727129,-1.,-1.9925514912615));
#20301=CARTESIAN_POINT('Ctrl Pts',(0.505181361323011,-1.,-1.99741107463567));
#20302=CARTESIAN_POINT('Ctrl Pts',(0.509046069886152,-1.,-2.00225107134733));
#20303=CARTESIAN_POINT('Ctrl Pts',(0.512953306961813,-1.,-2.00707309946955));
#20304=CARTESIAN_POINT('Ctrl Pts',(0.516902681728733,-1.,-2.01187773939257));
#20305=CARTESIAN_POINT('Ctrl Pts',(0.520893590399428,-1.,-2.01666477917306));
#20306=CARTESIAN_POINT('Ctrl Pts',(0.524925318333518,-1.,-2.02143356304712));
#20307=CARTESIAN_POINT('Ctrl Pts',(0.52899712724191,-1.,-2.02618329083289));
#20308=CARTESIAN_POINT('Ctrl Pts',(0.533108355132905,-1.,-2.03091336214401));
#20309=CARTESIAN_POINT('Ctrl Pts',(0.537258489833134,-1.,-2.03562362953993));
#20310=CARTESIAN_POINT('Ctrl Pts',(0.54144712061552,-1.,-2.0403142269048));
#20311=CARTESIAN_POINT('Ctrl Pts',(0.545673903817348,-1.,-2.0449854471456));
#20312=CARTESIAN_POINT('Ctrl Pts',(0.549938525150342,-1.,-2.04963761077974));
#20313=CARTESIAN_POINT('Ctrl Pts',(0.554240657464109,-1.,-2.05427091604482));
#20314=CARTESIAN_POINT('Ctrl Pts',(0.558579940185467,-1.,-2.05888537756571));
#20315=CARTESIAN_POINT('Ctrl Pts',(0.562955993082574,-1.,-2.06348090160697));
#20316=CARTESIAN_POINT('Ctrl Pts',(0.567368421181229,-1.,-2.06805732997383));
#20317=CARTESIAN_POINT('Ctrl Pts',(0.571816823242411,-1.,-2.07261449292758));
#20318=CARTESIAN_POINT('Ctrl Pts',(0.576300797416274,-1.,-2.07715226767361));
#20319=CARTESIAN_POINT('Ctrl Pts',(0.580819952107256,-1.,-2.08167059018138));
#20320=CARTESIAN_POINT('Ctrl Pts',(0.585373918990895,-1.,-2.086169437277));
#20321=CARTESIAN_POINT('Ctrl Pts',(0.589962365403189,-1.,-2.09064881812053));
#20322=CARTESIAN_POINT('Ctrl Pts',(0.594585006052823,-1.,-2.09510876220501));
#20323=CARTESIAN_POINT('Ctrl Pts',(0.599241616422144,-1.,-2.09954930865331));
#20324=CARTESIAN_POINT('Ctrl Pts',(0.603932030738212,-1.,-2.10397049887709));
#20325=CARTESIAN_POINT('Ctrl Pts',(0.607711315456826,-1.,-2.10749199615859));
#20326=CARTESIAN_POINT('Ctrl Pts',(0.610560911691113,-1.,-2.11012443807661));
#20327=CARTESIAN_POINT('Ctrl Pts',(0.61246736556225,-1.,-2.11187554260142));
#20328=CARTESIAN_POINT('Ctrl Pts',(0.61342227326009,-1.,-2.11275013067528));
#20329=CARTESIAN_POINT('',(0.745574324794401,-1.,-2.0698113262342));
#20330=CARTESIAN_POINT('',(0.61342227326009,-1.,-2.11275013067528));
#20331=CARTESIAN_POINT('',(0.693717979106306,-1.,-1.60662857109684));
#20332=CARTESIAN_POINT('Ctrl Pts',(0.745574324794401,-1.,-2.0698113262342));
#20333=CARTESIAN_POINT('Ctrl Pts',(0.74583279137781,-1.,-2.06854248895575));
#20334=CARTESIAN_POINT('Ctrl Pts',(0.746345871542695,-1.,-2.06600523016401));
#20335=CARTESIAN_POINT('Ctrl Pts',(0.747103932785504,-1.,-2.06220058927162));
#20336=CARTESIAN_POINT('Ctrl Pts',(0.748091554181101,-1.,-2.05713023030263));
#20337=CARTESIAN_POINT('Ctrl Pts',(0.749287468663053,-1.,-2.05079645591606));
#20338=CARTESIAN_POINT('Ctrl Pts',(0.750444657874758,-1.,-2.04446689147754));
#20339=CARTESIAN_POINT('Ctrl Pts',(0.751562963361383,-1.,-2.03814160092173));
#20340=CARTESIAN_POINT('Ctrl Pts',(0.752642180488104,-1.,-2.03182068456467));
#20341=CARTESIAN_POINT('Ctrl Pts',(0.753682061113765,-1.,-2.02550428623587));
#20342=CARTESIAN_POINT('Ctrl Pts',(0.75468233072352,-1.,-2.01919259406003));
#20343=CARTESIAN_POINT('Ctrl Pts',(0.7556427049581,-1.,-2.01288584328149));
#20344=CARTESIAN_POINT('Ctrl Pts',(0.756562904646496,-1.,-2.00658431587682));
#20345=CARTESIAN_POINT('Ctrl Pts',(0.757442676862341,-1.,-2.00028834739072));
#20346=CARTESIAN_POINT('Ctrl Pts',(0.758281796766377,-1.,-1.9939983109871));
#20347=CARTESIAN_POINT('Ctrl Pts',(0.759080037802242,-1.,-1.98771456680806));
#20348=CARTESIAN_POINT('Ctrl Pts',(0.759837147452135,-1.,-1.98143741418156));
#20349=CARTESIAN_POINT('Ctrl Pts',(0.760552825409855,-1.,-1.97516705321521));
#20350=CARTESIAN_POINT('Ctrl Pts',(0.761226690483986,-1.,-1.96890351582545));
#20351=CARTESIAN_POINT('Ctrl Pts',(0.761858300014575,-1.,-1.96264672744229));
#20352=CARTESIAN_POINT('Ctrl Pts',(0.762447203806263,-1.,-1.95639665309893));
#20353=CARTESIAN_POINT('Ctrl Pts',(0.762992990878774,-1.,-1.95015342590025));
#20354=CARTESIAN_POINT('Ctrl Pts',(0.76349533353858,-1.,-1.94391746617626));
#20355=CARTESIAN_POINT('Ctrl Pts',(0.763954049121393,-1.,-1.93768964875867));
#20356=CARTESIAN_POINT('Ctrl Pts',(0.764369010673889,-1.,-1.93147105496367));
#20357=CARTESIAN_POINT('Ctrl Pts',(0.764740025488189,-1.,-1.92526263537041));
#20358=CARTESIAN_POINT('Ctrl Pts',(0.765066729667095,-1.,-1.91906491634197));
#20359=CARTESIAN_POINT('Ctrl Pts',(0.765348465884739,-1.,-1.91287765805174));
#20360=CARTESIAN_POINT('Ctrl Pts',(0.765584196937936,-1.,-1.90669961402362));
#20361=CARTESIAN_POINT('Ctrl Pts',(0.765772772593395,-1.,-1.90052930393599));
#20362=CARTESIAN_POINT('Ctrl Pts',(0.765913193856979,-1.,-1.89436577771389));
#20363=CARTESIAN_POINT('Ctrl Pts',(0.76600483706209,-1.,-1.88820926433409));
#20364=CARTESIAN_POINT('Ctrl Pts',(0.766047794851868,-1.,-1.88206215302561));
#20365=CARTESIAN_POINT('Ctrl Pts',(0.766042837036759,-1.,-1.87592888967886));
#20366=CARTESIAN_POINT('Ctrl Pts',(0.765990708546111,-1.,-1.86981398314345));
#20367=CARTESIAN_POINT('Ctrl Pts',(0.765891519092557,-1.,-1.86372027063315));
#20368=CARTESIAN_POINT('Ctrl Pts',(0.765744212909305,-1.,-1.85764741390391));
#20369=CARTESIAN_POINT('Ctrl Pts',(0.765545710619023,-1.,-1.85158945130054));
#20370=CARTESIAN_POINT('Ctrl Pts',(0.765291664861971,-1.,-1.84553698875911));
#20371=CARTESIAN_POINT('Ctrl Pts',(0.764978057881687,-1.,-1.83948181064823));
#20372=CARTESIAN_POINT('Ctrl Pts',(0.764602549687845,-1.,-1.8334207722714));
#20373=CARTESIAN_POINT('Ctrl Pts',(0.764165902606055,-1.,-1.8273599120008));
#20374=CARTESIAN_POINT('Ctrl Pts',(0.763673465462854,-1.,-1.82131873145297));
#20375=CARTESIAN_POINT('Ctrl Pts',(0.763132003836783,-1.,-1.81532118405566));
#20376=CARTESIAN_POINT('Ctrl Pts',(0.762546129464036,-1.,-1.80938551463989));
#20377=CARTESIAN_POINT('Ctrl Pts',(0.761915336443515,-1.,-1.80351583877334));
#20378=CARTESIAN_POINT('Ctrl Pts',(0.761229695230359,-1.,-1.79768986997735));
#20379=CARTESIAN_POINT('Ctrl Pts',(0.760469555880425,-1.,-1.79185815610802));
#20380=CARTESIAN_POINT('Ctrl Pts',(0.759614401109868,-1.,-1.78596964884527));
#20381=CARTESIAN_POINT('Ctrl Pts',(0.75865062667738,-1.,-1.77999411220912));
#20382=CARTESIAN_POINT('Ctrl Pts',(0.757578264077238,-1.,-1.77394167108342));
#20383=CARTESIAN_POINT('Ctrl Pts',(0.756421896028403,-1.,-1.76789396003141));
#20384=CARTESIAN_POINT('Ctrl Pts',(0.755220979975262,-1.,-1.7619781724032));
#20385=CARTESIAN_POINT('Ctrl Pts',(0.75400925402848,-1.,-1.75631083600175));
#20386=CARTESIAN_POINT('Ctrl Pts',(0.752797683531377,-1.,-1.75095139468809));
#20387=CARTESIAN_POINT('Ctrl Pts',(0.751555614163629,-1.,-1.74585086852298));
#20388=CARTESIAN_POINT('Ctrl Pts',(0.75019343597954,-1.,-1.74080458266705));
#20389=CARTESIAN_POINT('Ctrl Pts',(0.748582462954854,-1.,-1.73550351679848));
#20390=CARTESIAN_POINT('Ctrl Pts',(0.746574710096436,-1.,-1.72958533647399));
#20391=CARTESIAN_POINT('Ctrl Pts',(0.744021445433764,-1.,-1.7226822991693));
#20392=CARTESIAN_POINT('Ctrl Pts',(0.740795162032087,-1.,-1.71447789751927));
#20393=CARTESIAN_POINT('Ctrl Pts',(0.736799665724771,-1.,-1.70473309006121));
#20394=CARTESIAN_POINT('Ctrl Pts',(0.731963238697195,-1.,-1.69326921975743));
#20395=CARTESIAN_POINT('Ctrl Pts',(0.726235967997433,-1.,-1.67996158455503));
#20396=CARTESIAN_POINT('Ctrl Pts',(0.719585433804282,-1.,-1.6647288055568));
#20397=CARTESIAN_POINT('Ctrl Pts',(0.711993139355394,-1.,-1.64752408832016));
#20398=CARTESIAN_POINT('Ctrl Pts',(0.705159151988319,-1.,-1.63216541664676));
#20399=CARTESIAN_POINT('Ctrl Pts',(0.699605146405088,-1.,-1.61974673472612));
#20400=CARTESIAN_POINT('Ctrl Pts',(0.695712097881194,-1.,-1.61106790958151));
#20401=CARTESIAN_POINT('Ctrl Pts',(0.693717979106306,-1.,-1.60662857109684));
#20402=CARTESIAN_POINT('',(0.892032620296855,-1.,-1.5055822144029));
#20403=CARTESIAN_POINT('Origin',(0.,-1.,0.));
#20404=CARTESIAN_POINT('',(1.23627494547115,-1.,-1.81978687191668));
#20405=CARTESIAN_POINT('Ctrl Pts',(0.892032620296855,-1.,-1.5055822144029));
#20406=CARTESIAN_POINT('Ctrl Pts',(0.894452006964543,-1.,-1.50980486806688));
#20407=CARTESIAN_POINT('Ctrl Pts',(0.89918504748351,-1.,-1.51805569590094));
#20408=CARTESIAN_POINT('Ctrl Pts',(0.905967409625651,-1.,-1.52984849887993));
#20409=CARTESIAN_POINT('Ctrl Pts',(0.914375919026456,-1.,-1.54440491149498));
#20410=CARTESIAN_POINT('Ctrl Pts',(0.923832188944341,-1.,-1.56065988578893));
#20411=CARTESIAN_POINT('Ctrl Pts',(0.932246680108685,-1.,-1.57499388382243));
#20412=CARTESIAN_POINT('Ctrl Pts',(0.939646377893399,-1.,-1.58744937487176));
#20413=CARTESIAN_POINT('Ctrl Pts',(0.946078063315257,-1.,-1.59810042043673));
#20414=CARTESIAN_POINT('Ctrl Pts',(0.951613284356035,-1.,-1.60706069896936));
#20415=CARTESIAN_POINT('Ctrl Pts',(0.95635442292067,-1.,-1.61449324337085));
#20416=CARTESIAN_POINT('Ctrl Pts',(0.960438326101728,-1.,-1.62061638140221));
#20417=CARTESIAN_POINT('Ctrl Pts',(0.964046107040535,-1.,-1.62571930670187));
#20418=CARTESIAN_POINT('Ctrl Pts',(0.967387853230345,-1.,-1.63013849959462));
#20419=CARTESIAN_POINT('Ctrl Pts',(0.970669715997509,-1.,-1.63420665729798));
#20420=CARTESIAN_POINT('Ctrl Pts',(0.974066058287418,-1.,-1.63820952658144));
#20421=CARTESIAN_POINT('Ctrl Pts',(0.977689794119416,-1.,-1.64233990826687));
#20422=CARTESIAN_POINT('Ctrl Pts',(0.981562530939489,-1.,-1.64665139190656));
#20423=CARTESIAN_POINT('Ctrl Pts',(0.98564262292082,-1.,-1.65110016612638));
#20424=CARTESIAN_POINT('Ctrl Pts',(0.989855627854164,-1.,-1.65559044289699));
#20425=CARTESIAN_POINT('Ctrl Pts',(0.994121836661305,-1.,-1.66001553809947));
#20426=CARTESIAN_POINT('Ctrl Pts',(0.998389654952757,-1.,-1.66430758030376));
#20427=CARTESIAN_POINT('Ctrl Pts',(1.00265091003727,-1.,-1.66846059277303));
#20428=CARTESIAN_POINT('Ctrl Pts',(1.00692206696414,-1.,-1.67250335383293));
#20429=CARTESIAN_POINT('Ctrl Pts',(1.01123236493511,-1.,-1.67648246776464));
#20430=CARTESIAN_POINT('Ctrl Pts',(1.01561026162773,-1.,-1.68044289894798));
#20431=CARTESIAN_POINT('Ctrl Pts',(1.02006795074201,-1.,-1.68440578021706));
#20432=CARTESIAN_POINT('Ctrl Pts',(1.02460180535255,-1.,-1.68836910178447));
#20433=CARTESIAN_POINT('Ctrl Pts',(1.02919977579147,-1.,-1.69231840863458));
#20434=CARTESIAN_POINT('Ctrl Pts',(1.03384646003588,-1.,-1.69623414782771));
#20435=CARTESIAN_POINT('Ctrl Pts',(1.03852922490789,-1.,-1.70010052930962));
#20436=CARTESIAN_POINT('Ctrl Pts',(1.04324363334554,-1.,-1.70391338707982));
#20437=CARTESIAN_POINT('Ctrl Pts',(1.04799085404995,-1.,-1.70767646263649));
#20438=CARTESIAN_POINT('Ctrl Pts',(1.05277517202855,-1.,-1.71139783543989));
#20439=CARTESIAN_POINT('Ctrl Pts',(1.05760163192479,-1.,-1.7150865442702));
#20440=CARTESIAN_POINT('Ctrl Pts',(1.06247324680647,-1.,-1.71874858456904));
#20441=CARTESIAN_POINT('Ctrl Pts',(1.06738966975462,-1.,-1.72238500928453));
#20442=CARTESIAN_POINT('Ctrl Pts',(1.07234866990252,-1.,-1.72599406198488));
#20443=CARTESIAN_POINT('Ctrl Pts',(1.0773470373727,-1.,-1.72957248977424));
#20444=CARTESIAN_POINT('Ctrl Pts',(1.08238162784749,-1.,-1.73311705663407));
#20445=CARTESIAN_POINT('Ctrl Pts',(1.08745056285427,-1.,-1.73662628326091));
#20446=CARTESIAN_POINT('Ctrl Pts',(1.09255329056493,-1.,-1.74010053962247));
#20447=CARTESIAN_POINT('Ctrl Pts',(1.09768999241225,-1.,-1.74354119236208));
#20448=CARTESIAN_POINT('Ctrl Pts',(1.10286118991143,-1.,-1.74695004214923));
#20449=CARTESIAN_POINT('Ctrl Pts',(1.10806728183007,-1.,-1.7503286607592));
#20450=CARTESIAN_POINT('Ctrl Pts',(1.11330807582551,-1.,-1.7536777209463));
#20451=CARTESIAN_POINT('Ctrl Pts',(1.11858293216763,-1.,-1.75699720772105));
#20452=CARTESIAN_POINT('Ctrl Pts',(1.12389096855086,-1.,-1.76028671825096));
#20453=CARTESIAN_POINT('Ctrl Pts',(1.12923123555075,-1.,-1.7635457196617));
#20454=CARTESIAN_POINT('Ctrl Pts',(1.1346029180462,-1.,-1.76677384551862));
#20455=CARTESIAN_POINT('Ctrl Pts',(1.14000548336975,-1.,-1.76997111386769));
#20456=CARTESIAN_POINT('Ctrl Pts',(1.1454385822692,-1.,-1.77313777896194));
#20457=CARTESIAN_POINT('Ctrl Pts',(1.15090197841514,-1.,-1.7762742255701));
#20458=CARTESIAN_POINT('Ctrl Pts',(1.15639547194698,-1.,-1.77938085564275));
#20459=CARTESIAN_POINT('Ctrl Pts',(1.16191881298499,-1.,-1.78245795881009));
#20460=CARTESIAN_POINT('Ctrl Pts',(1.16747166312303,-1.,-1.78550566040443));
#20461=CARTESIAN_POINT('Ctrl Pts',(1.17305363177328,-1.,-1.78852398877617));
#20462=CARTESIAN_POINT('Ctrl Pts',(1.17866429440809,-1.,-1.79151291552689));
#20463=CARTESIAN_POINT('Ctrl Pts',(1.18430321697432,-1.,-1.79447240321515));
#20464=CARTESIAN_POINT('Ctrl Pts',(1.18996997934445,-1.,-1.79740245923478));
#20465=CARTESIAN_POINT('Ctrl Pts',(1.19566418930242,-1.,-1.80030314369879));
#20466=CARTESIAN_POINT('Ctrl Pts',(1.20138548938974,-1.,-1.80317454838603));
#20467=CARTESIAN_POINT('Ctrl Pts',(1.20713356605475,-1.,-1.80601678480707));
#20468=CARTESIAN_POINT('Ctrl Pts',(1.21290815708314,-1.,-1.80882996917129));
#20469=CARTESIAN_POINT('Ctrl Pts',(1.21870906103557,-1.,-1.81161420806656));
#20470=CARTESIAN_POINT('Ctrl Pts',(1.2245361330495,-1.,-1.81436959210434));
#20471=CARTESIAN_POINT('Ctrl Pts',(1.2292186489137,-1.,-1.8165508718364));
#20472=CARTESIAN_POINT('Ctrl Pts',(1.2327422452705,-1.,-1.81817389921279));
#20473=CARTESIAN_POINT('Ctrl Pts',(1.23509651170476,-1.,-1.81925017193666));
#20474=CARTESIAN_POINT('Ctrl Pts',(1.23627494547115,-1.,-1.81978687191668));
#20475=CARTESIAN_POINT('',(1.34869019493419,-1.,-1.73811241238545));
#20476=CARTESIAN_POINT('',(1.23627494547115,-1.,-1.81978687191668));
#20477=CARTESIAN_POINT('',(1.15624053661742,-1.,-1.31362392696032));
#20478=CARTESIAN_POINT('Ctrl Pts',(1.34869019493419,-1.,-1.73811241238545));
#20479=CARTESIAN_POINT('Ctrl Pts',(1.34854391898045,-1.,-1.73682580585691));
#20480=CARTESIAN_POINT('Ctrl Pts',(1.34824783112887,-1.,-1.73425417885907));
#20481=CARTESIAN_POINT('Ctrl Pts',(1.34779309152035,-1.,-1.7304014965394));
#20482=CARTESIAN_POINT('Ctrl Pts',(1.34716554819527,-1.,-1.72527410680674));
#20483=CARTESIAN_POINT('Ctrl Pts',(1.34634568653227,-1.,-1.7188807715049));
#20484=CARTESIAN_POINT('Ctrl Pts',(1.34549029589416,-1.,-1.71250340686822));
#20485=CARTESIAN_POINT('Ctrl Pts',(1.34459924533831,-1.,-1.70614212266738));
#20486=CARTESIAN_POINT('Ctrl Pts',(1.34367237124483,-1.,-1.69979707754427));
#20487=CARTESIAN_POINT('Ctrl Pts',(1.34270948206319,-1.,-1.6934684849687));
#20488=CARTESIAN_POINT('Ctrl Pts',(1.341710374848,-1.,-1.68715660868764));
#20489=CARTESIAN_POINT('Ctrl Pts',(1.34067485185203,-1.,-1.68086176030362));
#20490=CARTESIAN_POINT('Ctrl Pts',(1.3396027347034,-1.,-1.67458429426086));
#20491=CARTESIAN_POINT('Ctrl Pts',(1.33849388654388,-1.,-1.66832460783989));
#20492=CARTESIAN_POINT('Ctrl Pts',(1.33734820885262,-1.,-1.66208312541983));
#20493=CARTESIAN_POINT('Ctrl Pts',(1.33616559745172,-1.,-1.65586025952593));
#20494=CARTESIAN_POINT('Ctrl Pts',(1.33494590467993,-1.,-1.6496563728683));
#20495=CARTESIAN_POINT('Ctrl Pts',(1.33368890676572,-1.,-1.6434717485603));
#20496=CARTESIAN_POINT('Ctrl Pts',(1.33239425103724,-1.,-1.63730653475089));
#20497=CARTESIAN_POINT('Ctrl Pts',(1.33106149345645,-1.,-1.63116079730923));
#20498=CARTESIAN_POINT('Ctrl Pts',(1.3296901950568,-1.,-1.62503464209797));
#20499=CARTESIAN_POINT('Ctrl Pts',(1.32828000610449,-1.,-1.61892832270724));
#20500=CARTESIAN_POINT('Ctrl Pts',(1.32683074483356,-1.,-1.6128423401575));
#20501=CARTESIAN_POINT('Ctrl Pts',(1.32534250785782,-1.,-1.60677758290954));
#20502=CARTESIAN_POINT('Ctrl Pts',(1.32381550858256,-1.,-1.60073511858687));
#20503=CARTESIAN_POINT('Ctrl Pts',(1.32224985747682,-1.,-1.59471591079403));
#20504=CARTESIAN_POINT('Ctrl Pts',(1.32064537110892,-1.,-1.58872057258245));
#20505=CARTESIAN_POINT('Ctrl Pts',(1.31900135021432,-1.,-1.58274907898834));
#20506=CARTESIAN_POINT('Ctrl Pts',(1.31731642317187,-1.,-1.5768005650559));
#20507=CARTESIAN_POINT('Ctrl Pts',(1.31558903860016,-1.,-1.57087397835723));
#20508=CARTESIAN_POINT('Ctrl Pts',(1.31381795281002,-1.,-1.56496872402353));
#20509=CARTESIAN_POINT('Ctrl Pts',(1.31200264341696,-1.,-1.55908521254821));
#20510=CARTESIAN_POINT('Ctrl Pts',(1.31014393684222,-1.,-1.55322568759481));
#20511=CARTESIAN_POINT('Ctrl Pts',(1.30824393907473,-1.,-1.54739413957185));
#20512=CARTESIAN_POINT('Ctrl Pts',(1.30630475189556,-1.,-1.54159462645432));
#20513=CARTESIAN_POINT('Ctrl Pts',(1.30432735639489,-1.,-1.53582981268977));
#20514=CARTESIAN_POINT('Ctrl Pts',(1.30231064395568,-1.,-1.53009970283891));
#20515=CARTESIAN_POINT('Ctrl Pts',(1.30024984366328,-1.,-1.52439957861062));
#20516=CARTESIAN_POINT('Ctrl Pts',(1.29813791800747,-1.,-1.51872184912724));
#20517=CARTESIAN_POINT('Ctrl Pts',(1.29596850710509,-1.,-1.51305994241402));
#20518=CARTESIAN_POINT('Ctrl Pts',(1.29373841372842,-1.,-1.50741159078365));
#20519=CARTESIAN_POINT('Ctrl Pts',(1.29145022885181,-1.,-1.50178230149776));
#20520=CARTESIAN_POINT('Ctrl Pts',(1.28911506584254,-1.,-1.49618896881754));
#20521=CARTESIAN_POINT('Ctrl Pts',(1.2867467611644,-1.,-1.4906522831278));
#20522=CARTESIAN_POINT('Ctrl Pts',(1.28435533880201,-1.,-1.4851881711891));
#20523=CARTESIAN_POINT('Ctrl Pts',(1.28194158939517,-1.,-1.47980070347096));
#20524=CARTESIAN_POINT('Ctrl Pts',(1.2794891824849,-1.,-1.4744717526707));
#20525=CARTESIAN_POINT('Ctrl Pts',(1.27696414831089,-1.,-1.46916035917133));
#20526=CARTESIAN_POINT('Ctrl Pts',(1.27433119897822,-1.,-1.46382431332476));
#20527=CARTESIAN_POINT('Ctrl Pts',(1.27156805265289,-1.,-1.45843906294697));
#20528=CARTESIAN_POINT('Ctrl Pts',(1.2686778680489,-1.,-1.45301422764247));
#20529=CARTESIAN_POINT('Ctrl Pts',(1.26570925118868,-1.,-1.44761985001662));
#20530=CARTESIAN_POINT('Ctrl Pts',(1.26273903323858,-1.,-1.44236470511303));
#20531=CARTESIAN_POINT('Ctrl Pts',(1.25983531012005,-1.,-1.43734919180848));
#20532=CARTESIAN_POINT('Ctrl Pts',(1.25702687965755,-1.,-1.43262645609691));
#20533=CARTESIAN_POINT('Ctrl Pts',(1.25426945222639,-1.,-1.42815938799387));
#20534=CARTESIAN_POINT('Ctrl Pts',(1.2514145557001,-1.,-1.42378102115575));
#20535=CARTESIAN_POINT('Ctrl Pts',(1.24824430986571,-1.,-1.41923722596025));
#20536=CARTESIAN_POINT('Ctrl Pts',(1.24450600513056,-1.,-1.41422913175179));
#20537=CARTESIAN_POINT('Ctrl Pts',(1.23994455029534,-1.,-1.40845295531283));
#20538=CARTESIAN_POINT('Ctrl Pts',(1.23434087290423,-1.,-1.40164708206106));
#20539=CARTESIAN_POINT('Ctrl Pts',(1.22752961899387,-1.,-1.39361389568796));
#20540=CARTESIAN_POINT('Ctrl Pts',(1.21938737280852,-1.,-1.38420564527715));
#20541=CARTESIAN_POINT('Ctrl Pts',(1.20982812925645,-1.,-1.37331915607905));
#20542=CARTESIAN_POINT('Ctrl Pts',(1.1987959077932,-1.,-1.36088705043885));
#20543=CARTESIAN_POINT('Ctrl Pts',(1.18625865667441,-1.,-1.34687054001093));
#20544=CARTESIAN_POINT('Ctrl Pts',(1.17501305789857,-1.,-1.33437539347008));
#20545=CARTESIAN_POINT('Ctrl Pts',(1.16589330093588,-1.,-1.32428080721772));
#20546=CARTESIAN_POINT('Ctrl Pts',(1.15950888730809,-1.,-1.31722977216397));
#20547=CARTESIAN_POINT('Ctrl Pts',(1.15624053661742,-1.,-1.31362392696032));
#20548=CARTESIAN_POINT('',(1.31362392696032,-1.,-1.15624053661742));
#20549=CARTESIAN_POINT('Origin',(0.,-1.,0.));
#20550=CARTESIAN_POINT('',(1.73811241238545,-1.,-1.34869019493419));
#20551=CARTESIAN_POINT('Ctrl Pts',(1.31362392696032,-1.,-1.15624053661742));
#20552=CARTESIAN_POINT('Ctrl Pts',(1.3172297721596,-1.,-1.15950888730433));
#20553=CARTESIAN_POINT('Ctrl Pts',(1.32428080720544,-1.,-1.16589330092532));
#20554=CARTESIAN_POINT('Ctrl Pts',(1.33437539344842,-1.,-1.17501305787994));
#20555=CARTESIAN_POINT('Ctrl Pts',(1.34687053998157,-1.,-1.18625865664915));
#20556=CARTESIAN_POINT('Ctrl Pts',(1.36088705040677,-1.,-1.1987959077656));
#20557=CARTESIAN_POINT('Ctrl Pts',(1.37331915604962,-1.,-1.20982812923113));
#20558=CARTESIAN_POINT('Ctrl Pts',(1.38420564525391,-1.,-1.21938737278853));
#20559=CARTESIAN_POINT('Ctrl Pts',(1.39361389567257,-1.,-1.22752961898063));
#20560=CARTESIAN_POINT('Ctrl Pts',(1.40164708205345,-1.,-1.23434087289768));
#20561=CARTESIAN_POINT('Ctrl Pts',(1.40845295531151,-1.,-1.23994455029421));
#20562=CARTESIAN_POINT('Ctrl Pts',(1.41422913175437,-1.,-1.24450600513278));
#20563=CARTESIAN_POINT('Ctrl Pts',(1.41923722596421,-1.,-1.24824430986911));
#20564=CARTESIAN_POINT('Ctrl Pts',(1.42378102115911,-1.,-1.25141455570299));
#20565=CARTESIAN_POINT('Ctrl Pts',(1.42815938799555,-1.,-1.25426945222783));
#20566=CARTESIAN_POINT('Ctrl Pts',(1.43262645609679,-1.,-1.25702687965744));
#20567=CARTESIAN_POINT('Ctrl Pts',(1.43734919180719,-1.,-1.25983531011894));
#20568=CARTESIAN_POINT('Ctrl Pts',(1.44236470511145,-1.,-1.26273903323723));
#20569=CARTESIAN_POINT('Ctrl Pts',(1.44761985001544,-1.,-1.26570925118767));
#20570=CARTESIAN_POINT('Ctrl Pts',(1.45301422764205,-1.,-1.26867786804854));
#20571=CARTESIAN_POINT('Ctrl Pts',(1.45843906294725,-1.,-1.27156805265312));
#20572=CARTESIAN_POINT('Ctrl Pts',(1.4638243133254,-1.,-1.27433119897877));
#20573=CARTESIAN_POINT('Ctrl Pts',(1.46916035917197,-1.,-1.27696414831144));
#20574=CARTESIAN_POINT('Ctrl Pts',(1.4744717526711,-1.,-1.27948918248524));
#20575=CARTESIAN_POINT('Ctrl Pts',(1.47980070347102,-1.,-1.28194158939522));
#20576=CARTESIAN_POINT('Ctrl Pts',(1.48518817118891,-1.,-1.28435533880184));
#20577=CARTESIAN_POINT('Ctrl Pts',(1.4906522831275,-1.,-1.28674676116415));
#20578=CARTESIAN_POINT('Ctrl Pts',(1.49618896881729,-1.,-1.28911506584232));
#20579=CARTESIAN_POINT('Ctrl Pts',(1.50178230149764,-1.,-1.29145022885171));
#20580=CARTESIAN_POINT('Ctrl Pts',(1.50741159078367,-1.,-1.29373841372843));
#20581=CARTESIAN_POINT('Ctrl Pts',(1.51305994241412,-1.,-1.29596850710518));
#20582=CARTESIAN_POINT('Ctrl Pts',(1.51872184912735,-1.,-1.29813791800757));
#20583=CARTESIAN_POINT('Ctrl Pts',(1.5243995786107,-1.,-1.30024984366334));
#20584=CARTESIAN_POINT('Ctrl Pts',(1.53009970283893,-1.,-1.3023106439557));
#20585=CARTESIAN_POINT('Ctrl Pts',(1.53582981268976,-1.,-1.30432735639487));
#20586=CARTESIAN_POINT('Ctrl Pts',(1.54159462645428,-1.,-1.30630475189553));
#20587=CARTESIAN_POINT('Ctrl Pts',(1.54739413957183,-1.,-1.30824393907471));
#20588=CARTESIAN_POINT('Ctrl Pts',(1.55322568759481,-1.,-1.31014393684221));
#20589=CARTESIAN_POINT('Ctrl Pts',(1.55908521254822,-1.,-1.31200264341696));
#20590=CARTESIAN_POINT('Ctrl Pts',(1.56496872402352,-1.,-1.31381795281002));
#20591=CARTESIAN_POINT('Ctrl Pts',(1.57087397835721,-1.,-1.31558903860015));
#20592=CARTESIAN_POINT('Ctrl Pts',(1.57680056505585,-1.,-1.31731642317183));
#20593=CARTESIAN_POINT('Ctrl Pts',(1.58274907898829,-1.,-1.31900135021428));
#20594=CARTESIAN_POINT('Ctrl Pts',(1.58872057258244,-1.,-1.32064537110891));
#20595=CARTESIAN_POINT('Ctrl Pts',(1.59471591079408,-1.,-1.32224985747686));
#20596=CARTESIAN_POINT('Ctrl Pts',(1.600735118587,-1.,-1.32381550858266));
#20597=CARTESIAN_POINT('Ctrl Pts',(1.6067775829097,-1.,-1.32534250785794));
#20598=CARTESIAN_POINT('Ctrl Pts',(1.61284234015762,-1.,-1.32683074483365));
#20599=CARTESIAN_POINT('Ctrl Pts',(1.61892832270723,-1.,-1.32828000610448));
#20600=CARTESIAN_POINT('Ctrl Pts',(1.62503464209777,-1.,-1.32969019505665));
#20601=CARTESIAN_POINT('Ctrl Pts',(1.63116079730887,-1.,-1.33106149345618));
#20602=CARTESIAN_POINT('Ctrl Pts',(1.63730653475049,-1.,-1.33239425103694));
#20603=CARTESIAN_POINT('Ctrl Pts',(1.64347174856007,-1.,-1.33368890676554));
#20604=CARTESIAN_POINT('Ctrl Pts',(1.64965637286843,-1.,-1.33494590468003));
#20605=CARTESIAN_POINT('Ctrl Pts',(1.65586025952651,-1.,-1.33616559745217));
#20606=CARTESIAN_POINT('Ctrl Pts',(1.66208312542073,-1.,-1.33734820885331));
#20607=CARTESIAN_POINT('Ctrl Pts',(1.66832460784078,-1.,-1.33849388654458));
#20608=CARTESIAN_POINT('Ctrl Pts',(1.67458429426126,-1.,-1.33960273470372));
#20609=CARTESIAN_POINT('Ctrl Pts',(1.68086176030308,-1.,-1.3406748518516));
#20610=CARTESIAN_POINT('Ctrl Pts',(1.68715660868602,-1.,-1.34171037484673));
#20611=CARTESIAN_POINT('Ctrl Pts',(1.6934684849664,-1.,-1.34270948206139));
#20612=CARTESIAN_POINT('Ctrl Pts',(1.69979707754221,-1.,-1.34367237124322));
#20613=CARTESIAN_POINT('Ctrl Pts',(1.70614212266676,-1.,-1.34459924533783));
#20614=CARTESIAN_POINT('Ctrl Pts',(1.71250340687011,-1.,-1.34549029589563));
#20615=CARTESIAN_POINT('Ctrl Pts',(1.7188807715095,-1.,-1.34634568653586));
#20616=CARTESIAN_POINT('Ctrl Pts',(1.72527410681298,-1.,-1.34716554820013));
#20617=CARTESIAN_POINT('Ctrl Pts',(1.73040149654497,-1.,-1.3477930915247));
#20618=CARTESIAN_POINT('Ctrl Pts',(1.73425417886254,-1.,-1.34824783113158));
#20619=CARTESIAN_POINT('Ctrl Pts',(1.73682580585819,-1.,-1.34854391898145));
#20620=CARTESIAN_POINT('Ctrl Pts',(1.73811241238545,-1.,-1.34869019493419));
#20621=CARTESIAN_POINT('',(1.81978687191668,-1.,-1.23627494547115));
#20622=CARTESIAN_POINT('',(1.73811241238545,-1.,-1.34869019493419));
#20623=CARTESIAN_POINT('',(1.5055822144029,-1.,-0.892032620296855));
#20624=CARTESIAN_POINT('Ctrl Pts',(1.81978687191668,-1.,-1.23627494547115));
#20625=CARTESIAN_POINT('Ctrl Pts',(1.81925017193531,-1.,-1.23509651170384));
#20626=CARTESIAN_POINT('Ctrl Pts',(1.81817389920914,-1.,-1.23274224526804));
#20627=CARTESIAN_POINT('Ctrl Pts',(1.81655087183054,-1.,-1.22921864890975));
#20628=CARTESIAN_POINT('Ctrl Pts',(1.81436959209778,-1.,-1.22453613304507));
#20629=CARTESIAN_POINT('Ctrl Pts',(1.81161420806172,-1.,-1.2187090610323));
#20630=CARTESIAN_POINT('Ctrl Pts',(1.80882996916931,-1.,-1.2129081570818));
#20631=CARTESIAN_POINT('Ctrl Pts',(1.80601678480772,-1.,-1.20713356605519));
#20632=CARTESIAN_POINT('Ctrl Pts',(1.8031745483882,-1.,-1.2013854893912));
#20633=CARTESIAN_POINT('Ctrl Pts',(1.80030314370121,-1.,-1.19566418930405));
#20634=CARTESIAN_POINT('Ctrl Pts',(1.79740245923649,-1.,-1.1899699793456));
#20635=CARTESIAN_POINT('Ctrl Pts',(1.79447240321572,-1.,-1.18430321697471));
#20636=CARTESIAN_POINT('Ctrl Pts',(1.79151291552646,-1.,-1.17866429440781));
#20637=CARTESIAN_POINT('Ctrl Pts',(1.78852398877523,-1.,-1.17305363177265));
#20638=CARTESIAN_POINT('Ctrl Pts',(1.78550566040349,-1.,-1.16747166312239));
#20639=CARTESIAN_POINT('Ctrl Pts',(1.78245795880949,-1.,-1.16191881298458));
#20640=CARTESIAN_POINT('Ctrl Pts',(1.77938085564261,-1.,-1.15639547194689));
#20641=CARTESIAN_POINT('Ctrl Pts',(1.77627422557034,-1.,-1.15090197841531));
#20642=CARTESIAN_POINT('Ctrl Pts',(1.77313777896234,-1.,-1.14543858226948));
#20643=CARTESIAN_POINT('Ctrl Pts',(1.76997111386806,-1.,-1.14000548337));
#20644=CARTESIAN_POINT('Ctrl Pts',(1.76677384551883,-1.,-1.13460291804635));
#20645=CARTESIAN_POINT('Ctrl Pts',(1.76354571966171,-1.,-1.12923123555076));
#20646=CARTESIAN_POINT('Ctrl Pts',(1.76028671825084,-1.,-1.12389096855078));
#20647=CARTESIAN_POINT('Ctrl Pts',(1.75699720772089,-1.,-1.11858293216752));
#20648=CARTESIAN_POINT('Ctrl Pts',(1.75367772094617,-1.,-1.11330807582542));
#20649=CARTESIAN_POINT('Ctrl Pts',(1.75032866075914,-1.,-1.10806728183003));
#20650=CARTESIAN_POINT('Ctrl Pts',(1.74695004214924,-1.,-1.10286118991144));
#20651=CARTESIAN_POINT('Ctrl Pts',(1.74354119236212,-1.,-1.09768999241229));
#20652=CARTESIAN_POINT('Ctrl Pts',(1.74010053962252,-1.,-1.09255329056496));
#20653=CARTESIAN_POINT('Ctrl Pts',(1.73662628326093,-1.,-1.08745056285429));
#20654=CARTESIAN_POINT('Ctrl Pts',(1.73311705663407,-1.,-1.08238162784749));
#20655=CARTESIAN_POINT('Ctrl Pts',(1.72957248977424,-1.,-1.0773470373727));
#20656=CARTESIAN_POINT('Ctrl Pts',(1.72599406198489,-1.,-1.07234866990252));
#20657=CARTESIAN_POINT('Ctrl Pts',(1.72238500928456,-1.,-1.06738966975463));
#20658=CARTESIAN_POINT('Ctrl Pts',(1.71874858456908,-1.,-1.0624732468065));
#20659=CARTESIAN_POINT('Ctrl Pts',(1.71508654427022,-1.,-1.05760163192481));
#20660=CARTESIAN_POINT('Ctrl Pts',(1.71139783543986,-1.,-1.05277517202854));
#20661=CARTESIAN_POINT('Ctrl Pts',(1.70767646263641,-1.,-1.0479908540499));
#20662=CARTESIAN_POINT('Ctrl Pts',(1.70391338707969,-1.,-1.04324363334546));
#20663=CARTESIAN_POINT('Ctrl Pts',(1.70010052930951,-1.,-1.03852922490782));
#20664=CARTESIAN_POINT('Ctrl Pts',(1.69623414782769,-1.,-1.03384646003587));
#20665=CARTESIAN_POINT('Ctrl Pts',(1.69231840863471,-1.,-1.02919977579155));
#20666=CARTESIAN_POINT('Ctrl Pts',(1.68836910178475,-1.,-1.02460180535272));
#20667=CARTESIAN_POINT('Ctrl Pts',(1.68440578021739,-1.,-1.02006795074222));
#20668=CARTESIAN_POINT('Ctrl Pts',(1.6804428989482,-1.,-1.01561026162787));
#20669=CARTESIAN_POINT('Ctrl Pts',(1.67648246776457,-1.,-1.01123236493507));
#20670=CARTESIAN_POINT('Ctrl Pts',(1.67250335383248,-1.,-1.00692206696387));
#20671=CARTESIAN_POINT('Ctrl Pts',(1.66846059277231,-1.,-1.00265091003682));
#20672=CARTESIAN_POINT('Ctrl Pts',(1.66430758030304,-1.,-0.998389654952317));
#20673=CARTESIAN_POINT('Ctrl Pts',(1.66001553809916,-1.,-0.994121836661116));
#20674=CARTESIAN_POINT('Ctrl Pts',(1.65559044289746,-1.,-0.98985562785445));
#20675=CARTESIAN_POINT('Ctrl Pts',(1.6511001661277,-1.,-0.985642622921626));
#20676=CARTESIAN_POINT('Ctrl Pts',(1.64665139190834,-1.,-0.981562530940574));
#20677=CARTESIAN_POINT('Ctrl Pts',(1.64233990826831,-1.,-0.977689794120297));
#20678=CARTESIAN_POINT('Ctrl Pts',(1.63820952658157,-1.,-0.974066058287501));
#20679=CARTESIAN_POINT('Ctrl Pts',(1.63420665729609,-1.,-0.970669715996356));
#20680=CARTESIAN_POINT('Ctrl Pts',(1.63013849959083,-1.,-0.967387853228041));
#20681=CARTESIAN_POINT('Ctrl Pts',(1.6257193066974,-1.,-0.964046107037821));
#20682=CARTESIAN_POINT('Ctrl Pts',(1.62061638139929,-1.,-0.960438326099958));
#20683=CARTESIAN_POINT('Ctrl Pts',(1.61449324337233,-1.,-0.956354422921573));
#20684=CARTESIAN_POINT('Ctrl Pts',(1.60706069897794,-1.,-0.951613284361248));
#20685=CARTESIAN_POINT('Ctrl Pts',(1.59810042045408,-1.,-0.946078063325796));
#20686=CARTESIAN_POINT('Ctrl Pts',(1.58744937489796,-1.,-0.939646377909319));
#20687=CARTESIAN_POINT('Ctrl Pts',(1.57499388385561,-1.,-0.932246680128849));
#20688=CARTESIAN_POINT('Ctrl Pts',(1.56065988582509,-1.,-0.923832188966322));
#20689=CARTESIAN_POINT('Ctrl Pts',(1.54440491152807,-1.,-0.91437591904658));
#20690=CARTESIAN_POINT('Ctrl Pts',(1.52984849890434,-1.,-0.905967409640499));
#20691=CARTESIAN_POINT('Ctrl Pts',(1.51805569591479,-1.,-0.89918504749193));
#20692=CARTESIAN_POINT('Ctrl Pts',(1.50980486807181,-1.,-0.894452006967538));
#20693=CARTESIAN_POINT('Ctrl Pts',(1.5055822144029,-1.,-0.892032620296855));
#20694=CARTESIAN_POINT('',(1.60662857109684,-1.,-0.693717979106306));
#20695=CARTESIAN_POINT('Origin',(0.,-1.,0.));
#20696=CARTESIAN_POINT('',(2.0698113262342,-1.,-0.745574324794401));
#20697=CARTESIAN_POINT('Ctrl Pts',(1.60662857109684,-1.,-0.693717979106306));
#20698=CARTESIAN_POINT('Ctrl Pts',(1.61106790957619,-1.,-0.69571209787897));
#20699=CARTESIAN_POINT('Ctrl Pts',(1.61974673471117,-1.,-0.699605146398837));
#20700=CARTESIAN_POINT('Ctrl Pts',(1.6321654166204,-1.,-0.705159151977294));
#20701=CARTESIAN_POINT('Ctrl Pts',(1.64752408828442,-1.,-0.711993139340448));
#20702=CARTESIAN_POINT('Ctrl Pts',(1.66472880551777,-1.,-0.71958543378795));
#20703=CARTESIAN_POINT('Ctrl Pts',(1.67996158451922,-1.,-0.726235967982445));
#20704=CARTESIAN_POINT('Ctrl Pts',(1.69326921972915,-1.,-0.731963238685357));
#20705=CARTESIAN_POINT('Ctrl Pts',(1.70473309004249,-1.,-0.736799665716932));
#20706=CARTESIAN_POINT('Ctrl Pts',(1.71447789751001,-1.,-0.74079516202821));
#20707=CARTESIAN_POINT('Ctrl Pts',(1.72268229916769,-1.,-0.744021445433094));
#20708=CARTESIAN_POINT('Ctrl Pts',(1.72958533647714,-1.,-0.746574710097752));
#20709=CARTESIAN_POINT('Ctrl Pts',(1.7355035168033,-1.,-0.74858246295687));
#20710=CARTESIAN_POINT('Ctrl Pts',(1.74080458267114,-1.,-0.75019343598125));
#20711=CARTESIAN_POINT('Ctrl Pts',(1.74585086852502,-1.,-0.751555614164483));
#20712=CARTESIAN_POINT('Ctrl Pts',(1.75095139468794,-1.,-0.752797683531314));
#20713=CARTESIAN_POINT('Ctrl Pts',(1.75631083600019,-1.,-0.754009254027829));
#20714=CARTESIAN_POINT('Ctrl Pts',(1.76197817240128,-1.,-0.755220979974462));
#20715=CARTESIAN_POINT('Ctrl Pts',(1.76789396002998,-1.,-0.75642189602781));
#20716=CARTESIAN_POINT('Ctrl Pts',(1.77394167108292,-1.,-0.757578264077029));
#20717=CARTESIAN_POINT('Ctrl Pts',(1.77999411220945,-1.,-0.758650626677519));
#20718=CARTESIAN_POINT('Ctrl Pts',(1.78596964884604,-1.,-0.75961440111019));
#20719=CARTESIAN_POINT('Ctrl Pts',(1.7918581561088,-1.,-0.760469555880749));
#20720=CARTESIAN_POINT('Ctrl Pts',(1.79768986997783,-1.,-0.761229695230558));
#20721=CARTESIAN_POINT('Ctrl Pts',(1.80351583877342,-1.,-0.761915336443547));
#20722=CARTESIAN_POINT('Ctrl Pts',(1.80938551463965,-1.,-0.762546129463938));
#20723=CARTESIAN_POINT('Ctrl Pts',(1.8153211840553,-1.,-0.763132003836634));
#20724=CARTESIAN_POINT('Ctrl Pts',(1.82131873145266,-1.,-0.763673465462727));
#20725=CARTESIAN_POINT('Ctrl Pts',(1.82735991200065,-1.,-0.764165902605995));
#20726=CARTESIAN_POINT('Ctrl Pts',(1.83342077227142,-1.,-0.764602549687853));
#20727=CARTESIAN_POINT('Ctrl Pts',(1.83948181064835,-1.,-0.764978057881738));
#20728=CARTESIAN_POINT('Ctrl Pts',(1.84553698875924,-1.,-0.765291664862029));
#20729=CARTESIAN_POINT('Ctrl Pts',(1.85158945130063,-1.,-0.765545710619063));
#20730=CARTESIAN_POINT('Ctrl Pts',(1.85764741390394,-1.,-0.765744212909319));
#20731=CARTESIAN_POINT('Ctrl Pts',(1.86372027063312,-1.,-0.765891519092547));
#20732=CARTESIAN_POINT('Ctrl Pts',(1.86981398314341,-1.,-0.765990708546091));
#20733=CARTESIAN_POINT('Ctrl Pts',(1.87592888967883,-1.,-0.766042837036744));
#20734=CARTESIAN_POINT('Ctrl Pts',(1.88206215302561,-1.,-0.766047794851865));
#20735=CARTESIAN_POINT('Ctrl Pts',(1.88820926433409,-1.,-0.766004837062091));
#20736=CARTESIAN_POINT('Ctrl Pts',(1.89436577771388,-1.,-0.765913193856978));
#20737=CARTESIAN_POINT('Ctrl Pts',(1.90052930393596,-1.,-0.765772772593386));
#20738=CARTESIAN_POINT('Ctrl Pts',(1.90669961402356,-1.,-0.765584196937919));
#20739=CARTESIAN_POINT('Ctrl Pts',(1.91287765805169,-1.,-0.765348465884722));
#20740=CARTESIAN_POINT('Ctrl Pts',(1.91906491634196,-1.,-0.765066729667089));
#20741=CARTESIAN_POINT('Ctrl Pts',(1.92526263537048,-1.,-0.764740025488212));
#20742=CARTESIAN_POINT('Ctrl Pts',(1.93147105496382,-1.,-0.764369010673941));
#20743=CARTESIAN_POINT('Ctrl Pts',(1.93768964875886,-1.,-0.763954049121459));
#20744=CARTESIAN_POINT('Ctrl Pts',(1.9439174661764,-1.,-0.763495333538629));
#20745=CARTESIAN_POINT('Ctrl Pts',(1.95015342590024,-1.,-0.762992990878769));
#20746=CARTESIAN_POINT('Ctrl Pts',(1.95639665309869,-1.,-0.762447203806179));
#20747=CARTESIAN_POINT('Ctrl Pts',(1.96264672744186,-1.,-0.761858300014424));
#20748=CARTESIAN_POINT('Ctrl Pts',(1.96890351582499,-1.,-0.761226690483821));
#20749=CARTESIAN_POINT('Ctrl Pts',(1.97516705321494,-1.,-0.760552825409757));
#20750=CARTESIAN_POINT('Ctrl Pts',(1.98143741418172,-1.,-0.75983714745219));
#20751=CARTESIAN_POINT('Ctrl Pts',(1.98771456680874,-1.,-0.759080037802488));
#20752=CARTESIAN_POINT('Ctrl Pts',(1.99399831098817,-1.,-0.758281796766761));
#20753=CARTESIAN_POINT('Ctrl Pts',(2.00028834739178,-1.,-0.757442676862724));
#20754=CARTESIAN_POINT('Ctrl Pts',(2.0065843158773,-1.,-0.756562904646671));
#20755=CARTESIAN_POINT('Ctrl Pts',(2.01288584328084,-1.,-0.755642704957865));
#20756=CARTESIAN_POINT('Ctrl Pts',(2.01919259405809,-1.,-0.754682330722816));
#20757=CARTESIAN_POINT('Ctrl Pts',(2.02550428623313,-1.,-0.753682061112768));
#20758=CARTESIAN_POINT('Ctrl Pts',(2.03182068456221,-1.,-0.752642180487211));
#20759=CARTESIAN_POINT('Ctrl Pts',(2.03814160092099,-1.,-0.751562963361115));
#20760=CARTESIAN_POINT('Ctrl Pts',(2.04446689147979,-1.,-0.750444657875576));
#20761=CARTESIAN_POINT('Ctrl Pts',(2.05079645592154,-1.,-0.749287468665046));
#20762=CARTESIAN_POINT('Ctrl Pts',(2.05713023031006,-1.,-0.748091554183803));
#20763=CARTESIAN_POINT('Ctrl Pts',(2.06220058927826,-1.,-0.74710393278792));
#20764=CARTESIAN_POINT('Ctrl Pts',(2.06600523016815,-1.,-0.746345871544201));
#20765=CARTESIAN_POINT('Ctrl Pts',(2.06854248895728,-1.,-0.745832791378367));
#20766=CARTESIAN_POINT('Ctrl Pts',(2.0698113262342,-1.,-0.745574324794401));
#20767=CARTESIAN_POINT('',(2.11275013067528,-1.,-0.61342227326009));
#20768=CARTESIAN_POINT('',(2.0698113262342,-1.,-0.745574324794401));
#20769=CARTESIAN_POINT('',(1.7075470150345,-1.,-0.383122945602004));
#20770=CARTESIAN_POINT('Ctrl Pts',(2.11275013067528,-1.,-0.61342227326009));
#20771=CARTESIAN_POINT('Ctrl Pts',(2.11187554259986,-1.,-0.6124673655618));
#20772=CARTESIAN_POINT('Ctrl Pts',(2.11012443807238,-1.,-0.610560911689899));
#20773=CARTESIAN_POINT('Ctrl Pts',(2.1074919961518,-1.,-0.607711315454876));
#20774=CARTESIAN_POINT('Ctrl Pts',(2.10397049886949,-1.,-0.60393203073603));
#20775=CARTESIAN_POINT('Ctrl Pts',(2.0995493086477,-1.,-0.599241616420534));
#20776=CARTESIAN_POINT('Ctrl Pts',(2.0951087622027,-1.,-0.594585006052162));
#20777=CARTESIAN_POINT('Ctrl Pts',(2.09064881812129,-1.,-0.589962365403406));
#20778=CARTESIAN_POINT('Ctrl Pts',(2.08616943727951,-1.,-0.585373918991617));
#20779=CARTESIAN_POINT('Ctrl Pts',(2.08167059018418,-1.,-0.580819952108064));
#20780=CARTESIAN_POINT('Ctrl Pts',(2.07715226767559,-1.,-0.576300797416845));
#20781=CARTESIAN_POINT('Ctrl Pts',(2.07261449292824,-1.,-0.571816823242603));
#20782=CARTESIAN_POINT('Ctrl Pts',(2.06805732997334,-1.,-0.567368421181087));
#20783=CARTESIAN_POINT('Ctrl Pts',(2.06348090160589,-1.,-0.562955993082262));
#20784=CARTESIAN_POINT('Ctrl Pts',(2.05888537756462,-1.,-0.558579940185152));
#20785=CARTESIAN_POINT('Ctrl Pts',(2.05427091604413,-1.,-0.554240657463906));
#20786=CARTESIAN_POINT('Ctrl Pts',(2.04963761077958,-1.,-0.549938525150295));
#20787=CARTESIAN_POINT('Ctrl Pts',(2.04498544714588,-1.,-0.54567390381743));
#20788=CARTESIAN_POINT('Ctrl Pts',(2.04031422690527,-1.,-0.541447120615659));
#20789=CARTESIAN_POINT('Ctrl Pts',(2.03562362954037,-1.,-0.537258489833262));
#20790=CARTESIAN_POINT('Ctrl Pts',(2.03091336214426,-1.,-0.533108355132977));
#20791=CARTESIAN_POINT('Ctrl Pts',(2.0261832908329,-1.,-0.528997127241914));
#20792=CARTESIAN_POINT('Ctrl Pts',(2.02143356304698,-1.,-0.524925318333476));
#20793=CARTESIAN_POINT('Ctrl Pts',(2.01666477917286,-1.,-0.520893590399371));
#20794=CARTESIAN_POINT('Ctrl Pts',(2.01187773939242,-1.,-0.516902681728687));
#20795=CARTESIAN_POINT('Ctrl Pts',(2.00707309946949,-1.,-0.512953306961793));
#20796=CARTESIAN_POINT('Ctrl Pts',(2.00225107134734,-1.,-0.509046069886157));
#20797=CARTESIAN_POINT('Ctrl Pts',(1.99741107463572,-1.,-0.505181361323026));
#20798=CARTESIAN_POINT('Ctrl Pts',(1.99255149126155,-1.,-0.501359287727146));
#20799=CARTESIAN_POINT('Ctrl Pts',(1.98767044752932,-1.,-0.497579909545574));
#20800=CARTESIAN_POINT('Ctrl Pts',(1.98276658761821,-1.,-0.493843476541495));
#20801=CARTESIAN_POINT('Ctrl Pts',(1.97783973019229,-1.,-0.490150627860953));
#20802=CARTESIAN_POINT('Ctrl Pts',(1.97289186263272,-1.,-0.486502692907659));
#20803=CARTESIAN_POINT('Ctrl Pts',(1.96792703422362,-1.,-0.482901662120691));
#20804=CARTESIAN_POINT('Ctrl Pts',(1.96294933055943,-1.,-0.479349583074855));
#20805=CARTESIAN_POINT('Ctrl Pts',(1.95796111148177,-1.,-0.475848034683176));
#20806=CARTESIAN_POINT('Ctrl Pts',(1.95296148278133,-1.,-0.472397672264072));
#20807=CARTESIAN_POINT('Ctrl Pts',(1.94794381136514,-1.,-0.468997482913135));
#20808=CARTESIAN_POINT('Ctrl Pts',(1.9428979419619,-1.,-0.46564546202603));
#20809=CARTESIAN_POINT('Ctrl Pts',(1.93781486640821,-1.,-0.462340031009057));
#20810=CARTESIAN_POINT('Ctrl Pts',(1.93269066517934,-1.,-0.459081234547926));
#20811=CARTESIAN_POINT('Ctrl Pts',(1.92753067150476,-1.,-0.455872005174371));
#20812=CARTESIAN_POINT('Ctrl Pts',(1.92235380648502,-1.,-0.452719478359433));
#20813=CARTESIAN_POINT('Ctrl Pts',(1.91718342555755,-1.,-0.449632260106662));
#20814=CARTESIAN_POINT('Ctrl Pts',(1.9120369998112,-1.,-0.446617343485711));
#20815=CARTESIAN_POINT('Ctrl Pts',(1.90691756144898,-1.,-0.443677556849151));
#20816=CARTESIAN_POINT('Ctrl Pts',(1.90180124389086,-1.,-0.440807833704038));
#20817=CARTESIAN_POINT('Ctrl Pts',(1.89663648956466,-1.,-0.437995003948244));
#20818=CARTESIAN_POINT('Ctrl Pts',(1.89136993975504,-1.,-0.435225660963383));
#20819=CARTESIAN_POINT('Ctrl Pts',(1.88596913666793,-1.,-0.432493038548748));
#20820=CARTESIAN_POINT('Ctrl Pts',(1.88044229001832,-1.,-0.429803062482345));
#20821=CARTESIAN_POINT('Ctrl Pts',(1.87486989291484,-1.,-0.427183828519102));
#20822=CARTESIAN_POINT('Ctrl Pts',(1.86937803944323,-1.,-0.424678177291359));
#20823=CARTESIAN_POINT('Ctrl Pts',(1.86408083334028,-1.,-0.422327307418275));
#20824=CARTESIAN_POINT('Ctrl Pts',(1.85903281096686,-1.,-0.42015728797562));
#20825=CARTESIAN_POINT('Ctrl Pts',(1.85417632856234,-1.,-0.418164129143534));
#20826=CARTESIAN_POINT('Ctrl Pts',(1.84929312929882,-1.,-0.416300022038864));
#20827=CARTESIAN_POINT('Ctrl Pts',(1.8440575707371,-1.,-0.41448743825434));
#20828=CARTESIAN_POINT('Ctrl Pts',(1.83808953475839,-1.,-0.412633125322162));
#20829=CARTESIAN_POINT('Ctrl Pts',(1.83100408895216,-1.,-0.410641256301675));
#20830=CARTESIAN_POINT('Ctrl Pts',(1.8224702267854,-1.,-0.408428948108534));
#20831=CARTESIAN_POINT('Ctrl Pts',(1.81223801813988,-1.,-0.405933518411838));
#20832=CARTESIAN_POINT('Ctrl Pts',(1.80012077176221,-1.,-0.403107976170441));
#20833=CARTESIAN_POINT('Ctrl Pts',(1.78598826347533,-1.,-0.399919403783081));
#20834=CARTESIAN_POINT('Ctrl Pts',(1.7697556004756,-1.,-0.39634619612042));
#20835=CARTESIAN_POINT('Ctrl Pts',(1.75137405313962,-1.,-0.392375812294307));
#20836=CARTESIAN_POINT('Ctrl Pts',(1.7349317097561,-1.,-0.388877023509192));
#20837=CARTESIAN_POINT('Ctrl Pts',(1.72162022246158,-1.,-0.38607079032701));
#20838=CARTESIAN_POINT('Ctrl Pts',(1.71231062891958,-1.,-0.384119047315542));
#20839=CARTESIAN_POINT('Ctrl Pts',(1.7075470150345,-1.,-0.383122945602004));
#20840=CARTESIAN_POINT('',(1.74236521665491,-1.,-0.163289472382896));
#20841=CARTESIAN_POINT('Origin',(0.,-1.,0.));
#20842=CARTESIAN_POINT('',(2.19890268624765,-1.,-0.0694764450219582));
#20843=CARTESIAN_POINT('Ctrl Pts',(1.74236521665491,-1.,-0.163289472382896));
#20844=CARTESIAN_POINT('Ctrl Pts',(1.7472034950333,-1.,-0.163814161002002));
#20845=CARTESIAN_POINT('Ctrl Pts',(1.75666056638427,-1.,-0.164834765707159));
#20846=CARTESIAN_POINT('Ctrl Pts',(1.77018771684844,-1.,-0.1662793551464));
#20847=CARTESIAN_POINT('Ctrl Pts',(1.7869064998507,-1.,-0.168032772805197));
#20848=CARTESIAN_POINT('Ctrl Pts',(1.80561530629706,-1.,-0.169936923904608));
#20849=CARTESIAN_POINT('Ctrl Pts',(1.82215766811545,-1.,-0.171554770204119));
#20850=CARTESIAN_POINT('Ctrl Pts',(1.83658380527692,-1.,-0.1728894428919));
#20851=CARTESIAN_POINT('Ctrl Pts',(1.8489811319852,-1.,-0.173946627587732));
#20852=CARTESIAN_POINT('Ctrl Pts',(1.85948367088837,-1.,-0.17473525927603));
#20853=CARTESIAN_POINT('Ctrl Pts',(1.86828349694799,-1.,-0.175268337590758));
#20854=CARTESIAN_POINT('Ctrl Pts',(1.87563767773588,-1.,-0.175563480746485));
#20855=CARTESIAN_POINT('Ctrl Pts',(1.88188663145367,-1.,-0.175644148889699));
#20856=CARTESIAN_POINT('Ctrl Pts',(1.88742606273259,-1.,-0.175538155840648));
#20857=CARTESIAN_POINT('Ctrl Pts',(1.892646301985,-1.,-0.175274276190844));
#20858=CARTESIAN_POINT('Ctrl Pts',(1.89788101117132,-1.,-0.174879405091263));
#20859=CARTESIAN_POINT('Ctrl Pts',(1.90335253862834,-1.,-0.174375518661085));
#20860=CARTESIAN_POINT('Ctrl Pts',(1.90911693975267,-1.,-0.173776635257817));
#20861=CARTESIAN_POINT('Ctrl Pts',(1.91511429159527,-1.,-0.173090695383496));
#20862=CARTESIAN_POINT('Ctrl Pts',(1.9212233439798,-1.,-0.172321621259514));
#20863=CARTESIAN_POINT('Ctrl Pts',(1.92731093582036,-1.,-0.171471191532988));
#20864=CARTESIAN_POINT('Ctrl Pts',(1.93329183155539,-1.,-0.170541253116202));
#20865=CARTESIAN_POINT('Ctrl Pts',(1.93915639211581,-1.,-0.169534904817491));
#20866=CARTESIAN_POINT('Ctrl Pts',(1.94493757756931,-1.,-0.168455741607556));
#20867=CARTESIAN_POINT('Ctrl Pts',(1.95069027794294,-1.,-0.167307501784476));
#20868=CARTESIAN_POINT('Ctrl Pts',(1.9564675971873,-1.,-0.166093592002813));
#20869=CARTESIAN_POINT('Ctrl Pts',(1.96229379940136,-1.,-0.164816568920269));
#20870=CARTESIAN_POINT('Ctrl Pts',(1.96816512677967,-1.,-0.163478185457734));
#20871=CARTESIAN_POINT('Ctrl Pts',(1.97406280235188,-1.,-0.162079693556289));
#20872=CARTESIAN_POINT('Ctrl Pts',(1.97996195437559,-1.,-0.160622060784611));
#20873=CARTESIAN_POINT('Ctrl Pts',(1.98584238283292,-1.,-0.159106226437299));
#20874=CARTESIAN_POINT('Ctrl Pts',(1.99169810931908,-1.,-0.157533331459227));
#20875=CARTESIAN_POINT('Ctrl Pts',(1.99753284771497,-1.,-0.155904629548784));
#20876=CARTESIAN_POINT('Ctrl Pts',(2.00335565310543,-1.,-0.154221403049722));
#20877=CARTESIAN_POINT('Ctrl Pts',(2.00917680318424,-1.,-0.15248488362145));
#20878=CARTESIAN_POINT('Ctrl Pts',(2.01500291940238,-1.,-0.150696157673078));
#20879=CARTESIAN_POINT('Ctrl Pts',(2.02083464969894,-1.,-0.148856124775337));
#20880=CARTESIAN_POINT('Ctrl Pts',(2.02666926182017,-1.,-0.146965557332583));
#20881=CARTESIAN_POINT('Ctrl Pts',(2.03250223739942,-1.,-0.145025140186058));
#20882=CARTESIAN_POINT('Ctrl Pts',(2.03832911025912,-1.,-0.143035515058209));
#20883=CARTESIAN_POINT('Ctrl Pts',(2.04414757947916,-1.,-0.140997332152546));
#20884=CARTESIAN_POINT('Ctrl Pts',(2.04995762001328,-1.,-0.138911255368966));
#20885=CARTESIAN_POINT('Ctrl Pts',(2.05576044414264,-1.,-0.136777941218044));
#20886=CARTESIAN_POINT('Ctrl Pts',(2.06155781517842,-1.,-0.134598026192106));
#20887=CARTESIAN_POINT('Ctrl Pts',(2.06735123910326,-1.,-0.132372111547711));
#20888=CARTESIAN_POINT('Ctrl Pts',(2.07314114713063,-1.,-0.130100748328404));
#20889=CARTESIAN_POINT('Ctrl Pts',(2.07892715110987,-1.,-0.12778444527612));
#20890=CARTESIAN_POINT('Ctrl Pts',(2.08470840653643,-1.,-0.125423679412062));
#20891=CARTESIAN_POINT('Ctrl Pts',(2.09048392424825,-1.,-0.123018905621083));
#20892=CARTESIAN_POINT('Ctrl Pts',(2.0962529286773,-1.,-0.120570567965122));
#20893=CARTESIAN_POINT('Ctrl Pts',(2.102015121329,-1.,-0.118079107988356));
#20894=CARTESIAN_POINT('Ctrl Pts',(2.10777050261309,-1.,-0.115544957687927));
#20895=CARTESIAN_POINT('Ctrl Pts',(2.11351924490306,-1.,-0.112968534419737));
#20896=CARTESIAN_POINT('Ctrl Pts',(2.11926155590865,-1.,-0.110350236135025));
#20897=CARTESIAN_POINT('Ctrl Pts',(2.12499752307,-1.,-0.10769043523109));
#20898=CARTESIAN_POINT('Ctrl Pts',(2.13072704887293,-1.,-0.10498947915274));
#20899=CARTESIAN_POINT('Ctrl Pts',(2.13644992667165,-1.,-0.102247700556101));
#20900=CARTESIAN_POINT('Ctrl Pts',(2.14216588396025,-1.,-0.0994654261990917));
#20901=CARTESIAN_POINT('Ctrl Pts',(2.14787463531795,-1.,-0.096642985230546));
#20902=CARTESIAN_POINT('Ctrl Pts',(2.1535759397817,-1.,-0.0937807218867645));
#20903=CARTESIAN_POINT('Ctrl Pts',(2.15926961544516,-1.,-0.0908789888107267));
#20904=CARTESIAN_POINT('Ctrl Pts',(2.16495552645014,-1.,-0.0879381291386924));
#20905=CARTESIAN_POINT('Ctrl Pts',(2.17063357870952,-1.,-0.0849584620835374));
#20906=CARTESIAN_POINT('Ctrl Pts',(2.176303712113,-1.,-0.0819402680872767));
#20907=CARTESIAN_POINT('Ctrl Pts',(2.18196589448887,-1.,-0.0788837727685244));
#20908=CARTESIAN_POINT('Ctrl Pts',(2.1876201139953,-1.,-0.0757891465836149));
#20909=CARTESIAN_POINT('Ctrl Pts',(2.19213712013662,-1.,-0.0732830357306726));
#20910=CARTESIAN_POINT('Ctrl Pts',(2.19552129484002,-1.,-0.0713863779526155));
#20911=CARTESIAN_POINT('Ctrl Pts',(2.19777582085423,-1.,-0.0701143536325491));
#20912=CARTESIAN_POINT('Ctrl Pts',(2.19890268624765,-1.,-0.0694764450219582));
#20913=CARTESIAN_POINT('',(2.19890268624765,-1.,0.0694764450219582));
#20914=CARTESIAN_POINT('',(2.19890268624765,-1.,-0.0694764450219582));
#20915=CARTESIAN_POINT('',(1.74236521665491,-1.,0.163289472382896));
#20916=CARTESIAN_POINT('Ctrl Pts',(2.19890268624765,-1.,0.0694764450219582));
#20917=CARTESIAN_POINT('Ctrl Pts',(2.19777582085261,-1.,0.0701143536324925));
#20918=CARTESIAN_POINT('Ctrl Pts',(2.19552129483562,-1.,0.0713863779524626));
#20919=CARTESIAN_POINT('Ctrl Pts',(2.19213712012956,-1.,0.0732830357304275));
#20920=CARTESIAN_POINT('Ctrl Pts',(2.1876201139874,-1.,0.075789146583341));
#20921=CARTESIAN_POINT('Ctrl Pts',(2.18196589448304,-1.,0.0788837727683226));
#20922=CARTESIAN_POINT('Ctrl Pts',(2.1763037121106,-1.,0.0819402680871938));
#20923=CARTESIAN_POINT('Ctrl Pts',(2.17063357871031,-1.,0.0849584620835642));
#20924=CARTESIAN_POINT('Ctrl Pts',(2.16495552645275,-1.,0.0879381291387821));
#20925=CARTESIAN_POINT('Ctrl Pts',(2.15926961544808,-1.,0.0908789888108265));
#20926=CARTESIAN_POINT('Ctrl Pts',(2.15357593978377,-1.,0.0937807218868344));
#20927=CARTESIAN_POINT('Ctrl Pts',(2.14787463531864,-1.,0.0966429852305688));
#20928=CARTESIAN_POINT('Ctrl Pts',(2.14216588395974,-1.,0.0994654261990741));
#20929=CARTESIAN_POINT('Ctrl Pts',(2.13644992667052,-1.,0.102247700556063));
#20930=CARTESIAN_POINT('Ctrl Pts',(2.1307270488718,-1.,0.104989479152703));
#20931=CARTESIAN_POINT('Ctrl Pts',(2.12499752306927,-1.,0.107690435231068));
#20932=CARTESIAN_POINT('Ctrl Pts',(2.11926155590849,-1.,0.11035023613502));
#20933=CARTESIAN_POINT('Ctrl Pts',(2.11351924490335,-1.,0.112968534419746));
#20934=CARTESIAN_POINT('Ctrl Pts',(2.10777050261359,-1.,0.11554495768794));
#20935=CARTESIAN_POINT('Ctrl Pts',(2.10201512132945,-1.,0.118079107988368));
#20936=CARTESIAN_POINT('Ctrl Pts',(2.09625292867756,-1.,0.120570567965129));
#20937=CARTESIAN_POINT('Ctrl Pts',(2.09048392424826,-1.,0.123018905621083));
#20938=CARTESIAN_POINT('Ctrl Pts',(2.08470840653628,-1.,0.125423679412058));
#20939=CARTESIAN_POINT('Ctrl Pts',(2.07892715110967,-1.,0.127784445276116));
#20940=CARTESIAN_POINT('Ctrl Pts',(2.07314114713047,-1.,0.1301007483284));
#20941=CARTESIAN_POINT('Ctrl Pts',(2.06735123910319,-1.,0.132372111547709));
#20942=CARTESIAN_POINT('Ctrl Pts',(2.06155781517844,-1.,0.134598026192107));
#20943=CARTESIAN_POINT('Ctrl Pts',(2.0557604441427,-1.,0.136777941218044));
#20944=CARTESIAN_POINT('Ctrl Pts',(2.04995762001333,-1.,0.138911255368966));
#20945=CARTESIAN_POINT('Ctrl Pts',(2.04414757947919,-1.,0.140997332152545));
#20946=CARTESIAN_POINT('Ctrl Pts',(2.03832911025913,-1.,0.143035515058208));
#20947=CARTESIAN_POINT('Ctrl Pts',(2.03250223739941,-1.,0.145025140186058));
#20948=CARTESIAN_POINT('Ctrl Pts',(2.02666926182017,-1.,0.146965557332586));
#20949=CARTESIAN_POINT('Ctrl Pts',(2.02083464969897,-1.,0.148856124775342));
#20950=CARTESIAN_POINT('Ctrl Pts',(2.01500291940243,-1.,0.150696157673084));
#20951=CARTESIAN_POINT('Ctrl Pts',(2.00917680318426,-1.,0.152484883621452));
#20952=CARTESIAN_POINT('Ctrl Pts',(2.00335565310539,-1.,0.154221403049719));
#20953=CARTESIAN_POINT('Ctrl Pts',(1.99753284771487,-1.,0.155904629548774));
#20954=CARTESIAN_POINT('Ctrl Pts',(1.99169810931893,-1.,0.157533331459215));
#20955=CARTESIAN_POINT('Ctrl Pts',(1.98584238283279,-1.,0.159106226437288));
#20956=CARTESIAN_POINT('Ctrl Pts',(1.97996195437557,-1.,0.16062206078461));
#20957=CARTESIAN_POINT('Ctrl Pts',(1.97406280235204,-1.,0.162079693556302));
#20958=CARTESIAN_POINT('Ctrl Pts',(1.96816512678,-1.,0.16347818545776));
#20959=CARTESIAN_POINT('Ctrl Pts',(1.96229379940174,-1.,0.1648165689203));
#20960=CARTESIAN_POINT('Ctrl Pts',(1.95646759718755,-1.,0.166093592002832));
#20961=CARTESIAN_POINT('Ctrl Pts',(1.95069027794286,-1.,0.167307501784469));
#20962=CARTESIAN_POINT('Ctrl Pts',(1.94493757756879,-1.,0.168455741607515));
#20963=CARTESIAN_POINT('Ctrl Pts',(1.93915639211497,-1.,0.169534904817425));
#20964=CARTESIAN_POINT('Ctrl Pts',(1.93329183155455,-1.,0.170541253116136));
#20965=CARTESIAN_POINT('Ctrl Pts',(1.92731093582,-1.,0.17147119153296));
#20966=CARTESIAN_POINT('Ctrl Pts',(1.92122334398034,-1.,0.172321621259556));
#20967=CARTESIAN_POINT('Ctrl Pts',(1.91511429159681,-1.,0.173090695383619));
#20968=CARTESIAN_POINT('Ctrl Pts',(1.90911693975475,-1.,0.173776635257983));
#20969=CARTESIAN_POINT('Ctrl Pts',(1.90335253863003,-1.,0.174375518661222));
#20970=CARTESIAN_POINT('Ctrl Pts',(1.89788101117148,-1.,0.174879405091277));
#20971=CARTESIAN_POINT('Ctrl Pts',(1.89264630198279,-1.,0.175274276190664));
#20972=CARTESIAN_POINT('Ctrl Pts',(1.88742606272818,-1.,0.175538155840286));
#20973=CARTESIAN_POINT('Ctrl Pts',(1.88188663144846,-1.,0.175644148889271));
#20974=CARTESIAN_POINT('Ctrl Pts',(1.87563767773249,-1.,0.175563480746205));
#20975=CARTESIAN_POINT('Ctrl Pts',(1.86828349694972,-1.,0.1752683375909));
#20976=CARTESIAN_POINT('Ctrl Pts',(1.85948367089838,-1.,0.174735259276856));
#20977=CARTESIAN_POINT('Ctrl Pts',(1.84898113200543,-1.,0.173946627589401));
#20978=CARTESIAN_POINT('Ctrl Pts',(1.83658380530747,-1.,0.17288944289442));
#20979=CARTESIAN_POINT('Ctrl Pts',(1.82215766815414,-1.,0.171554770207306));
#20980=CARTESIAN_POINT('Ctrl Pts',(1.80561530633924,-1.,0.169936923908078));
#20981=CARTESIAN_POINT('Ctrl Pts',(1.78690649988931,-1.,0.16803277280837));
#20982=CARTESIAN_POINT('Ctrl Pts',(1.77018771687692,-1.,0.166279355148738));
#20983=CARTESIAN_POINT('Ctrl Pts',(1.75666056640041,-1.,0.164834765708484));
#20984=CARTESIAN_POINT('Ctrl Pts',(1.74720349503904,-1.,0.163814161002474));
#20985=CARTESIAN_POINT('Ctrl Pts',(1.74236521665491,-1.,0.163289472382896));
#20986=CARTESIAN_POINT('',(1.7075470150345,-1.,0.383122945602004));
#20987=CARTESIAN_POINT('Origin',(0.,-1.,0.));
#20988=CARTESIAN_POINT('',(2.11275013067528,-1.,0.613422273260091));
#20989=CARTESIAN_POINT('Ctrl Pts',(1.7075470150345,-1.,0.383122945602004));
#20990=CARTESIAN_POINT('Ctrl Pts',(1.71231062891398,-1.,0.384119047314215));
#20991=CARTESIAN_POINT('Ctrl Pts',(1.72162022244582,-1.,0.386070790323281));
#20992=CARTESIAN_POINT('Ctrl Pts',(1.73493170972829,-1.,0.388877023502615));
#20993=CARTESIAN_POINT('Ctrl Pts',(1.75137405310193,-1.,0.392375812285396));
#20994=CARTESIAN_POINT('Ctrl Pts',(1.76975560043442,-1.,0.396346196110688));
#20995=CARTESIAN_POINT('Ctrl Pts',(1.78598826343754,-1.,0.399919403774156));
#20996=CARTESIAN_POINT('Ctrl Pts',(1.80012077173238,-1.,0.403107976163396));
#20997=CARTESIAN_POINT('Ctrl Pts',(1.81223801812013,-1.,0.405933518407176));
#20998=CARTESIAN_POINT('Ctrl Pts',(1.82247022677562,-1.,0.408428948106228));
#20999=CARTESIAN_POINT('Ctrl Pts',(1.83100408895047,-1.,0.410641256301276));
#21000=CARTESIAN_POINT('Ctrl Pts',(1.8380895347617,-1.,0.412633125322945));
#21001=CARTESIAN_POINT('Ctrl Pts',(1.84405757074218,-1.,0.414487438255542));
#21002=CARTESIAN_POINT('Ctrl Pts',(1.84929312930314,-1.,0.416300022039885));
#21003=CARTESIAN_POINT('Ctrl Pts',(1.8541763285645,-1.,0.418164129144046));
#21004=CARTESIAN_POINT('Ctrl Pts',(1.8590328109667,-1.,0.420157287975583));
#21005=CARTESIAN_POINT('Ctrl Pts',(1.86408083333863,-1.,0.422327307417885));
#21006=CARTESIAN_POINT('Ctrl Pts',(1.8693780394412,-1.,0.424678177290876));
#21007=CARTESIAN_POINT('Ctrl Pts',(1.87486989291333,-1.,0.427183828518743));
#21008=CARTESIAN_POINT('Ctrl Pts',(1.88044229001778,-1.,0.429803062482217));
#21009=CARTESIAN_POINT('Ctrl Pts',(1.88596913666828,-1.,0.432493038548833));
#21010=CARTESIAN_POINT('Ctrl Pts',(1.89136993975585,-1.,0.43522566096358));
#21011=CARTESIAN_POINT('Ctrl Pts',(1.89663648956549,-1.,0.437995003948443));
#21012=CARTESIAN_POINT('Ctrl Pts',(1.90180124389137,-1.,0.440807833704161));
#21013=CARTESIAN_POINT('Ctrl Pts',(1.90691756144906,-1.,0.443677556849171));
#21014=CARTESIAN_POINT('Ctrl Pts',(1.91203699981095,-1.,0.446617343485651));
#21015=CARTESIAN_POINT('Ctrl Pts',(1.91718342555717,-1.,0.449632260106572));
#21016=CARTESIAN_POINT('Ctrl Pts',(1.9223538064847,-1.,0.452719478359356));
#21017=CARTESIAN_POINT('Ctrl Pts',(1.92753067150461,-1.,0.455872005174336));
#21018=CARTESIAN_POINT('Ctrl Pts',(1.93269066517936,-1.,0.459081234547932));
#21019=CARTESIAN_POINT('Ctrl Pts',(1.93781486640834,-1.,0.462340031009087));
#21020=CARTESIAN_POINT('Ctrl Pts',(1.94289794196205,-1.,0.465645462026065));
#21021=CARTESIAN_POINT('Ctrl Pts',(1.94794381136524,-1.,0.468997482913158));
#21022=CARTESIAN_POINT('Ctrl Pts',(1.95296148278136,-1.,0.47239767226408));
#21023=CARTESIAN_POINT('Ctrl Pts',(1.95796111148175,-1.,0.475848034683172));
#21024=CARTESIAN_POINT('Ctrl Pts',(1.96294933055938,-1.,0.479349583074846));
#21025=CARTESIAN_POINT('Ctrl Pts',(1.96792703422358,-1.,0.482901662120687));
#21026=CARTESIAN_POINT('Ctrl Pts',(1.97289186263272,-1.,0.486502692907661));
#21027=CARTESIAN_POINT('Ctrl Pts',(1.97783973019229,-1.,0.490150627860955));
#21028=CARTESIAN_POINT('Ctrl Pts',(1.9827665876182,-1.,0.493843476541493));
#21029=CARTESIAN_POINT('Ctrl Pts',(1.98767044752929,-1.,0.497579909545564));
#21030=CARTESIAN_POINT('Ctrl Pts',(1.9925514912615,-1.,0.501359287727129));
#21031=CARTESIAN_POINT('Ctrl Pts',(1.99741107463567,-1.,0.505181361323011));
#21032=CARTESIAN_POINT('Ctrl Pts',(2.00225107134733,-1.,0.509046069886152));
#21033=CARTESIAN_POINT('Ctrl Pts',(2.00707309946955,-1.,0.512953306961814));
#21034=CARTESIAN_POINT('Ctrl Pts',(2.01187773939257,-1.,0.516902681728733));
#21035=CARTESIAN_POINT('Ctrl Pts',(2.01666477917305,-1.,0.520893590399429));
#21036=CARTESIAN_POINT('Ctrl Pts',(2.02143356304712,-1.,0.524925318333519));
#21037=CARTESIAN_POINT('Ctrl Pts',(2.02618329083289,-1.,0.528997127241911));
#21038=CARTESIAN_POINT('Ctrl Pts',(2.03091336214401,-1.,0.533108355132905));
#21039=CARTESIAN_POINT('Ctrl Pts',(2.03562362953993,-1.,0.537258489833135));
#21040=CARTESIAN_POINT('Ctrl Pts',(2.0403142269048,-1.,0.54144712061552));
#21041=CARTESIAN_POINT('Ctrl Pts',(2.0449854471456,-1.,0.545673903817349));
#21042=CARTESIAN_POINT('Ctrl Pts',(2.04963761077974,-1.,0.549938525150342));
#21043=CARTESIAN_POINT('Ctrl Pts',(2.05427091604482,-1.,0.55424065746411));
#21044=CARTESIAN_POINT('Ctrl Pts',(2.05888537756571,-1.,0.558579940185468));
#21045=CARTESIAN_POINT('Ctrl Pts',(2.06348090160697,-1.,0.562955993082574));
#21046=CARTESIAN_POINT('Ctrl Pts',(2.06805732997383,-1.,0.56736842118123));
#21047=CARTESIAN_POINT('Ctrl Pts',(2.07261449292757,-1.,0.571816823242411));
#21048=CARTESIAN_POINT('Ctrl Pts',(2.07715226767361,-1.,0.576300797416275));
#21049=CARTESIAN_POINT('Ctrl Pts',(2.08167059018138,-1.,0.580819952107257));
#21050=CARTESIAN_POINT('Ctrl Pts',(2.086169437277,-1.,0.585373918990895));
#21051=CARTESIAN_POINT('Ctrl Pts',(2.09064881812053,-1.,0.58996236540319));
#21052=CARTESIAN_POINT('Ctrl Pts',(2.09510876220501,-1.,0.594585006052824));
#21053=CARTESIAN_POINT('Ctrl Pts',(2.09954930865331,-1.,0.599241616422144));
#21054=CARTESIAN_POINT('Ctrl Pts',(2.10397049887709,-1.,0.603932030738212));
#21055=CARTESIAN_POINT('Ctrl Pts',(2.10749199615859,-1.,0.607711315456826));
#21056=CARTESIAN_POINT('Ctrl Pts',(2.11012443807661,-1.,0.610560911691114));
#21057=CARTESIAN_POINT('Ctrl Pts',(2.11187554260142,-1.,0.61246736556225));
#21058=CARTESIAN_POINT('Ctrl Pts',(2.11275013067528,-1.,0.613422273260091));
#21059=CARTESIAN_POINT('',(2.0698113262342,-1.,0.745574324794401));
#21060=CARTESIAN_POINT('',(2.11275013067528,-1.,0.613422273260091));
#21061=CARTESIAN_POINT('Ctrl Pts',(2.0698113262342,-1.,0.745574324794401));
#21062=CARTESIAN_POINT('Ctrl Pts',(2.06854248895575,-1.,0.74583279137781));
#21063=CARTESIAN_POINT('Ctrl Pts',(2.06600523016401,-1.,0.746345871542696));
#21064=CARTESIAN_POINT('Ctrl Pts',(2.06220058927162,-1.,0.747103932785504));
#21065=CARTESIAN_POINT('Ctrl Pts',(2.05713023030263,-1.,0.748091554181101));
#21066=CARTESIAN_POINT('Ctrl Pts',(2.05079645591606,-1.,0.749287468663053));
#21067=CARTESIAN_POINT('Ctrl Pts',(2.04446689147754,-1.,0.750444657874758));
#21068=CARTESIAN_POINT('Ctrl Pts',(2.03814160092173,-1.,0.751562963361384));
#21069=CARTESIAN_POINT('Ctrl Pts',(2.03182068456467,-1.,0.752642180488104));
#21070=CARTESIAN_POINT('Ctrl Pts',(2.02550428623587,-1.,0.753682061113766));
#21071=CARTESIAN_POINT('Ctrl Pts',(2.01919259406003,-1.,0.75468233072352));
#21072=CARTESIAN_POINT('Ctrl Pts',(2.01288584328149,-1.,0.755642704958101));
#21073=CARTESIAN_POINT('Ctrl Pts',(2.00658431587682,-1.,0.756562904646496));
#21074=CARTESIAN_POINT('Ctrl Pts',(2.00028834739072,-1.,0.757442676862342));
#21075=CARTESIAN_POINT('Ctrl Pts',(1.9939983109871,-1.,0.758281796766377));
#21076=CARTESIAN_POINT('Ctrl Pts',(1.98771456680806,-1.,0.759080037802243));
#21077=CARTESIAN_POINT('Ctrl Pts',(1.98143741418156,-1.,0.759837147452135));
#21078=CARTESIAN_POINT('Ctrl Pts',(1.97516705321521,-1.,0.760552825409856));
#21079=CARTESIAN_POINT('Ctrl Pts',(1.96890351582545,-1.,0.761226690483986));
#21080=CARTESIAN_POINT('Ctrl Pts',(1.96264672744229,-1.,0.761858300014575));
#21081=CARTESIAN_POINT('Ctrl Pts',(1.95639665309893,-1.,0.762447203806264));
#21082=CARTESIAN_POINT('Ctrl Pts',(1.95015342590025,-1.,0.762992990878774));
#21083=CARTESIAN_POINT('Ctrl Pts',(1.94391746617626,-1.,0.763495333538581));
#21084=CARTESIAN_POINT('Ctrl Pts',(1.93768964875867,-1.,0.763954049121394));
#21085=CARTESIAN_POINT('Ctrl Pts',(1.93147105496367,-1.,0.76436901067389));
#21086=CARTESIAN_POINT('Ctrl Pts',(1.92526263537041,-1.,0.764740025488189));
#21087=CARTESIAN_POINT('Ctrl Pts',(1.91906491634197,-1.,0.765066729667095));
#21088=CARTESIAN_POINT('Ctrl Pts',(1.91287765805174,-1.,0.765348465884739));
#21089=CARTESIAN_POINT('Ctrl Pts',(1.90669961402362,-1.,0.765584196937937));
#21090=CARTESIAN_POINT('Ctrl Pts',(1.90052930393599,-1.,0.765772772593395));
#21091=CARTESIAN_POINT('Ctrl Pts',(1.89436577771389,-1.,0.765913193856979));
#21092=CARTESIAN_POINT('Ctrl Pts',(1.88820926433409,-1.,0.76600483706209));
#21093=CARTESIAN_POINT('Ctrl Pts',(1.88206215302561,-1.,0.766047794851869));
#21094=CARTESIAN_POINT('Ctrl Pts',(1.87592888967886,-1.,0.766042837036759));
#21095=CARTESIAN_POINT('Ctrl Pts',(1.86981398314345,-1.,0.765990708546112));
#21096=CARTESIAN_POINT('Ctrl Pts',(1.86372027063314,-1.,0.765891519092557));
#21097=CARTESIAN_POINT('Ctrl Pts',(1.85764741390391,-1.,0.765744212909305));
#21098=CARTESIAN_POINT('Ctrl Pts',(1.85158945130054,-1.,0.765545710619023));
#21099=CARTESIAN_POINT('Ctrl Pts',(1.8455369887591,-1.,0.765291664861972));
#21100=CARTESIAN_POINT('Ctrl Pts',(1.83948181064823,-1.,0.764978057881688));
#21101=CARTESIAN_POINT('Ctrl Pts',(1.8334207722714,-1.,0.764602549687846));
#21102=CARTESIAN_POINT('Ctrl Pts',(1.8273599120008,-1.,0.764165902606056));
#21103=CARTESIAN_POINT('Ctrl Pts',(1.82131873145297,-1.,0.763673465462854));
#21104=CARTESIAN_POINT('Ctrl Pts',(1.81532118405566,-1.,0.763132003836783));
#21105=CARTESIAN_POINT('Ctrl Pts',(1.80938551463989,-1.,0.762546129464036));
#21106=CARTESIAN_POINT('Ctrl Pts',(1.80351583877334,-1.,0.761915336443516));
#21107=CARTESIAN_POINT('Ctrl Pts',(1.79768986997735,-1.,0.761229695230359));
#21108=CARTESIAN_POINT('Ctrl Pts',(1.79185815610802,-1.,0.760469555880425));
#21109=CARTESIAN_POINT('Ctrl Pts',(1.78596964884526,-1.,0.759614401109868));
#21110=CARTESIAN_POINT('Ctrl Pts',(1.77999411220912,-1.,0.75865062667738));
#21111=CARTESIAN_POINT('Ctrl Pts',(1.77394167108342,-1.,0.757578264077238));
#21112=CARTESIAN_POINT('Ctrl Pts',(1.76789396003141,-1.,0.756421896028403));
#21113=CARTESIAN_POINT('Ctrl Pts',(1.7619781724032,-1.,0.755220979975262));
#21114=CARTESIAN_POINT('Ctrl Pts',(1.75631083600175,-1.,0.75400925402848));
#21115=CARTESIAN_POINT('Ctrl Pts',(1.75095139468809,-1.,0.752797683531377));
#21116=CARTESIAN_POINT('Ctrl Pts',(1.74585086852298,-1.,0.751555614163629));
#21117=CARTESIAN_POINT('Ctrl Pts',(1.74080458266705,-1.,0.750193435979541));
#21118=CARTESIAN_POINT('Ctrl Pts',(1.73550351679848,-1.,0.748582462954855));
#21119=CARTESIAN_POINT('Ctrl Pts',(1.72958533647399,-1.,0.746574710096437));
#21120=CARTESIAN_POINT('Ctrl Pts',(1.7226822991693,-1.,0.744021445433765));
#21121=CARTESIAN_POINT('Ctrl Pts',(1.71447789751927,-1.,0.740795162032088));
#21122=CARTESIAN_POINT('Ctrl Pts',(1.70473309006121,-1.,0.736799665724771));
#21123=CARTESIAN_POINT('Ctrl Pts',(1.69326921975743,-1.,0.731963238697195));
#21124=CARTESIAN_POINT('Ctrl Pts',(1.67996158455503,-1.,0.726235967997433));
#21125=CARTESIAN_POINT('Ctrl Pts',(1.6647288055568,-1.,0.719585433804282));
#21126=CARTESIAN_POINT('Ctrl Pts',(1.64752408832016,-1.,0.711993139355394));
#21127=CARTESIAN_POINT('Ctrl Pts',(1.63216541664676,-1.,0.705159151988319));
#21128=CARTESIAN_POINT('Ctrl Pts',(1.61974673472612,-1.,0.699605146405088));
#21129=CARTESIAN_POINT('Ctrl Pts',(1.61106790958151,-1.,0.695712097881194));
#21130=CARTESIAN_POINT('Ctrl Pts',(1.60662857109684,-1.,0.693717979106306));
#21131=CARTESIAN_POINT('Origin',(0.,-1.,0.));
#21132=CARTESIAN_POINT('Origin',(0.,0.,0.));
#21133=CARTESIAN_POINT('Origin',(0.,2.2,0.));
#21134=CARTESIAN_POINT('Origin',(0.,1.,0.));
#21135=CARTESIAN_POINT('',(-1.4,2.2,1.71450551880629E-16));
#21136=CARTESIAN_POINT('Origin',(0.,2.2,0.));
#21137=CARTESIAN_POINT('',(-1.4,1.,1.71450551880629E-16));
#21138=CARTESIAN_POINT('',(-1.4,1.,1.71450551880629E-16));
#21139=CARTESIAN_POINT('Origin',(0.,1.,0.));
#21140=CARTESIAN_POINT('Origin',(0.,2.2,0.));
#21141=CARTESIAN_POINT('Ctrl Pts',(2.11275013067528,-1.,0.613422273260091));
#21142=CARTESIAN_POINT('Ctrl Pts',(2.11275013067528,1.,0.613422273260091));
#21143=CARTESIAN_POINT('Ctrl Pts',(2.11187554260142,-1.,0.61246736556225));
#21144=CARTESIAN_POINT('Ctrl Pts',(2.11187554260142,1.,0.61246736556225));
#21145=CARTESIAN_POINT('Ctrl Pts',(2.11012443807661,-1.,0.610560911691114));
#21146=CARTESIAN_POINT('Ctrl Pts',(2.11012443807661,1.,0.610560911691114));
#21147=CARTESIAN_POINT('Ctrl Pts',(2.10749199615859,-1.,0.607711315456826));
#21148=CARTESIAN_POINT('Ctrl Pts',(2.10749199615859,1.,0.607711315456826));
#21149=CARTESIAN_POINT('Ctrl Pts',(2.10397049887709,-1.,0.603932030738212));
#21150=CARTESIAN_POINT('Ctrl Pts',(2.10397049887709,1.,0.603932030738212));
#21151=CARTESIAN_POINT('Ctrl Pts',(2.09954930865331,-1.,0.599241616422144));
#21152=CARTESIAN_POINT('Ctrl Pts',(2.09954930865331,1.,0.599241616422144));
#21153=CARTESIAN_POINT('Ctrl Pts',(2.09510876220501,-1.,0.594585006052824));
#21154=CARTESIAN_POINT('Ctrl Pts',(2.09510876220501,1.,0.594585006052824));
#21155=CARTESIAN_POINT('Ctrl Pts',(2.09064881812053,-1.,0.58996236540319));
#21156=CARTESIAN_POINT('Ctrl Pts',(2.09064881812053,1.,0.58996236540319));
#21157=CARTESIAN_POINT('Ctrl Pts',(2.086169437277,-1.,0.585373918990895));
#21158=CARTESIAN_POINT('Ctrl Pts',(2.086169437277,1.,0.585373918990895));
#21159=CARTESIAN_POINT('Ctrl Pts',(2.08167059018138,-1.,0.580819952107257));
#21160=CARTESIAN_POINT('Ctrl Pts',(2.08167059018138,1.,0.580819952107257));
#21161=CARTESIAN_POINT('Ctrl Pts',(2.07715226767361,-1.,0.576300797416275));
#21162=CARTESIAN_POINT('Ctrl Pts',(2.07715226767361,1.,0.576300797416275));
#21163=CARTESIAN_POINT('Ctrl Pts',(2.07261449292757,-1.,0.571816823242411));
#21164=CARTESIAN_POINT('Ctrl Pts',(2.07261449292757,1.,0.571816823242411));
#21165=CARTESIAN_POINT('Ctrl Pts',(2.06805732997383,-1.,0.56736842118123));
#21166=CARTESIAN_POINT('Ctrl Pts',(2.06805732997383,1.,0.56736842118123));
#21167=CARTESIAN_POINT('Ctrl Pts',(2.06348090160697,-1.,0.562955993082574));
#21168=CARTESIAN_POINT('Ctrl Pts',(2.06348090160697,1.,0.562955993082574));
#21169=CARTESIAN_POINT('Ctrl Pts',(2.05888537756571,-1.,0.558579940185468));
#21170=CARTESIAN_POINT('Ctrl Pts',(2.05888537756571,1.,0.558579940185468));
#21171=CARTESIAN_POINT('Ctrl Pts',(2.05427091604482,-1.,0.55424065746411));
#21172=CARTESIAN_POINT('Ctrl Pts',(2.05427091604482,1.,0.55424065746411));
#21173=CARTESIAN_POINT('Ctrl Pts',(2.04963761077974,-1.,0.549938525150342));
#21174=CARTESIAN_POINT('Ctrl Pts',(2.04963761077974,1.,0.549938525150342));
#21175=CARTESIAN_POINT('Ctrl Pts',(2.0449854471456,-1.,0.545673903817349));
#21176=CARTESIAN_POINT('Ctrl Pts',(2.0449854471456,1.,0.545673903817349));
#21177=CARTESIAN_POINT('Ctrl Pts',(2.0403142269048,-1.,0.54144712061552));
#21178=CARTESIAN_POINT('Ctrl Pts',(2.0403142269048,1.,0.54144712061552));
#21179=CARTESIAN_POINT('Ctrl Pts',(2.03562362953993,-1.,0.537258489833135));
#21180=CARTESIAN_POINT('Ctrl Pts',(2.03562362953993,1.,0.537258489833135));
#21181=CARTESIAN_POINT('Ctrl Pts',(2.03091336214401,-1.,0.533108355132905));
#21182=CARTESIAN_POINT('Ctrl Pts',(2.03091336214401,1.,0.533108355132905));
#21183=CARTESIAN_POINT('Ctrl Pts',(2.02618329083289,-1.,0.528997127241911));
#21184=CARTESIAN_POINT('Ctrl Pts',(2.02618329083289,1.,0.528997127241911));
#21185=CARTESIAN_POINT('Ctrl Pts',(2.02143356304712,-1.,0.524925318333519));
#21186=CARTESIAN_POINT('Ctrl Pts',(2.02143356304712,1.,0.524925318333519));
#21187=CARTESIAN_POINT('Ctrl Pts',(2.01666477917305,-1.,0.520893590399429));
#21188=CARTESIAN_POINT('Ctrl Pts',(2.01666477917305,1.,0.520893590399429));
#21189=CARTESIAN_POINT('Ctrl Pts',(2.01187773939257,-1.,0.516902681728733));
#21190=CARTESIAN_POINT('Ctrl Pts',(2.01187773939257,1.,0.516902681728733));
#21191=CARTESIAN_POINT('Ctrl Pts',(2.00707309946955,-1.,0.512953306961814));
#21192=CARTESIAN_POINT('Ctrl Pts',(2.00707309946955,1.,0.512953306961814));
#21193=CARTESIAN_POINT('Ctrl Pts',(2.00225107134733,-1.,0.509046069886152));
#21194=CARTESIAN_POINT('Ctrl Pts',(2.00225107134733,1.,0.509046069886152));
#21195=CARTESIAN_POINT('Ctrl Pts',(1.99741107463567,-1.,0.505181361323011));
#21196=CARTESIAN_POINT('Ctrl Pts',(1.99741107463567,1.,0.505181361323011));
#21197=CARTESIAN_POINT('Ctrl Pts',(1.9925514912615,-1.,0.501359287727129));
#21198=CARTESIAN_POINT('Ctrl Pts',(1.9925514912615,1.,0.501359287727129));
#21199=CARTESIAN_POINT('Ctrl Pts',(1.98767044752929,-1.,0.497579909545564));
#21200=CARTESIAN_POINT('Ctrl Pts',(1.98767044752929,1.,0.497579909545564));
#21201=CARTESIAN_POINT('Ctrl Pts',(1.9827665876182,-1.,0.493843476541493));
#21202=CARTESIAN_POINT('Ctrl Pts',(1.9827665876182,1.,0.493843476541493));
#21203=CARTESIAN_POINT('Ctrl Pts',(1.97783973019229,-1.,0.490150627860955));
#21204=CARTESIAN_POINT('Ctrl Pts',(1.97783973019229,1.,0.490150627860955));
#21205=CARTESIAN_POINT('Ctrl Pts',(1.97289186263272,-1.,0.486502692907661));
#21206=CARTESIAN_POINT('Ctrl Pts',(1.97289186263272,1.,0.486502692907661));
#21207=CARTESIAN_POINT('Ctrl Pts',(1.96792703422358,-1.,0.482901662120687));
#21208=CARTESIAN_POINT('Ctrl Pts',(1.96792703422358,1.,0.482901662120687));
#21209=CARTESIAN_POINT('Ctrl Pts',(1.96294933055938,-1.,0.479349583074846));
#21210=CARTESIAN_POINT('Ctrl Pts',(1.96294933055938,1.,0.479349583074846));
#21211=CARTESIAN_POINT('Ctrl Pts',(1.95796111148175,-1.,0.475848034683172));
#21212=CARTESIAN_POINT('Ctrl Pts',(1.95796111148175,1.,0.475848034683172));
#21213=CARTESIAN_POINT('Ctrl Pts',(1.95296148278136,-1.,0.47239767226408));
#21214=CARTESIAN_POINT('Ctrl Pts',(1.95296148278136,1.,0.47239767226408));
#21215=CARTESIAN_POINT('Ctrl Pts',(1.94794381136524,-1.,0.468997482913158));
#21216=CARTESIAN_POINT('Ctrl Pts',(1.94794381136524,1.,0.468997482913158));
#21217=CARTESIAN_POINT('Ctrl Pts',(1.94289794196205,-1.,0.465645462026065));
#21218=CARTESIAN_POINT('Ctrl Pts',(1.94289794196205,1.,0.465645462026065));
#21219=CARTESIAN_POINT('Ctrl Pts',(1.93781486640834,-1.,0.462340031009087));
#21220=CARTESIAN_POINT('Ctrl Pts',(1.93781486640834,1.,0.462340031009087));
#21221=CARTESIAN_POINT('Ctrl Pts',(1.93269066517936,-1.,0.459081234547932));
#21222=CARTESIAN_POINT('Ctrl Pts',(1.93269066517936,1.,0.459081234547932));
#21223=CARTESIAN_POINT('Ctrl Pts',(1.92753067150461,-1.,0.455872005174336));
#21224=CARTESIAN_POINT('Ctrl Pts',(1.92753067150461,1.,0.455872005174336));
#21225=CARTESIAN_POINT('Ctrl Pts',(1.9223538064847,-1.,0.452719478359356));
#21226=CARTESIAN_POINT('Ctrl Pts',(1.9223538064847,1.,0.452719478359356));
#21227=CARTESIAN_POINT('Ctrl Pts',(1.91718342555717,-1.,0.449632260106572));
#21228=CARTESIAN_POINT('Ctrl Pts',(1.91718342555717,1.,0.449632260106572));
#21229=CARTESIAN_POINT('Ctrl Pts',(1.91203699981095,-1.,0.446617343485651));
#21230=CARTESIAN_POINT('Ctrl Pts',(1.91203699981095,1.,0.446617343485651));
#21231=CARTESIAN_POINT('Ctrl Pts',(1.90691756144906,-1.,0.443677556849171));
#21232=CARTESIAN_POINT('Ctrl Pts',(1.90691756144906,1.,0.443677556849171));
#21233=CARTESIAN_POINT('Ctrl Pts',(1.90180124389137,-1.,0.440807833704161));
#21234=CARTESIAN_POINT('Ctrl Pts',(1.90180124389137,1.,0.440807833704161));
#21235=CARTESIAN_POINT('Ctrl Pts',(1.89663648956549,-1.,0.437995003948443));
#21236=CARTESIAN_POINT('Ctrl Pts',(1.89663648956549,1.,0.437995003948443));
#21237=CARTESIAN_POINT('Ctrl Pts',(1.89136993975585,-1.,0.43522566096358));
#21238=CARTESIAN_POINT('Ctrl Pts',(1.89136993975585,1.,0.43522566096358));
#21239=CARTESIAN_POINT('Ctrl Pts',(1.88596913666828,-1.,0.432493038548833));
#21240=CARTESIAN_POINT('Ctrl Pts',(1.88596913666828,1.,0.432493038548833));
#21241=CARTESIAN_POINT('Ctrl Pts',(1.88044229001778,-1.,0.429803062482217));
#21242=CARTESIAN_POINT('Ctrl Pts',(1.88044229001778,1.,0.429803062482217));
#21243=CARTESIAN_POINT('Ctrl Pts',(1.87486989291333,-1.,0.427183828518743));
#21244=CARTESIAN_POINT('Ctrl Pts',(1.87486989291333,1.,0.427183828518743));
#21245=CARTESIAN_POINT('Ctrl Pts',(1.8693780394412,-1.,0.424678177290876));
#21246=CARTESIAN_POINT('Ctrl Pts',(1.8693780394412,1.,0.424678177290876));
#21247=CARTESIAN_POINT('Ctrl Pts',(1.86408083333863,-1.,0.422327307417885));
#21248=CARTESIAN_POINT('Ctrl Pts',(1.86408083333863,1.,0.422327307417885));
#21249=CARTESIAN_POINT('Ctrl Pts',(1.8590328109667,-1.,0.420157287975583));
#21250=CARTESIAN_POINT('Ctrl Pts',(1.8590328109667,1.,0.420157287975583));
#21251=CARTESIAN_POINT('Ctrl Pts',(1.8541763285645,-1.,0.418164129144046));
#21252=CARTESIAN_POINT('Ctrl Pts',(1.8541763285645,1.,0.418164129144046));
#21253=CARTESIAN_POINT('Ctrl Pts',(1.84929312930314,-1.,0.416300022039885));
#21254=CARTESIAN_POINT('Ctrl Pts',(1.84929312930314,1.,0.416300022039885));
#21255=CARTESIAN_POINT('Ctrl Pts',(1.84405757074218,-1.,0.414487438255542));
#21256=CARTESIAN_POINT('Ctrl Pts',(1.84405757074218,1.,0.414487438255542));
#21257=CARTESIAN_POINT('Ctrl Pts',(1.8380895347617,-1.,0.412633125322945));
#21258=CARTESIAN_POINT('Ctrl Pts',(1.8380895347617,1.,0.412633125322945));
#21259=CARTESIAN_POINT('Ctrl Pts',(1.83100408895047,-1.,0.410641256301276));
#21260=CARTESIAN_POINT('Ctrl Pts',(1.83100408895047,1.,0.410641256301276));
#21261=CARTESIAN_POINT('Ctrl Pts',(1.82247022677562,-1.,0.408428948106228));
#21262=CARTESIAN_POINT('Ctrl Pts',(1.82247022677562,1.,0.408428948106228));
#21263=CARTESIAN_POINT('Ctrl Pts',(1.81223801812013,-1.,0.405933518407176));
#21264=CARTESIAN_POINT('Ctrl Pts',(1.81223801812013,1.,0.405933518407176));
#21265=CARTESIAN_POINT('Ctrl Pts',(1.80012077173238,-1.,0.403107976163396));
#21266=CARTESIAN_POINT('Ctrl Pts',(1.80012077173238,1.,0.403107976163396));
#21267=CARTESIAN_POINT('Ctrl Pts',(1.78598826343754,-1.,0.399919403774156));
#21268=CARTESIAN_POINT('Ctrl Pts',(1.78598826343754,1.,0.399919403774156));
#21269=CARTESIAN_POINT('Ctrl Pts',(1.76975560043442,-1.,0.396346196110688));
#21270=CARTESIAN_POINT('Ctrl Pts',(1.76975560043442,1.,0.396346196110688));
#21271=CARTESIAN_POINT('Ctrl Pts',(1.75137405310193,-1.,0.392375812285396));
#21272=CARTESIAN_POINT('Ctrl Pts',(1.75137405310193,1.,0.392375812285396));
#21273=CARTESIAN_POINT('Ctrl Pts',(1.73493170972829,-1.,0.388877023502615));
#21274=CARTESIAN_POINT('Ctrl Pts',(1.73493170972829,1.,0.388877023502615));
#21275=CARTESIAN_POINT('Ctrl Pts',(1.72162022244582,-1.,0.386070790323281));
#21276=CARTESIAN_POINT('Ctrl Pts',(1.72162022244582,1.,0.386070790323281));
#21277=CARTESIAN_POINT('Ctrl Pts',(1.71231062891398,-1.,0.384119047314215));
#21278=CARTESIAN_POINT('Ctrl Pts',(1.71231062891398,1.,0.384119047314215));
#21279=CARTESIAN_POINT('Ctrl Pts',(1.7075470150345,-1.,0.383122945602004));
#21280=CARTESIAN_POINT('Ctrl Pts',(1.7075470150345,1.,0.383122945602004));
#21281=CARTESIAN_POINT('',(1.7075470150345,1.,0.383122945602004));
#21282=CARTESIAN_POINT('',(1.7075470150345,0.,0.383122945602005));
#21283=CARTESIAN_POINT('',(2.11275013067528,1.,0.613422273260091));
#21284=CARTESIAN_POINT('Ctrl Pts',(2.11275013067528,1.,0.613422273260091));
#21285=CARTESIAN_POINT('Ctrl Pts',(2.11187554260142,1.,0.61246736556225));
#21286=CARTESIAN_POINT('Ctrl Pts',(2.11012443807661,1.,0.610560911691114));
#21287=CARTESIAN_POINT('Ctrl Pts',(2.10749199615859,1.,0.607711315456826));
#21288=CARTESIAN_POINT('Ctrl Pts',(2.10397049887709,1.,0.603932030738212));
#21289=CARTESIAN_POINT('Ctrl Pts',(2.09954930865331,1.,0.599241616422144));
#21290=CARTESIAN_POINT('Ctrl Pts',(2.09510876220501,1.,0.594585006052824));
#21291=CARTESIAN_POINT('Ctrl Pts',(2.09064881812053,1.,0.58996236540319));
#21292=CARTESIAN_POINT('Ctrl Pts',(2.086169437277,1.,0.585373918990895));
#21293=CARTESIAN_POINT('Ctrl Pts',(2.08167059018138,1.,0.580819952107257));
#21294=CARTESIAN_POINT('Ctrl Pts',(2.07715226767361,1.,0.576300797416275));
#21295=CARTESIAN_POINT('Ctrl Pts',(2.07261449292757,1.,0.571816823242411));
#21296=CARTESIAN_POINT('Ctrl Pts',(2.06805732997383,1.,0.56736842118123));
#21297=CARTESIAN_POINT('Ctrl Pts',(2.06348090160697,1.,0.562955993082574));
#21298=CARTESIAN_POINT('Ctrl Pts',(2.05888537756571,1.,0.558579940185468));
#21299=CARTESIAN_POINT('Ctrl Pts',(2.05427091604482,1.,0.55424065746411));
#21300=CARTESIAN_POINT('Ctrl Pts',(2.04963761077974,1.,0.549938525150342));
#21301=CARTESIAN_POINT('Ctrl Pts',(2.0449854471456,1.,0.545673903817349));
#21302=CARTESIAN_POINT('Ctrl Pts',(2.0403142269048,1.,0.54144712061552));
#21303=CARTESIAN_POINT('Ctrl Pts',(2.03562362953993,1.,0.537258489833135));
#21304=CARTESIAN_POINT('Ctrl Pts',(2.03091336214401,1.,0.533108355132905));
#21305=CARTESIAN_POINT('Ctrl Pts',(2.02618329083289,1.,0.528997127241911));
#21306=CARTESIAN_POINT('Ctrl Pts',(2.02143356304712,1.,0.524925318333519));
#21307=CARTESIAN_POINT('Ctrl Pts',(2.01666477917305,1.,0.520893590399429));
#21308=CARTESIAN_POINT('Ctrl Pts',(2.01187773939257,1.,0.516902681728733));
#21309=CARTESIAN_POINT('Ctrl Pts',(2.00707309946955,1.,0.512953306961814));
#21310=CARTESIAN_POINT('Ctrl Pts',(2.00225107134733,1.,0.509046069886152));
#21311=CARTESIAN_POINT('Ctrl Pts',(1.99741107463567,1.,0.505181361323011));
#21312=CARTESIAN_POINT('Ctrl Pts',(1.9925514912615,1.,0.501359287727129));
#21313=CARTESIAN_POINT('Ctrl Pts',(1.98767044752929,1.,0.497579909545564));
#21314=CARTESIAN_POINT('Ctrl Pts',(1.9827665876182,1.,0.493843476541493));
#21315=CARTESIAN_POINT('Ctrl Pts',(1.97783973019229,1.,0.490150627860955));
#21316=CARTESIAN_POINT('Ctrl Pts',(1.97289186263272,1.,0.486502692907661));
#21317=CARTESIAN_POINT('Ctrl Pts',(1.96792703422358,1.,0.482901662120687));
#21318=CARTESIAN_POINT('Ctrl Pts',(1.96294933055938,1.,0.479349583074846));
#21319=CARTESIAN_POINT('Ctrl Pts',(1.95796111148175,1.,0.475848034683172));
#21320=CARTESIAN_POINT('Ctrl Pts',(1.95296148278136,1.,0.47239767226408));
#21321=CARTESIAN_POINT('Ctrl Pts',(1.94794381136524,1.,0.468997482913158));
#21322=CARTESIAN_POINT('Ctrl Pts',(1.94289794196205,1.,0.465645462026065));
#21323=CARTESIAN_POINT('Ctrl Pts',(1.93781486640834,1.,0.462340031009087));
#21324=CARTESIAN_POINT('Ctrl Pts',(1.93269066517936,1.,0.459081234547932));
#21325=CARTESIAN_POINT('Ctrl Pts',(1.92753067150461,1.,0.455872005174336));
#21326=CARTESIAN_POINT('Ctrl Pts',(1.9223538064847,1.,0.452719478359356));
#21327=CARTESIAN_POINT('Ctrl Pts',(1.91718342555717,1.,0.449632260106572));
#21328=CARTESIAN_POINT('Ctrl Pts',(1.91203699981095,1.,0.446617343485651));
#21329=CARTESIAN_POINT('Ctrl Pts',(1.90691756144906,1.,0.443677556849171));
#21330=CARTESIAN_POINT('Ctrl Pts',(1.90180124389137,1.,0.440807833704161));
#21331=CARTESIAN_POINT('Ctrl Pts',(1.89663648956549,1.,0.437995003948443));
#21332=CARTESIAN_POINT('Ctrl Pts',(1.89136993975585,1.,0.43522566096358));
#21333=CARTESIAN_POINT('Ctrl Pts',(1.88596913666828,1.,0.432493038548833));
#21334=CARTESIAN_POINT('Ctrl Pts',(1.88044229001778,1.,0.429803062482217));
#21335=CARTESIAN_POINT('Ctrl Pts',(1.87486989291333,1.,0.427183828518743));
#21336=CARTESIAN_POINT('Ctrl Pts',(1.8693780394412,1.,0.424678177290876));
#21337=CARTESIAN_POINT('Ctrl Pts',(1.86408083333863,1.,0.422327307417885));
#21338=CARTESIAN_POINT('Ctrl Pts',(1.8590328109667,1.,0.420157287975583));
#21339=CARTESIAN_POINT('Ctrl Pts',(1.8541763285645,1.,0.418164129144046));
#21340=CARTESIAN_POINT('Ctrl Pts',(1.84929312930314,1.,0.416300022039885));
#21341=CARTESIAN_POINT('Ctrl Pts',(1.84405757074218,1.,0.414487438255542));
#21342=CARTESIAN_POINT('Ctrl Pts',(1.8380895347617,1.,0.412633125322945));
#21343=CARTESIAN_POINT('Ctrl Pts',(1.83100408895047,1.,0.410641256301276));
#21344=CARTESIAN_POINT('Ctrl Pts',(1.82247022677562,1.,0.408428948106228));
#21345=CARTESIAN_POINT('Ctrl Pts',(1.81223801812013,1.,0.405933518407176));
#21346=CARTESIAN_POINT('Ctrl Pts',(1.80012077173238,1.,0.403107976163396));
#21347=CARTESIAN_POINT('Ctrl Pts',(1.78598826343754,1.,0.399919403774156));
#21348=CARTESIAN_POINT('Ctrl Pts',(1.76975560043442,1.,0.396346196110688));
#21349=CARTESIAN_POINT('Ctrl Pts',(1.75137405310193,1.,0.392375812285396));
#21350=CARTESIAN_POINT('Ctrl Pts',(1.73493170972829,1.,0.388877023502615));
#21351=CARTESIAN_POINT('Ctrl Pts',(1.72162022244582,1.,0.386070790323281));
#21352=CARTESIAN_POINT('Ctrl Pts',(1.71231062891398,1.,0.384119047314215));
#21353=CARTESIAN_POINT('Ctrl Pts',(1.7075470150345,1.,0.383122945602004));
#21354=CARTESIAN_POINT('',(2.11275013067528,0.,0.613422273260091));
#21355=CARTESIAN_POINT('Origin',(2.0698113262342,0.,0.745574324794401));
#21356=CARTESIAN_POINT('',(2.0698113262342,1.,0.745574324794401));
#21357=CARTESIAN_POINT('',(2.11275013067528,1.,0.613422273260091));
#21358=CARTESIAN_POINT('',(2.0698113262342,0.,0.745574324794401));
#21359=CARTESIAN_POINT('Ctrl Pts',(1.60662857109684,-1.,0.693717979106306));
#21360=CARTESIAN_POINT('Ctrl Pts',(1.60662857109684,1.,0.693717979106306));
#21361=CARTESIAN_POINT('Ctrl Pts',(1.61106790958151,-1.,0.695712097881194));
#21362=CARTESIAN_POINT('Ctrl Pts',(1.61106790958151,1.,0.695712097881194));
#21363=CARTESIAN_POINT('Ctrl Pts',(1.61974673472612,-1.,0.699605146405088));
#21364=CARTESIAN_POINT('Ctrl Pts',(1.61974673472612,1.,0.699605146405088));
#21365=CARTESIAN_POINT('Ctrl Pts',(1.63216541664676,-1.,0.705159151988319));
#21366=CARTESIAN_POINT('Ctrl Pts',(1.63216541664676,1.,0.705159151988319));
#21367=CARTESIAN_POINT('Ctrl Pts',(1.64752408832016,-1.,0.711993139355394));
#21368=CARTESIAN_POINT('Ctrl Pts',(1.64752408832016,1.,0.711993139355394));
#21369=CARTESIAN_POINT('Ctrl Pts',(1.6647288055568,-1.,0.719585433804282));
#21370=CARTESIAN_POINT('Ctrl Pts',(1.6647288055568,1.,0.719585433804282));
#21371=CARTESIAN_POINT('Ctrl Pts',(1.67996158455503,-1.,0.726235967997433));
#21372=CARTESIAN_POINT('Ctrl Pts',(1.67996158455503,1.,0.726235967997433));
#21373=CARTESIAN_POINT('Ctrl Pts',(1.69326921975743,-1.,0.731963238697195));
#21374=CARTESIAN_POINT('Ctrl Pts',(1.69326921975743,1.,0.731963238697195));
#21375=CARTESIAN_POINT('Ctrl Pts',(1.70473309006121,-1.,0.736799665724771));
#21376=CARTESIAN_POINT('Ctrl Pts',(1.70473309006121,1.,0.736799665724771));
#21377=CARTESIAN_POINT('Ctrl Pts',(1.71447789751927,-1.,0.740795162032088));
#21378=CARTESIAN_POINT('Ctrl Pts',(1.71447789751927,1.,0.740795162032088));
#21379=CARTESIAN_POINT('Ctrl Pts',(1.7226822991693,-1.,0.744021445433765));
#21380=CARTESIAN_POINT('Ctrl Pts',(1.7226822991693,1.,0.744021445433765));
#21381=CARTESIAN_POINT('Ctrl Pts',(1.72958533647399,-1.,0.746574710096437));
#21382=CARTESIAN_POINT('Ctrl Pts',(1.72958533647399,1.,0.746574710096437));
#21383=CARTESIAN_POINT('Ctrl Pts',(1.73550351679848,-1.,0.748582462954855));
#21384=CARTESIAN_POINT('Ctrl Pts',(1.73550351679848,1.,0.748582462954855));
#21385=CARTESIAN_POINT('Ctrl Pts',(1.74080458266705,-1.,0.750193435979541));
#21386=CARTESIAN_POINT('Ctrl Pts',(1.74080458266705,1.,0.750193435979541));
#21387=CARTESIAN_POINT('Ctrl Pts',(1.74585086852298,-1.,0.751555614163629));
#21388=CARTESIAN_POINT('Ctrl Pts',(1.74585086852298,1.,0.751555614163629));
#21389=CARTESIAN_POINT('Ctrl Pts',(1.75095139468809,-1.,0.752797683531377));
#21390=CARTESIAN_POINT('Ctrl Pts',(1.75095139468809,1.,0.752797683531377));
#21391=CARTESIAN_POINT('Ctrl Pts',(1.75631083600175,-1.,0.75400925402848));
#21392=CARTESIAN_POINT('Ctrl Pts',(1.75631083600175,1.,0.75400925402848));
#21393=CARTESIAN_POINT('Ctrl Pts',(1.7619781724032,-1.,0.755220979975262));
#21394=CARTESIAN_POINT('Ctrl Pts',(1.7619781724032,1.,0.755220979975262));
#21395=CARTESIAN_POINT('Ctrl Pts',(1.76789396003141,-1.,0.756421896028403));
#21396=CARTESIAN_POINT('Ctrl Pts',(1.76789396003141,1.,0.756421896028403));
#21397=CARTESIAN_POINT('Ctrl Pts',(1.77394167108342,-1.,0.757578264077238));
#21398=CARTESIAN_POINT('Ctrl Pts',(1.77394167108342,1.,0.757578264077238));
#21399=CARTESIAN_POINT('Ctrl Pts',(1.77999411220912,-1.,0.75865062667738));
#21400=CARTESIAN_POINT('Ctrl Pts',(1.77999411220912,1.,0.75865062667738));
#21401=CARTESIAN_POINT('Ctrl Pts',(1.78596964884526,-1.,0.759614401109868));
#21402=CARTESIAN_POINT('Ctrl Pts',(1.78596964884526,1.,0.759614401109868));
#21403=CARTESIAN_POINT('Ctrl Pts',(1.79185815610802,-1.,0.760469555880425));
#21404=CARTESIAN_POINT('Ctrl Pts',(1.79185815610802,1.,0.760469555880425));
#21405=CARTESIAN_POINT('Ctrl Pts',(1.79768986997735,-1.,0.761229695230359));
#21406=CARTESIAN_POINT('Ctrl Pts',(1.79768986997735,1.,0.761229695230359));
#21407=CARTESIAN_POINT('Ctrl Pts',(1.80351583877334,-1.,0.761915336443516));
#21408=CARTESIAN_POINT('Ctrl Pts',(1.80351583877334,1.,0.761915336443516));
#21409=CARTESIAN_POINT('Ctrl Pts',(1.80938551463989,-1.,0.762546129464036));
#21410=CARTESIAN_POINT('Ctrl Pts',(1.80938551463989,1.,0.762546129464036));
#21411=CARTESIAN_POINT('Ctrl Pts',(1.81532118405566,-1.,0.763132003836783));
#21412=CARTESIAN_POINT('Ctrl Pts',(1.81532118405566,1.,0.763132003836783));
#21413=CARTESIAN_POINT('Ctrl Pts',(1.82131873145297,-1.,0.763673465462854));
#21414=CARTESIAN_POINT('Ctrl Pts',(1.82131873145297,1.,0.763673465462854));
#21415=CARTESIAN_POINT('Ctrl Pts',(1.8273599120008,-1.,0.764165902606056));
#21416=CARTESIAN_POINT('Ctrl Pts',(1.8273599120008,1.,0.764165902606056));
#21417=CARTESIAN_POINT('Ctrl Pts',(1.8334207722714,-1.,0.764602549687846));
#21418=CARTESIAN_POINT('Ctrl Pts',(1.8334207722714,1.,0.764602549687846));
#21419=CARTESIAN_POINT('Ctrl Pts',(1.83948181064823,-1.,0.764978057881688));
#21420=CARTESIAN_POINT('Ctrl Pts',(1.83948181064823,1.,0.764978057881688));
#21421=CARTESIAN_POINT('Ctrl Pts',(1.8455369887591,-1.,0.765291664861972));
#21422=CARTESIAN_POINT('Ctrl Pts',(1.8455369887591,1.,0.765291664861972));
#21423=CARTESIAN_POINT('Ctrl Pts',(1.85158945130054,-1.,0.765545710619023));
#21424=CARTESIAN_POINT('Ctrl Pts',(1.85158945130054,1.,0.765545710619023));
#21425=CARTESIAN_POINT('Ctrl Pts',(1.85764741390391,-1.,0.765744212909305));
#21426=CARTESIAN_POINT('Ctrl Pts',(1.85764741390391,1.,0.765744212909305));
#21427=CARTESIAN_POINT('Ctrl Pts',(1.86372027063314,-1.,0.765891519092557));
#21428=CARTESIAN_POINT('Ctrl Pts',(1.86372027063314,1.,0.765891519092557));
#21429=CARTESIAN_POINT('Ctrl Pts',(1.86981398314345,-1.,0.765990708546112));
#21430=CARTESIAN_POINT('Ctrl Pts',(1.86981398314345,1.,0.765990708546112));
#21431=CARTESIAN_POINT('Ctrl Pts',(1.87592888967886,-1.,0.766042837036759));
#21432=CARTESIAN_POINT('Ctrl Pts',(1.87592888967886,1.,0.766042837036759));
#21433=CARTESIAN_POINT('Ctrl Pts',(1.88206215302561,-1.,0.766047794851869));
#21434=CARTESIAN_POINT('Ctrl Pts',(1.88206215302561,1.,0.766047794851869));
#21435=CARTESIAN_POINT('Ctrl Pts',(1.88820926433409,-1.,0.76600483706209));
#21436=CARTESIAN_POINT('Ctrl Pts',(1.88820926433409,1.,0.76600483706209));
#21437=CARTESIAN_POINT('Ctrl Pts',(1.89436577771389,-1.,0.765913193856979));
#21438=CARTESIAN_POINT('Ctrl Pts',(1.89436577771389,1.,0.765913193856979));
#21439=CARTESIAN_POINT('Ctrl Pts',(1.90052930393599,-1.,0.765772772593395));
#21440=CARTESIAN_POINT('Ctrl Pts',(1.90052930393599,1.,0.765772772593395));
#21441=CARTESIAN_POINT('Ctrl Pts',(1.90669961402362,-1.,0.765584196937937));
#21442=CARTESIAN_POINT('Ctrl Pts',(1.90669961402362,1.,0.765584196937937));
#21443=CARTESIAN_POINT('Ctrl Pts',(1.91287765805174,-1.,0.765348465884739));
#21444=CARTESIAN_POINT('Ctrl Pts',(1.91287765805174,1.,0.765348465884739));
#21445=CARTESIAN_POINT('Ctrl Pts',(1.91906491634197,-1.,0.765066729667095));
#21446=CARTESIAN_POINT('Ctrl Pts',(1.91906491634197,1.,0.765066729667095));
#21447=CARTESIAN_POINT('Ctrl Pts',(1.92526263537041,-1.,0.764740025488189));
#21448=CARTESIAN_POINT('Ctrl Pts',(1.92526263537041,1.,0.764740025488189));
#21449=CARTESIAN_POINT('Ctrl Pts',(1.93147105496367,-1.,0.76436901067389));
#21450=CARTESIAN_POINT('Ctrl Pts',(1.93147105496367,1.,0.76436901067389));
#21451=CARTESIAN_POINT('Ctrl Pts',(1.93768964875867,-1.,0.763954049121394));
#21452=CARTESIAN_POINT('Ctrl Pts',(1.93768964875867,1.,0.763954049121394));
#21453=CARTESIAN_POINT('Ctrl Pts',(1.94391746617626,-1.,0.763495333538581));
#21454=CARTESIAN_POINT('Ctrl Pts',(1.94391746617626,1.,0.763495333538581));
#21455=CARTESIAN_POINT('Ctrl Pts',(1.95015342590025,-1.,0.762992990878774));
#21456=CARTESIAN_POINT('Ctrl Pts',(1.95015342590025,1.,0.762992990878774));
#21457=CARTESIAN_POINT('Ctrl Pts',(1.95639665309893,-1.,0.762447203806264));
#21458=CARTESIAN_POINT('Ctrl Pts',(1.95639665309893,1.,0.762447203806264));
#21459=CARTESIAN_POINT('Ctrl Pts',(1.96264672744229,-1.,0.761858300014575));
#21460=CARTESIAN_POINT('Ctrl Pts',(1.96264672744229,1.,0.761858300014575));
#21461=CARTESIAN_POINT('Ctrl Pts',(1.96890351582545,-1.,0.761226690483986));
#21462=CARTESIAN_POINT('Ctrl Pts',(1.96890351582545,1.,0.761226690483986));
#21463=CARTESIAN_POINT('Ctrl Pts',(1.97516705321521,-1.,0.760552825409856));
#21464=CARTESIAN_POINT('Ctrl Pts',(1.97516705321521,1.,0.760552825409856));
#21465=CARTESIAN_POINT('Ctrl Pts',(1.98143741418156,-1.,0.759837147452135));
#21466=CARTESIAN_POINT('Ctrl Pts',(1.98143741418156,1.,0.759837147452135));
#21467=CARTESIAN_POINT('Ctrl Pts',(1.98771456680806,-1.,0.759080037802243));
#21468=CARTESIAN_POINT('Ctrl Pts',(1.98771456680806,1.,0.759080037802243));
#21469=CARTESIAN_POINT('Ctrl Pts',(1.9939983109871,-1.,0.758281796766377));
#21470=CARTESIAN_POINT('Ctrl Pts',(1.9939983109871,1.,0.758281796766377));
#21471=CARTESIAN_POINT('Ctrl Pts',(2.00028834739072,-1.,0.757442676862342));
#21472=CARTESIAN_POINT('Ctrl Pts',(2.00028834739072,1.,0.757442676862342));
#21473=CARTESIAN_POINT('Ctrl Pts',(2.00658431587682,-1.,0.756562904646496));
#21474=CARTESIAN_POINT('Ctrl Pts',(2.00658431587682,1.,0.756562904646496));
#21475=CARTESIAN_POINT('Ctrl Pts',(2.01288584328149,-1.,0.755642704958101));
#21476=CARTESIAN_POINT('Ctrl Pts',(2.01288584328149,1.,0.755642704958101));
#21477=CARTESIAN_POINT('Ctrl Pts',(2.01919259406003,-1.,0.75468233072352));
#21478=CARTESIAN_POINT('Ctrl Pts',(2.01919259406003,1.,0.75468233072352));
#21479=CARTESIAN_POINT('Ctrl Pts',(2.02550428623587,-1.,0.753682061113766));
#21480=CARTESIAN_POINT('Ctrl Pts',(2.02550428623587,1.,0.753682061113766));
#21481=CARTESIAN_POINT('Ctrl Pts',(2.03182068456467,-1.,0.752642180488104));
#21482=CARTESIAN_POINT('Ctrl Pts',(2.03182068456467,1.,0.752642180488104));
#21483=CARTESIAN_POINT('Ctrl Pts',(2.03814160092173,-1.,0.751562963361384));
#21484=CARTESIAN_POINT('Ctrl Pts',(2.03814160092173,1.,0.751562963361384));
#21485=CARTESIAN_POINT('Ctrl Pts',(2.04446689147754,-1.,0.750444657874758));
#21486=CARTESIAN_POINT('Ctrl Pts',(2.04446689147754,1.,0.750444657874758));
#21487=CARTESIAN_POINT('Ctrl Pts',(2.05079645591606,-1.,0.749287468663053));
#21488=CARTESIAN_POINT('Ctrl Pts',(2.05079645591606,1.,0.749287468663053));
#21489=CARTESIAN_POINT('Ctrl Pts',(2.05713023030263,-1.,0.748091554181101));
#21490=CARTESIAN_POINT('Ctrl Pts',(2.05713023030263,1.,0.748091554181101));
#21491=CARTESIAN_POINT('Ctrl Pts',(2.06220058927162,-1.,0.747103932785504));
#21492=CARTESIAN_POINT('Ctrl Pts',(2.06220058927162,1.,0.747103932785504));
#21493=CARTESIAN_POINT('Ctrl Pts',(2.06600523016401,-1.,0.746345871542696));
#21494=CARTESIAN_POINT('Ctrl Pts',(2.06600523016401,1.,0.746345871542696));
#21495=CARTESIAN_POINT('Ctrl Pts',(2.06854248895575,-1.,0.74583279137781));
#21496=CARTESIAN_POINT('Ctrl Pts',(2.06854248895575,1.,0.74583279137781));
#21497=CARTESIAN_POINT('Ctrl Pts',(2.0698113262342,-1.,0.745574324794401));
#21498=CARTESIAN_POINT('Ctrl Pts',(2.0698113262342,1.,0.745574324794401));
#21499=CARTESIAN_POINT('',(1.60662857109684,1.,0.693717979106306));
#21500=CARTESIAN_POINT('Ctrl Pts',(1.60662857109684,1.,0.693717979106306));
#21501=CARTESIAN_POINT('Ctrl Pts',(1.61106790958151,1.,0.695712097881194));
#21502=CARTESIAN_POINT('Ctrl Pts',(1.61974673472612,1.,0.699605146405088));
#21503=CARTESIAN_POINT('Ctrl Pts',(1.63216541664676,1.,0.705159151988319));
#21504=CARTESIAN_POINT('Ctrl Pts',(1.64752408832016,1.,0.711993139355394));
#21505=CARTESIAN_POINT('Ctrl Pts',(1.6647288055568,1.,0.719585433804282));
#21506=CARTESIAN_POINT('Ctrl Pts',(1.67996158455503,1.,0.726235967997433));
#21507=CARTESIAN_POINT('Ctrl Pts',(1.69326921975743,1.,0.731963238697195));
#21508=CARTESIAN_POINT('Ctrl Pts',(1.70473309006121,1.,0.736799665724771));
#21509=CARTESIAN_POINT('Ctrl Pts',(1.71447789751927,1.,0.740795162032088));
#21510=CARTESIAN_POINT('Ctrl Pts',(1.7226822991693,1.,0.744021445433765));
#21511=CARTESIAN_POINT('Ctrl Pts',(1.72958533647399,1.,0.746574710096437));
#21512=CARTESIAN_POINT('Ctrl Pts',(1.73550351679848,1.,0.748582462954855));
#21513=CARTESIAN_POINT('Ctrl Pts',(1.74080458266705,1.,0.750193435979541));
#21514=CARTESIAN_POINT('Ctrl Pts',(1.74585086852298,1.,0.751555614163629));
#21515=CARTESIAN_POINT('Ctrl Pts',(1.75095139468809,1.,0.752797683531377));
#21516=CARTESIAN_POINT('Ctrl Pts',(1.75631083600175,1.,0.75400925402848));
#21517=CARTESIAN_POINT('Ctrl Pts',(1.7619781724032,1.,0.755220979975262));
#21518=CARTESIAN_POINT('Ctrl Pts',(1.76789396003141,1.,0.756421896028403));
#21519=CARTESIAN_POINT('Ctrl Pts',(1.77394167108342,1.,0.757578264077238));
#21520=CARTESIAN_POINT('Ctrl Pts',(1.77999411220912,1.,0.75865062667738));
#21521=CARTESIAN_POINT('Ctrl Pts',(1.78596964884526,1.,0.759614401109868));
#21522=CARTESIAN_POINT('Ctrl Pts',(1.79185815610802,1.,0.760469555880425));
#21523=CARTESIAN_POINT('Ctrl Pts',(1.79768986997735,1.,0.761229695230359));
#21524=CARTESIAN_POINT('Ctrl Pts',(1.80351583877334,1.,0.761915336443516));
#21525=CARTESIAN_POINT('Ctrl Pts',(1.80938551463989,1.,0.762546129464036));
#21526=CARTESIAN_POINT('Ctrl Pts',(1.81532118405566,1.,0.763132003836783));
#21527=CARTESIAN_POINT('Ctrl Pts',(1.82131873145297,1.,0.763673465462854));
#21528=CARTESIAN_POINT('Ctrl Pts',(1.8273599120008,1.,0.764165902606056));
#21529=CARTESIAN_POINT('Ctrl Pts',(1.8334207722714,1.,0.764602549687846));
#21530=CARTESIAN_POINT('Ctrl Pts',(1.83948181064823,1.,0.764978057881688));
#21531=CARTESIAN_POINT('Ctrl Pts',(1.8455369887591,1.,0.765291664861972));
#21532=CARTESIAN_POINT('Ctrl Pts',(1.85158945130054,1.,0.765545710619023));
#21533=CARTESIAN_POINT('Ctrl Pts',(1.85764741390391,1.,0.765744212909305));
#21534=CARTESIAN_POINT('Ctrl Pts',(1.86372027063314,1.,0.765891519092557));
#21535=CARTESIAN_POINT('Ctrl Pts',(1.86981398314345,1.,0.765990708546112));
#21536=CARTESIAN_POINT('Ctrl Pts',(1.87592888967886,1.,0.766042837036759));
#21537=CARTESIAN_POINT('Ctrl Pts',(1.88206215302561,1.,0.766047794851869));
#21538=CARTESIAN_POINT('Ctrl Pts',(1.88820926433409,1.,0.76600483706209));
#21539=CARTESIAN_POINT('Ctrl Pts',(1.89436577771389,1.,0.765913193856979));
#21540=CARTESIAN_POINT('Ctrl Pts',(1.90052930393599,1.,0.765772772593395));
#21541=CARTESIAN_POINT('Ctrl Pts',(1.90669961402362,1.,0.765584196937937));
#21542=CARTESIAN_POINT('Ctrl Pts',(1.91287765805174,1.,0.765348465884739));
#21543=CARTESIAN_POINT('Ctrl Pts',(1.91906491634197,1.,0.765066729667095));
#21544=CARTESIAN_POINT('Ctrl Pts',(1.92526263537041,1.,0.764740025488189));
#21545=CARTESIAN_POINT('Ctrl Pts',(1.93147105496367,1.,0.76436901067389));
#21546=CARTESIAN_POINT('Ctrl Pts',(1.93768964875867,1.,0.763954049121394));
#21547=CARTESIAN_POINT('Ctrl Pts',(1.94391746617626,1.,0.763495333538581));
#21548=CARTESIAN_POINT('Ctrl Pts',(1.95015342590025,1.,0.762992990878774));
#21549=CARTESIAN_POINT('Ctrl Pts',(1.95639665309893,1.,0.762447203806264));
#21550=CARTESIAN_POINT('Ctrl Pts',(1.96264672744229,1.,0.761858300014575));
#21551=CARTESIAN_POINT('Ctrl Pts',(1.96890351582545,1.,0.761226690483986));
#21552=CARTESIAN_POINT('Ctrl Pts',(1.97516705321521,1.,0.760552825409856));
#21553=CARTESIAN_POINT('Ctrl Pts',(1.98143741418156,1.,0.759837147452135));
#21554=CARTESIAN_POINT('Ctrl Pts',(1.98771456680806,1.,0.759080037802243));
#21555=CARTESIAN_POINT('Ctrl Pts',(1.9939983109871,1.,0.758281796766377));
#21556=CARTESIAN_POINT('Ctrl Pts',(2.00028834739072,1.,0.757442676862342));
#21557=CARTESIAN_POINT('Ctrl Pts',(2.00658431587682,1.,0.756562904646496));
#21558=CARTESIAN_POINT('Ctrl Pts',(2.01288584328149,1.,0.755642704958101));
#21559=CARTESIAN_POINT('Ctrl Pts',(2.01919259406003,1.,0.75468233072352));
#21560=CARTESIAN_POINT('Ctrl Pts',(2.02550428623587,1.,0.753682061113766));
#21561=CARTESIAN_POINT('Ctrl Pts',(2.03182068456467,1.,0.752642180488104));
#21562=CARTESIAN_POINT('Ctrl Pts',(2.03814160092173,1.,0.751562963361384));
#21563=CARTESIAN_POINT('Ctrl Pts',(2.04446689147754,1.,0.750444657874758));
#21564=CARTESIAN_POINT('Ctrl Pts',(2.05079645591606,1.,0.749287468663053));
#21565=CARTESIAN_POINT('Ctrl Pts',(2.05713023030263,1.,0.748091554181101));
#21566=CARTESIAN_POINT('Ctrl Pts',(2.06220058927162,1.,0.747103932785504));
#21567=CARTESIAN_POINT('Ctrl Pts',(2.06600523016401,1.,0.746345871542696));
#21568=CARTESIAN_POINT('Ctrl Pts',(2.06854248895575,1.,0.74583279137781));
#21569=CARTESIAN_POINT('Ctrl Pts',(2.0698113262342,1.,0.745574324794401));
#21570=CARTESIAN_POINT('',(1.60662857109684,0.,0.693717979106305));
#21571=CARTESIAN_POINT('Origin',(0.,0.,0.));
#21572=CARTESIAN_POINT('',(1.5055822144029,1.,0.892032620296856));
#21573=CARTESIAN_POINT('Origin',(0.,1.,0.));
#21574=CARTESIAN_POINT('',(1.5055822144029,0.,0.892032620296855));
#21575=CARTESIAN_POINT('Ctrl Pts',(1.81978687191668,-1.,1.23627494547115));
#21576=CARTESIAN_POINT('Ctrl Pts',(1.81978687191668,1.,1.23627494547115));
#21577=CARTESIAN_POINT('Ctrl Pts',(1.81925017193666,-1.,1.23509651170476));
#21578=CARTESIAN_POINT('Ctrl Pts',(1.81925017193666,1.,1.23509651170476));
#21579=CARTESIAN_POINT('Ctrl Pts',(1.81817389921279,-1.,1.2327422452705));
#21580=CARTESIAN_POINT('Ctrl Pts',(1.81817389921279,1.,1.2327422452705));
#21581=CARTESIAN_POINT('Ctrl Pts',(1.8165508718364,-1.,1.2292186489137));
#21582=CARTESIAN_POINT('Ctrl Pts',(1.8165508718364,1.,1.2292186489137));
#21583=CARTESIAN_POINT('Ctrl Pts',(1.81436959210434,-1.,1.2245361330495));
#21584=CARTESIAN_POINT('Ctrl Pts',(1.81436959210434,1.,1.2245361330495));
#21585=CARTESIAN_POINT('Ctrl Pts',(1.81161420806656,-1.,1.21870906103557));
#21586=CARTESIAN_POINT('Ctrl Pts',(1.81161420806656,1.,1.21870906103557));
#21587=CARTESIAN_POINT('Ctrl Pts',(1.80882996917129,-1.,1.21290815708314));
#21588=CARTESIAN_POINT('Ctrl Pts',(1.80882996917129,1.,1.21290815708314));
#21589=CARTESIAN_POINT('Ctrl Pts',(1.80601678480707,-1.,1.20713356605475));
#21590=CARTESIAN_POINT('Ctrl Pts',(1.80601678480707,1.,1.20713356605475));
#21591=CARTESIAN_POINT('Ctrl Pts',(1.80317454838603,-1.,1.20138548938974));
#21592=CARTESIAN_POINT('Ctrl Pts',(1.80317454838603,1.,1.20138548938974));
#21593=CARTESIAN_POINT('Ctrl Pts',(1.80030314369879,-1.,1.19566418930242));
#21594=CARTESIAN_POINT('Ctrl Pts',(1.80030314369879,1.,1.19566418930242));
#21595=CARTESIAN_POINT('Ctrl Pts',(1.79740245923478,-1.,1.18996997934445));
#21596=CARTESIAN_POINT('Ctrl Pts',(1.79740245923478,1.,1.18996997934445));
#21597=CARTESIAN_POINT('Ctrl Pts',(1.79447240321515,-1.,1.18430321697432));
#21598=CARTESIAN_POINT('Ctrl Pts',(1.79447240321515,1.,1.18430321697432));
#21599=CARTESIAN_POINT('Ctrl Pts',(1.79151291552689,-1.,1.17866429440809));
#21600=CARTESIAN_POINT('Ctrl Pts',(1.79151291552689,1.,1.17866429440809));
#21601=CARTESIAN_POINT('Ctrl Pts',(1.78852398877616,-1.,1.17305363177328));
#21602=CARTESIAN_POINT('Ctrl Pts',(1.78852398877616,1.,1.17305363177328));
#21603=CARTESIAN_POINT('Ctrl Pts',(1.78550566040443,-1.,1.16747166312303));
#21604=CARTESIAN_POINT('Ctrl Pts',(1.78550566040443,1.,1.16747166312303));
#21605=CARTESIAN_POINT('Ctrl Pts',(1.78245795881009,-1.,1.16191881298499));
#21606=CARTESIAN_POINT('Ctrl Pts',(1.78245795881009,1.,1.16191881298499));
#21607=CARTESIAN_POINT('Ctrl Pts',(1.77938085564275,-1.,1.15639547194698));
#21608=CARTESIAN_POINT('Ctrl Pts',(1.77938085564275,1.,1.15639547194698));
#21609=CARTESIAN_POINT('Ctrl Pts',(1.7762742255701,-1.,1.15090197841515));
#21610=CARTESIAN_POINT('Ctrl Pts',(1.7762742255701,1.,1.15090197841515));
#21611=CARTESIAN_POINT('Ctrl Pts',(1.77313777896194,-1.,1.1454385822692));
#21612=CARTESIAN_POINT('Ctrl Pts',(1.77313777896194,1.,1.1454385822692));
#21613=CARTESIAN_POINT('Ctrl Pts',(1.76997111386769,-1.,1.14000548336975));
#21614=CARTESIAN_POINT('Ctrl Pts',(1.76997111386769,1.,1.14000548336975));
#21615=CARTESIAN_POINT('Ctrl Pts',(1.76677384551862,-1.,1.1346029180462));
#21616=CARTESIAN_POINT('Ctrl Pts',(1.76677384551862,1.,1.1346029180462));
#21617=CARTESIAN_POINT('Ctrl Pts',(1.7635457196617,-1.,1.12923123555075));
#21618=CARTESIAN_POINT('Ctrl Pts',(1.7635457196617,1.,1.12923123555075));
#21619=CARTESIAN_POINT('Ctrl Pts',(1.76028671825096,-1.,1.12389096855086));
#21620=CARTESIAN_POINT('Ctrl Pts',(1.76028671825096,1.,1.12389096855086));
#21621=CARTESIAN_POINT('Ctrl Pts',(1.75699720772105,-1.,1.11858293216763));
#21622=CARTESIAN_POINT('Ctrl Pts',(1.75699720772105,1.,1.11858293216763));
#21623=CARTESIAN_POINT('Ctrl Pts',(1.7536777209463,-1.,1.11330807582551));
#21624=CARTESIAN_POINT('Ctrl Pts',(1.7536777209463,1.,1.11330807582551));
#21625=CARTESIAN_POINT('Ctrl Pts',(1.7503286607592,-1.,1.10806728183007));
#21626=CARTESIAN_POINT('Ctrl Pts',(1.7503286607592,1.,1.10806728183007));
#21627=CARTESIAN_POINT('Ctrl Pts',(1.74695004214923,-1.,1.10286118991143));
#21628=CARTESIAN_POINT('Ctrl Pts',(1.74695004214923,1.,1.10286118991143));
#21629=CARTESIAN_POINT('Ctrl Pts',(1.74354119236208,-1.,1.09768999241226));
#21630=CARTESIAN_POINT('Ctrl Pts',(1.74354119236208,1.,1.09768999241226));
#21631=CARTESIAN_POINT('Ctrl Pts',(1.74010053962247,-1.,1.09255329056493));
#21632=CARTESIAN_POINT('Ctrl Pts',(1.74010053962247,1.,1.09255329056493));
#21633=CARTESIAN_POINT('Ctrl Pts',(1.73662628326091,-1.,1.08745056285427));
#21634=CARTESIAN_POINT('Ctrl Pts',(1.73662628326091,1.,1.08745056285427));
#21635=CARTESIAN_POINT('Ctrl Pts',(1.73311705663407,-1.,1.08238162784749));
#21636=CARTESIAN_POINT('Ctrl Pts',(1.73311705663407,1.,1.08238162784749));
#21637=CARTESIAN_POINT('Ctrl Pts',(1.72957248977424,-1.,1.0773470373727));
#21638=CARTESIAN_POINT('Ctrl Pts',(1.72957248977424,1.,1.0773470373727));
#21639=CARTESIAN_POINT('Ctrl Pts',(1.72599406198488,-1.,1.07234866990252));
#21640=CARTESIAN_POINT('Ctrl Pts',(1.72599406198488,1.,1.07234866990252));
#21641=CARTESIAN_POINT('Ctrl Pts',(1.72238500928453,-1.,1.06738966975462));
#21642=CARTESIAN_POINT('Ctrl Pts',(1.72238500928453,1.,1.06738966975462));
#21643=CARTESIAN_POINT('Ctrl Pts',(1.71874858456904,-1.,1.06247324680647));
#21644=CARTESIAN_POINT('Ctrl Pts',(1.71874858456904,1.,1.06247324680647));
#21645=CARTESIAN_POINT('Ctrl Pts',(1.7150865442702,-1.,1.05760163192479));
#21646=CARTESIAN_POINT('Ctrl Pts',(1.7150865442702,1.,1.05760163192479));
#21647=CARTESIAN_POINT('Ctrl Pts',(1.71139783543989,-1.,1.05277517202855));
#21648=CARTESIAN_POINT('Ctrl Pts',(1.71139783543989,1.,1.05277517202855));
#21649=CARTESIAN_POINT('Ctrl Pts',(1.70767646263649,-1.,1.04799085404995));
#21650=CARTESIAN_POINT('Ctrl Pts',(1.70767646263649,1.,1.04799085404995));
#21651=CARTESIAN_POINT('Ctrl Pts',(1.70391338707982,-1.,1.04324363334554));
#21652=CARTESIAN_POINT('Ctrl Pts',(1.70391338707982,1.,1.04324363334554));
#21653=CARTESIAN_POINT('Ctrl Pts',(1.70010052930962,-1.,1.03852922490789));
#21654=CARTESIAN_POINT('Ctrl Pts',(1.70010052930962,1.,1.03852922490789));
#21655=CARTESIAN_POINT('Ctrl Pts',(1.69623414782771,-1.,1.03384646003588));
#21656=CARTESIAN_POINT('Ctrl Pts',(1.69623414782771,1.,1.03384646003588));
#21657=CARTESIAN_POINT('Ctrl Pts',(1.69231840863458,-1.,1.02919977579147));
#21658=CARTESIAN_POINT('Ctrl Pts',(1.69231840863458,1.,1.02919977579147));
#21659=CARTESIAN_POINT('Ctrl Pts',(1.68836910178447,-1.,1.02460180535255));
#21660=CARTESIAN_POINT('Ctrl Pts',(1.68836910178447,1.,1.02460180535255));
#21661=CARTESIAN_POINT('Ctrl Pts',(1.68440578021706,-1.,1.02006795074201));
#21662=CARTESIAN_POINT('Ctrl Pts',(1.68440578021706,1.,1.02006795074201));
#21663=CARTESIAN_POINT('Ctrl Pts',(1.68044289894798,-1.,1.01561026162773));
#21664=CARTESIAN_POINT('Ctrl Pts',(1.68044289894798,1.,1.01561026162773));
#21665=CARTESIAN_POINT('Ctrl Pts',(1.67648246776464,-1.,1.01123236493511));
#21666=CARTESIAN_POINT('Ctrl Pts',(1.67648246776464,1.,1.01123236493511));
#21667=CARTESIAN_POINT('Ctrl Pts',(1.67250335383293,-1.,1.00692206696414));
#21668=CARTESIAN_POINT('Ctrl Pts',(1.67250335383293,1.,1.00692206696414));
#21669=CARTESIAN_POINT('Ctrl Pts',(1.66846059277303,-1.,1.00265091003727));
#21670=CARTESIAN_POINT('Ctrl Pts',(1.66846059277303,1.,1.00265091003727));
#21671=CARTESIAN_POINT('Ctrl Pts',(1.66430758030376,-1.,0.998389654952758));
#21672=CARTESIAN_POINT('Ctrl Pts',(1.66430758030376,1.,0.998389654952758));
#21673=CARTESIAN_POINT('Ctrl Pts',(1.66001553809947,-1.,0.994121836661306));
#21674=CARTESIAN_POINT('Ctrl Pts',(1.66001553809947,1.,0.994121836661306));
#21675=CARTESIAN_POINT('Ctrl Pts',(1.65559044289699,-1.,0.989855627854165));
#21676=CARTESIAN_POINT('Ctrl Pts',(1.65559044289699,1.,0.989855627854165));
#21677=CARTESIAN_POINT('Ctrl Pts',(1.65110016612638,-1.,0.985642622920821));
#21678=CARTESIAN_POINT('Ctrl Pts',(1.65110016612638,1.,0.985642622920821));
#21679=CARTESIAN_POINT('Ctrl Pts',(1.64665139190656,-1.,0.981562530939489));
#21680=CARTESIAN_POINT('Ctrl Pts',(1.64665139190656,1.,0.981562530939489));
#21681=CARTESIAN_POINT('Ctrl Pts',(1.64233990826687,-1.,0.977689794119417));
#21682=CARTESIAN_POINT('Ctrl Pts',(1.64233990826687,1.,0.977689794119417));
#21683=CARTESIAN_POINT('Ctrl Pts',(1.63820952658144,-1.,0.974066058287419));
#21684=CARTESIAN_POINT('Ctrl Pts',(1.63820952658144,1.,0.974066058287419));
#21685=CARTESIAN_POINT('Ctrl Pts',(1.63420665729798,-1.,0.970669715997509));
#21686=CARTESIAN_POINT('Ctrl Pts',(1.63420665729798,1.,0.970669715997509));
#21687=CARTESIAN_POINT('Ctrl Pts',(1.63013849959461,-1.,0.967387853230345));
#21688=CARTESIAN_POINT('Ctrl Pts',(1.63013849959461,1.,0.967387853230345));
#21689=CARTESIAN_POINT('Ctrl Pts',(1.62571930670187,-1.,0.964046107040536));
#21690=CARTESIAN_POINT('Ctrl Pts',(1.62571930670187,1.,0.964046107040536));
#21691=CARTESIAN_POINT('Ctrl Pts',(1.62061638140221,-1.,0.960438326101729));
#21692=CARTESIAN_POINT('Ctrl Pts',(1.62061638140221,1.,0.960438326101729));
#21693=CARTESIAN_POINT('Ctrl Pts',(1.61449324337085,-1.,0.956354422920671));
#21694=CARTESIAN_POINT('Ctrl Pts',(1.61449324337085,1.,0.956354422920671));
#21695=CARTESIAN_POINT('Ctrl Pts',(1.60706069896936,-1.,0.951613284356035));
#21696=CARTESIAN_POINT('Ctrl Pts',(1.60706069896936,1.,0.951613284356035));
#21697=CARTESIAN_POINT('Ctrl Pts',(1.59810042043673,-1.,0.946078063315257));
#21698=CARTESIAN_POINT('Ctrl Pts',(1.59810042043673,1.,0.946078063315257));
#21699=CARTESIAN_POINT('Ctrl Pts',(1.58744937487176,-1.,0.939646377893399));
#21700=CARTESIAN_POINT('Ctrl Pts',(1.58744937487176,1.,0.939646377893399));
#21701=CARTESIAN_POINT('Ctrl Pts',(1.57499388382243,-1.,0.932246680108685));
#21702=CARTESIAN_POINT('Ctrl Pts',(1.57499388382243,1.,0.932246680108685));
#21703=CARTESIAN_POINT('Ctrl Pts',(1.56065988578893,-1.,0.923832188944341));
#21704=CARTESIAN_POINT('Ctrl Pts',(1.56065988578893,1.,0.923832188944341));
#21705=CARTESIAN_POINT('Ctrl Pts',(1.54440491149498,-1.,0.914375919026456));
#21706=CARTESIAN_POINT('Ctrl Pts',(1.54440491149498,1.,0.914375919026456));
#21707=CARTESIAN_POINT('Ctrl Pts',(1.52984849887993,-1.,0.905967409625651));
#21708=CARTESIAN_POINT('Ctrl Pts',(1.52984849887993,1.,0.905967409625651));
#21709=CARTESIAN_POINT('Ctrl Pts',(1.51805569590094,-1.,0.899185047483511));
#21710=CARTESIAN_POINT('Ctrl Pts',(1.51805569590094,1.,0.899185047483511));
#21711=CARTESIAN_POINT('Ctrl Pts',(1.50980486806688,-1.,0.894452006964544));
#21712=CARTESIAN_POINT('Ctrl Pts',(1.50980486806688,1.,0.894452006964544));
#21713=CARTESIAN_POINT('Ctrl Pts',(1.5055822144029,-1.,0.892032620296856));
#21714=CARTESIAN_POINT('Ctrl Pts',(1.5055822144029,1.,0.892032620296856));
#21715=CARTESIAN_POINT('',(1.81978687191668,1.,1.23627494547115));
#21716=CARTESIAN_POINT('Ctrl Pts',(1.81978687191668,1.,1.23627494547115));
#21717=CARTESIAN_POINT('Ctrl Pts',(1.81925017193666,1.,1.23509651170476));
#21718=CARTESIAN_POINT('Ctrl Pts',(1.81817389921279,1.,1.2327422452705));
#21719=CARTESIAN_POINT('Ctrl Pts',(1.8165508718364,1.,1.2292186489137));
#21720=CARTESIAN_POINT('Ctrl Pts',(1.81436959210434,1.,1.2245361330495));
#21721=CARTESIAN_POINT('Ctrl Pts',(1.81161420806656,1.,1.21870906103557));
#21722=CARTESIAN_POINT('Ctrl Pts',(1.80882996917129,1.,1.21290815708314));
#21723=CARTESIAN_POINT('Ctrl Pts',(1.80601678480707,1.,1.20713356605475));
#21724=CARTESIAN_POINT('Ctrl Pts',(1.80317454838603,1.,1.20138548938974));
#21725=CARTESIAN_POINT('Ctrl Pts',(1.80030314369879,1.,1.19566418930242));
#21726=CARTESIAN_POINT('Ctrl Pts',(1.79740245923478,1.,1.18996997934445));
#21727=CARTESIAN_POINT('Ctrl Pts',(1.79447240321515,1.,1.18430321697432));
#21728=CARTESIAN_POINT('Ctrl Pts',(1.79151291552689,1.,1.17866429440809));
#21729=CARTESIAN_POINT('Ctrl Pts',(1.78852398877616,1.,1.17305363177328));
#21730=CARTESIAN_POINT('Ctrl Pts',(1.78550566040443,1.,1.16747166312303));
#21731=CARTESIAN_POINT('Ctrl Pts',(1.78245795881009,1.,1.16191881298499));
#21732=CARTESIAN_POINT('Ctrl Pts',(1.77938085564275,1.,1.15639547194698));
#21733=CARTESIAN_POINT('Ctrl Pts',(1.7762742255701,1.,1.15090197841515));
#21734=CARTESIAN_POINT('Ctrl Pts',(1.77313777896194,1.,1.1454385822692));
#21735=CARTESIAN_POINT('Ctrl Pts',(1.76997111386769,1.,1.14000548336975));
#21736=CARTESIAN_POINT('Ctrl Pts',(1.76677384551862,1.,1.1346029180462));
#21737=CARTESIAN_POINT('Ctrl Pts',(1.7635457196617,1.,1.12923123555075));
#21738=CARTESIAN_POINT('Ctrl Pts',(1.76028671825096,1.,1.12389096855086));
#21739=CARTESIAN_POINT('Ctrl Pts',(1.75699720772105,1.,1.11858293216763));
#21740=CARTESIAN_POINT('Ctrl Pts',(1.7536777209463,1.,1.11330807582551));
#21741=CARTESIAN_POINT('Ctrl Pts',(1.7503286607592,1.,1.10806728183007));
#21742=CARTESIAN_POINT('Ctrl Pts',(1.74695004214923,1.,1.10286118991143));
#21743=CARTESIAN_POINT('Ctrl Pts',(1.74354119236208,1.,1.09768999241226));
#21744=CARTESIAN_POINT('Ctrl Pts',(1.74010053962247,1.,1.09255329056493));
#21745=CARTESIAN_POINT('Ctrl Pts',(1.73662628326091,1.,1.08745056285427));
#21746=CARTESIAN_POINT('Ctrl Pts',(1.73311705663407,1.,1.08238162784749));
#21747=CARTESIAN_POINT('Ctrl Pts',(1.72957248977424,1.,1.0773470373727));
#21748=CARTESIAN_POINT('Ctrl Pts',(1.72599406198488,1.,1.07234866990252));
#21749=CARTESIAN_POINT('Ctrl Pts',(1.72238500928453,1.,1.06738966975462));
#21750=CARTESIAN_POINT('Ctrl Pts',(1.71874858456904,1.,1.06247324680647));
#21751=CARTESIAN_POINT('Ctrl Pts',(1.7150865442702,1.,1.05760163192479));
#21752=CARTESIAN_POINT('Ctrl Pts',(1.71139783543989,1.,1.05277517202855));
#21753=CARTESIAN_POINT('Ctrl Pts',(1.70767646263649,1.,1.04799085404995));
#21754=CARTESIAN_POINT('Ctrl Pts',(1.70391338707982,1.,1.04324363334554));
#21755=CARTESIAN_POINT('Ctrl Pts',(1.70010052930962,1.,1.03852922490789));
#21756=CARTESIAN_POINT('Ctrl Pts',(1.69623414782771,1.,1.03384646003588));
#21757=CARTESIAN_POINT('Ctrl Pts',(1.69231840863458,1.,1.02919977579147));
#21758=CARTESIAN_POINT('Ctrl Pts',(1.68836910178447,1.,1.02460180535255));
#21759=CARTESIAN_POINT('Ctrl Pts',(1.68440578021706,1.,1.02006795074201));
#21760=CARTESIAN_POINT('Ctrl Pts',(1.68044289894798,1.,1.01561026162773));
#21761=CARTESIAN_POINT('Ctrl Pts',(1.67648246776464,1.,1.01123236493511));
#21762=CARTESIAN_POINT('Ctrl Pts',(1.67250335383293,1.,1.00692206696414));
#21763=CARTESIAN_POINT('Ctrl Pts',(1.66846059277303,1.,1.00265091003727));
#21764=CARTESIAN_POINT('Ctrl Pts',(1.66430758030376,1.,0.998389654952758));
#21765=CARTESIAN_POINT('Ctrl Pts',(1.66001553809947,1.,0.994121836661306));
#21766=CARTESIAN_POINT('Ctrl Pts',(1.65559044289699,1.,0.989855627854165));
#21767=CARTESIAN_POINT('Ctrl Pts',(1.65110016612638,1.,0.985642622920821));
#21768=CARTESIAN_POINT('Ctrl Pts',(1.64665139190656,1.,0.981562530939489));
#21769=CARTESIAN_POINT('Ctrl Pts',(1.64233990826687,1.,0.977689794119417));
#21770=CARTESIAN_POINT('Ctrl Pts',(1.63820952658144,1.,0.974066058287419));
#21771=CARTESIAN_POINT('Ctrl Pts',(1.63420665729798,1.,0.970669715997509));
#21772=CARTESIAN_POINT('Ctrl Pts',(1.63013849959461,1.,0.967387853230345));
#21773=CARTESIAN_POINT('Ctrl Pts',(1.62571930670187,1.,0.964046107040536));
#21774=CARTESIAN_POINT('Ctrl Pts',(1.62061638140221,1.,0.960438326101729));
#21775=CARTESIAN_POINT('Ctrl Pts',(1.61449324337085,1.,0.956354422920671));
#21776=CARTESIAN_POINT('Ctrl Pts',(1.60706069896936,1.,0.951613284356035));
#21777=CARTESIAN_POINT('Ctrl Pts',(1.59810042043673,1.,0.946078063315257));
#21778=CARTESIAN_POINT('Ctrl Pts',(1.58744937487176,1.,0.939646377893399));
#21779=CARTESIAN_POINT('Ctrl Pts',(1.57499388382243,1.,0.932246680108685));
#21780=CARTESIAN_POINT('Ctrl Pts',(1.56065988578893,1.,0.923832188944341));
#21781=CARTESIAN_POINT('Ctrl Pts',(1.54440491149498,1.,0.914375919026456));
#21782=CARTESIAN_POINT('Ctrl Pts',(1.52984849887993,1.,0.905967409625651));
#21783=CARTESIAN_POINT('Ctrl Pts',(1.51805569590094,1.,0.899185047483511));
#21784=CARTESIAN_POINT('Ctrl Pts',(1.50980486806688,1.,0.894452006964544));
#21785=CARTESIAN_POINT('Ctrl Pts',(1.5055822144029,1.,0.892032620296856));
#21786=CARTESIAN_POINT('',(1.81978687191668,0.,1.23627494547115));
#21787=CARTESIAN_POINT('Origin',(1.73811241238545,0.,1.34869019493419));
#21788=CARTESIAN_POINT('',(1.73811241238545,1.,1.34869019493419));
#21789=CARTESIAN_POINT('',(1.81978687191668,1.,1.23627494547115));
#21790=CARTESIAN_POINT('',(1.73811241238545,0.,1.34869019493419));
#21791=CARTESIAN_POINT('Ctrl Pts',(1.31362392696032,-1.,1.15624053661742));
#21792=CARTESIAN_POINT('Ctrl Pts',(1.31362392696032,1.,1.15624053661742));
#21793=CARTESIAN_POINT('Ctrl Pts',(1.31722977216397,-1.,1.15950888730809));
#21794=CARTESIAN_POINT('Ctrl Pts',(1.31722977216397,1.,1.15950888730809));
#21795=CARTESIAN_POINT('Ctrl Pts',(1.32428080721772,-1.,1.16589330093588));
#21796=CARTESIAN_POINT('Ctrl Pts',(1.32428080721772,1.,1.16589330093588));
#21797=CARTESIAN_POINT('Ctrl Pts',(1.33437539347008,-1.,1.17501305789857));
#21798=CARTESIAN_POINT('Ctrl Pts',(1.33437539347008,1.,1.17501305789857));
#21799=CARTESIAN_POINT('Ctrl Pts',(1.34687054001093,-1.,1.18625865667441));
#21800=CARTESIAN_POINT('Ctrl Pts',(1.34687054001093,1.,1.18625865667441));
#21801=CARTESIAN_POINT('Ctrl Pts',(1.36088705043885,-1.,1.1987959077932));
#21802=CARTESIAN_POINT('Ctrl Pts',(1.36088705043885,1.,1.1987959077932));
#21803=CARTESIAN_POINT('Ctrl Pts',(1.37331915607905,-1.,1.20982812925645));
#21804=CARTESIAN_POINT('Ctrl Pts',(1.37331915607905,1.,1.20982812925645));
#21805=CARTESIAN_POINT('Ctrl Pts',(1.38420564527715,-1.,1.21938737280852));
#21806=CARTESIAN_POINT('Ctrl Pts',(1.38420564527715,1.,1.21938737280852));
#21807=CARTESIAN_POINT('Ctrl Pts',(1.39361389568796,-1.,1.22752961899387));
#21808=CARTESIAN_POINT('Ctrl Pts',(1.39361389568796,1.,1.22752961899387));
#21809=CARTESIAN_POINT('Ctrl Pts',(1.40164708206106,-1.,1.23434087290423));
#21810=CARTESIAN_POINT('Ctrl Pts',(1.40164708206106,1.,1.23434087290423));
#21811=CARTESIAN_POINT('Ctrl Pts',(1.40845295531283,-1.,1.23994455029534));
#21812=CARTESIAN_POINT('Ctrl Pts',(1.40845295531283,1.,1.23994455029534));
#21813=CARTESIAN_POINT('Ctrl Pts',(1.41422913175179,-1.,1.24450600513056));
#21814=CARTESIAN_POINT('Ctrl Pts',(1.41422913175179,1.,1.24450600513056));
#21815=CARTESIAN_POINT('Ctrl Pts',(1.41923722596025,-1.,1.24824430986571));
#21816=CARTESIAN_POINT('Ctrl Pts',(1.41923722596025,1.,1.24824430986571));
#21817=CARTESIAN_POINT('Ctrl Pts',(1.42378102115575,-1.,1.2514145557001));
#21818=CARTESIAN_POINT('Ctrl Pts',(1.42378102115575,1.,1.2514145557001));
#21819=CARTESIAN_POINT('Ctrl Pts',(1.42815938799387,-1.,1.25426945222639));
#21820=CARTESIAN_POINT('Ctrl Pts',(1.42815938799387,1.,1.25426945222639));
#21821=CARTESIAN_POINT('Ctrl Pts',(1.43262645609691,-1.,1.25702687965755));
#21822=CARTESIAN_POINT('Ctrl Pts',(1.43262645609691,1.,1.25702687965755));
#21823=CARTESIAN_POINT('Ctrl Pts',(1.43734919180847,-1.,1.25983531012005));
#21824=CARTESIAN_POINT('Ctrl Pts',(1.43734919180847,1.,1.25983531012005));
#21825=CARTESIAN_POINT('Ctrl Pts',(1.44236470511303,-1.,1.26273903323859));
#21826=CARTESIAN_POINT('Ctrl Pts',(1.44236470511303,1.,1.26273903323859));
#21827=CARTESIAN_POINT('Ctrl Pts',(1.44761985001662,-1.,1.26570925118868));
#21828=CARTESIAN_POINT('Ctrl Pts',(1.44761985001662,1.,1.26570925118868));
#21829=CARTESIAN_POINT('Ctrl Pts',(1.45301422764247,-1.,1.2686778680489));
#21830=CARTESIAN_POINT('Ctrl Pts',(1.45301422764247,1.,1.2686778680489));
#21831=CARTESIAN_POINT('Ctrl Pts',(1.45843906294697,-1.,1.27156805265289));
#21832=CARTESIAN_POINT('Ctrl Pts',(1.45843906294697,1.,1.27156805265289));
#21833=CARTESIAN_POINT('Ctrl Pts',(1.46382431332476,-1.,1.27433119897822));
#21834=CARTESIAN_POINT('Ctrl Pts',(1.46382431332476,1.,1.27433119897822));
#21835=CARTESIAN_POINT('Ctrl Pts',(1.46916035917133,-1.,1.2769641483109));
#21836=CARTESIAN_POINT('Ctrl Pts',(1.46916035917133,1.,1.2769641483109));
#21837=CARTESIAN_POINT('Ctrl Pts',(1.4744717526707,-1.,1.2794891824849));
#21838=CARTESIAN_POINT('Ctrl Pts',(1.4744717526707,1.,1.2794891824849));
#21839=CARTESIAN_POINT('Ctrl Pts',(1.47980070347095,-1.,1.28194158939517));
#21840=CARTESIAN_POINT('Ctrl Pts',(1.47980070347095,1.,1.28194158939517));
#21841=CARTESIAN_POINT('Ctrl Pts',(1.4851881711891,-1.,1.28435533880201));
#21842=CARTESIAN_POINT('Ctrl Pts',(1.4851881711891,1.,1.28435533880201));
#21843=CARTESIAN_POINT('Ctrl Pts',(1.4906522831278,-1.,1.2867467611644));
#21844=CARTESIAN_POINT('Ctrl Pts',(1.4906522831278,1.,1.2867467611644));
#21845=CARTESIAN_POINT('Ctrl Pts',(1.49618896881754,-1.,1.28911506584254));
#21846=CARTESIAN_POINT('Ctrl Pts',(1.49618896881754,1.,1.28911506584254));
#21847=CARTESIAN_POINT('Ctrl Pts',(1.50178230149776,-1.,1.29145022885181));
#21848=CARTESIAN_POINT('Ctrl Pts',(1.50178230149776,1.,1.29145022885181));
#21849=CARTESIAN_POINT('Ctrl Pts',(1.50741159078365,-1.,1.29373841372842));
#21850=CARTESIAN_POINT('Ctrl Pts',(1.50741159078365,1.,1.29373841372842));
#21851=CARTESIAN_POINT('Ctrl Pts',(1.51305994241402,-1.,1.29596850710509));
#21852=CARTESIAN_POINT('Ctrl Pts',(1.51305994241402,1.,1.29596850710509));
#21853=CARTESIAN_POINT('Ctrl Pts',(1.51872184912724,-1.,1.29813791800747));
#21854=CARTESIAN_POINT('Ctrl Pts',(1.51872184912724,1.,1.29813791800747));
#21855=CARTESIAN_POINT('Ctrl Pts',(1.52439957861062,-1.,1.30024984366328));
#21856=CARTESIAN_POINT('Ctrl Pts',(1.52439957861062,1.,1.30024984366328));
#21857=CARTESIAN_POINT('Ctrl Pts',(1.53009970283891,-1.,1.30231064395568));
#21858=CARTESIAN_POINT('Ctrl Pts',(1.53009970283891,1.,1.30231064395568));
#21859=CARTESIAN_POINT('Ctrl Pts',(1.53582981268977,-1.,1.30432735639489));
#21860=CARTESIAN_POINT('Ctrl Pts',(1.53582981268977,1.,1.30432735639489));
#21861=CARTESIAN_POINT('Ctrl Pts',(1.54159462645432,-1.,1.30630475189556));
#21862=CARTESIAN_POINT('Ctrl Pts',(1.54159462645432,1.,1.30630475189556));
#21863=CARTESIAN_POINT('Ctrl Pts',(1.54739413957185,-1.,1.30824393907473));
#21864=CARTESIAN_POINT('Ctrl Pts',(1.54739413957185,1.,1.30824393907473));
#21865=CARTESIAN_POINT('Ctrl Pts',(1.55322568759481,-1.,1.31014393684222));
#21866=CARTESIAN_POINT('Ctrl Pts',(1.55322568759481,1.,1.31014393684222));
#21867=CARTESIAN_POINT('Ctrl Pts',(1.55908521254821,-1.,1.31200264341696));
#21868=CARTESIAN_POINT('Ctrl Pts',(1.55908521254821,1.,1.31200264341696));
#21869=CARTESIAN_POINT('Ctrl Pts',(1.56496872402353,-1.,1.31381795281002));
#21870=CARTESIAN_POINT('Ctrl Pts',(1.56496872402353,1.,1.31381795281002));
#21871=CARTESIAN_POINT('Ctrl Pts',(1.57087397835723,-1.,1.31558903860016));
#21872=CARTESIAN_POINT('Ctrl Pts',(1.57087397835723,1.,1.31558903860016));
#21873=CARTESIAN_POINT('Ctrl Pts',(1.5768005650559,-1.,1.31731642317187));
#21874=CARTESIAN_POINT('Ctrl Pts',(1.5768005650559,1.,1.31731642317187));
#21875=CARTESIAN_POINT('Ctrl Pts',(1.58274907898834,-1.,1.31900135021432));
#21876=CARTESIAN_POINT('Ctrl Pts',(1.58274907898834,1.,1.31900135021432));
#21877=CARTESIAN_POINT('Ctrl Pts',(1.58872057258245,-1.,1.32064537110892));
#21878=CARTESIAN_POINT('Ctrl Pts',(1.58872057258245,1.,1.32064537110892));
#21879=CARTESIAN_POINT('Ctrl Pts',(1.59471591079403,-1.,1.32224985747682));
#21880=CARTESIAN_POINT('Ctrl Pts',(1.59471591079403,1.,1.32224985747682));
#21881=CARTESIAN_POINT('Ctrl Pts',(1.60073511858687,-1.,1.32381550858256));
#21882=CARTESIAN_POINT('Ctrl Pts',(1.60073511858687,1.,1.32381550858256));
#21883=CARTESIAN_POINT('Ctrl Pts',(1.60677758290954,-1.,1.32534250785782));
#21884=CARTESIAN_POINT('Ctrl Pts',(1.60677758290954,1.,1.32534250785782));
#21885=CARTESIAN_POINT('Ctrl Pts',(1.6128423401575,-1.,1.32683074483356));
#21886=CARTESIAN_POINT('Ctrl Pts',(1.6128423401575,1.,1.32683074483356));
#21887=CARTESIAN_POINT('Ctrl Pts',(1.61892832270724,-1.,1.32828000610449));
#21888=CARTESIAN_POINT('Ctrl Pts',(1.61892832270724,1.,1.32828000610449));
#21889=CARTESIAN_POINT('Ctrl Pts',(1.62503464209797,-1.,1.3296901950568));
#21890=CARTESIAN_POINT('Ctrl Pts',(1.62503464209797,1.,1.3296901950568));
#21891=CARTESIAN_POINT('Ctrl Pts',(1.63116079730923,-1.,1.33106149345645));
#21892=CARTESIAN_POINT('Ctrl Pts',(1.63116079730923,1.,1.33106149345645));
#21893=CARTESIAN_POINT('Ctrl Pts',(1.63730653475089,-1.,1.33239425103724));
#21894=CARTESIAN_POINT('Ctrl Pts',(1.63730653475089,1.,1.33239425103724));
#21895=CARTESIAN_POINT('Ctrl Pts',(1.6434717485603,-1.,1.33368890676572));
#21896=CARTESIAN_POINT('Ctrl Pts',(1.6434717485603,1.,1.33368890676572));
#21897=CARTESIAN_POINT('Ctrl Pts',(1.6496563728683,-1.,1.33494590467993));
#21898=CARTESIAN_POINT('Ctrl Pts',(1.6496563728683,1.,1.33494590467993));
#21899=CARTESIAN_POINT('Ctrl Pts',(1.65586025952593,-1.,1.33616559745172));
#21900=CARTESIAN_POINT('Ctrl Pts',(1.65586025952593,1.,1.33616559745172));
#21901=CARTESIAN_POINT('Ctrl Pts',(1.66208312541983,-1.,1.33734820885262));
#21902=CARTESIAN_POINT('Ctrl Pts',(1.66208312541983,1.,1.33734820885262));
#21903=CARTESIAN_POINT('Ctrl Pts',(1.66832460783989,-1.,1.33849388654388));
#21904=CARTESIAN_POINT('Ctrl Pts',(1.66832460783989,1.,1.33849388654388));
#21905=CARTESIAN_POINT('Ctrl Pts',(1.67458429426086,-1.,1.3396027347034));
#21906=CARTESIAN_POINT('Ctrl Pts',(1.67458429426086,1.,1.3396027347034));
#21907=CARTESIAN_POINT('Ctrl Pts',(1.68086176030362,-1.,1.34067485185203));
#21908=CARTESIAN_POINT('Ctrl Pts',(1.68086176030362,1.,1.34067485185203));
#21909=CARTESIAN_POINT('Ctrl Pts',(1.68715660868764,-1.,1.341710374848));
#21910=CARTESIAN_POINT('Ctrl Pts',(1.68715660868764,1.,1.341710374848));
#21911=CARTESIAN_POINT('Ctrl Pts',(1.6934684849687,-1.,1.34270948206319));
#21912=CARTESIAN_POINT('Ctrl Pts',(1.6934684849687,1.,1.34270948206319));
#21913=CARTESIAN_POINT('Ctrl Pts',(1.69979707754427,-1.,1.34367237124483));
#21914=CARTESIAN_POINT('Ctrl Pts',(1.69979707754427,1.,1.34367237124483));
#21915=CARTESIAN_POINT('Ctrl Pts',(1.70614212266738,-1.,1.34459924533831));
#21916=CARTESIAN_POINT('Ctrl Pts',(1.70614212266738,1.,1.34459924533831));
#21917=CARTESIAN_POINT('Ctrl Pts',(1.71250340686822,-1.,1.34549029589416));
#21918=CARTESIAN_POINT('Ctrl Pts',(1.71250340686822,1.,1.34549029589416));
#21919=CARTESIAN_POINT('Ctrl Pts',(1.7188807715049,-1.,1.34634568653227));
#21920=CARTESIAN_POINT('Ctrl Pts',(1.7188807715049,1.,1.34634568653227));
#21921=CARTESIAN_POINT('Ctrl Pts',(1.72527410680674,-1.,1.34716554819527));
#21922=CARTESIAN_POINT('Ctrl Pts',(1.72527410680674,1.,1.34716554819527));
#21923=CARTESIAN_POINT('Ctrl Pts',(1.7304014965394,-1.,1.34779309152035));
#21924=CARTESIAN_POINT('Ctrl Pts',(1.7304014965394,1.,1.34779309152035));
#21925=CARTESIAN_POINT('Ctrl Pts',(1.73425417885907,-1.,1.34824783112887));
#21926=CARTESIAN_POINT('Ctrl Pts',(1.73425417885907,1.,1.34824783112887));
#21927=CARTESIAN_POINT('Ctrl Pts',(1.73682580585691,-1.,1.34854391898045));
#21928=CARTESIAN_POINT('Ctrl Pts',(1.73682580585691,1.,1.34854391898045));
#21929=CARTESIAN_POINT('Ctrl Pts',(1.73811241238545,-1.,1.34869019493419));
#21930=CARTESIAN_POINT('Ctrl Pts',(1.73811241238545,1.,1.34869019493419));
#21931=CARTESIAN_POINT('',(1.31362392696032,1.,1.15624053661742));
#21932=CARTESIAN_POINT('Ctrl Pts',(1.31362392696032,1.,1.15624053661742));
#21933=CARTESIAN_POINT('Ctrl Pts',(1.31722977216397,1.,1.15950888730809));
#21934=CARTESIAN_POINT('Ctrl Pts',(1.32428080721772,1.,1.16589330093588));
#21935=CARTESIAN_POINT('Ctrl Pts',(1.33437539347008,1.,1.17501305789857));
#21936=CARTESIAN_POINT('Ctrl Pts',(1.34687054001093,1.,1.18625865667441));
#21937=CARTESIAN_POINT('Ctrl Pts',(1.36088705043885,1.,1.1987959077932));
#21938=CARTESIAN_POINT('Ctrl Pts',(1.37331915607905,1.,1.20982812925645));
#21939=CARTESIAN_POINT('Ctrl Pts',(1.38420564527715,1.,1.21938737280852));
#21940=CARTESIAN_POINT('Ctrl Pts',(1.39361389568796,1.,1.22752961899387));
#21941=CARTESIAN_POINT('Ctrl Pts',(1.40164708206106,1.,1.23434087290423));
#21942=CARTESIAN_POINT('Ctrl Pts',(1.40845295531283,1.,1.23994455029534));
#21943=CARTESIAN_POINT('Ctrl Pts',(1.41422913175179,1.,1.24450600513056));
#21944=CARTESIAN_POINT('Ctrl Pts',(1.41923722596025,1.,1.24824430986571));
#21945=CARTESIAN_POINT('Ctrl Pts',(1.42378102115575,1.,1.2514145557001));
#21946=CARTESIAN_POINT('Ctrl Pts',(1.42815938799387,1.,1.25426945222639));
#21947=CARTESIAN_POINT('Ctrl Pts',(1.43262645609691,1.,1.25702687965755));
#21948=CARTESIAN_POINT('Ctrl Pts',(1.43734919180847,1.,1.25983531012005));
#21949=CARTESIAN_POINT('Ctrl Pts',(1.44236470511303,1.,1.26273903323859));
#21950=CARTESIAN_POINT('Ctrl Pts',(1.44761985001662,1.,1.26570925118868));
#21951=CARTESIAN_POINT('Ctrl Pts',(1.45301422764247,1.,1.2686778680489));
#21952=CARTESIAN_POINT('Ctrl Pts',(1.45843906294697,1.,1.27156805265289));
#21953=CARTESIAN_POINT('Ctrl Pts',(1.46382431332476,1.,1.27433119897822));
#21954=CARTESIAN_POINT('Ctrl Pts',(1.46916035917133,1.,1.2769641483109));
#21955=CARTESIAN_POINT('Ctrl Pts',(1.4744717526707,1.,1.2794891824849));
#21956=CARTESIAN_POINT('Ctrl Pts',(1.47980070347095,1.,1.28194158939517));
#21957=CARTESIAN_POINT('Ctrl Pts',(1.4851881711891,1.,1.28435533880201));
#21958=CARTESIAN_POINT('Ctrl Pts',(1.4906522831278,1.,1.2867467611644));
#21959=CARTESIAN_POINT('Ctrl Pts',(1.49618896881754,1.,1.28911506584254));
#21960=CARTESIAN_POINT('Ctrl Pts',(1.50178230149776,1.,1.29145022885181));
#21961=CARTESIAN_POINT('Ctrl Pts',(1.50741159078365,1.,1.29373841372842));
#21962=CARTESIAN_POINT('Ctrl Pts',(1.51305994241402,1.,1.29596850710509));
#21963=CARTESIAN_POINT('Ctrl Pts',(1.51872184912724,1.,1.29813791800747));
#21964=CARTESIAN_POINT('Ctrl Pts',(1.52439957861062,1.,1.30024984366328));
#21965=CARTESIAN_POINT('Ctrl Pts',(1.53009970283891,1.,1.30231064395568));
#21966=CARTESIAN_POINT('Ctrl Pts',(1.53582981268977,1.,1.30432735639489));
#21967=CARTESIAN_POINT('Ctrl Pts',(1.54159462645432,1.,1.30630475189556));
#21968=CARTESIAN_POINT('Ctrl Pts',(1.54739413957185,1.,1.30824393907473));
#21969=CARTESIAN_POINT('Ctrl Pts',(1.55322568759481,1.,1.31014393684222));
#21970=CARTESIAN_POINT('Ctrl Pts',(1.55908521254821,1.,1.31200264341696));
#21971=CARTESIAN_POINT('Ctrl Pts',(1.56496872402353,1.,1.31381795281002));
#21972=CARTESIAN_POINT('Ctrl Pts',(1.57087397835723,1.,1.31558903860016));
#21973=CARTESIAN_POINT('Ctrl Pts',(1.5768005650559,1.,1.31731642317187));
#21974=CARTESIAN_POINT('Ctrl Pts',(1.58274907898834,1.,1.31900135021432));
#21975=CARTESIAN_POINT('Ctrl Pts',(1.58872057258245,1.,1.32064537110892));
#21976=CARTESIAN_POINT('Ctrl Pts',(1.59471591079403,1.,1.32224985747682));
#21977=CARTESIAN_POINT('Ctrl Pts',(1.60073511858687,1.,1.32381550858256));
#21978=CARTESIAN_POINT('Ctrl Pts',(1.60677758290954,1.,1.32534250785782));
#21979=CARTESIAN_POINT('Ctrl Pts',(1.6128423401575,1.,1.32683074483356));
#21980=CARTESIAN_POINT('Ctrl Pts',(1.61892832270724,1.,1.32828000610449));
#21981=CARTESIAN_POINT('Ctrl Pts',(1.62503464209797,1.,1.3296901950568));
#21982=CARTESIAN_POINT('Ctrl Pts',(1.63116079730923,1.,1.33106149345645));
#21983=CARTESIAN_POINT('Ctrl Pts',(1.63730653475089,1.,1.33239425103724));
#21984=CARTESIAN_POINT('Ctrl Pts',(1.6434717485603,1.,1.33368890676572));
#21985=CARTESIAN_POINT('Ctrl Pts',(1.6496563728683,1.,1.33494590467993));
#21986=CARTESIAN_POINT('Ctrl Pts',(1.65586025952593,1.,1.33616559745172));
#21987=CARTESIAN_POINT('Ctrl Pts',(1.66208312541983,1.,1.33734820885262));
#21988=CARTESIAN_POINT('Ctrl Pts',(1.66832460783989,1.,1.33849388654388));
#21989=CARTESIAN_POINT('Ctrl Pts',(1.67458429426086,1.,1.3396027347034));
#21990=CARTESIAN_POINT('Ctrl Pts',(1.68086176030362,1.,1.34067485185203));
#21991=CARTESIAN_POINT('Ctrl Pts',(1.68715660868764,1.,1.341710374848));
#21992=CARTESIAN_POINT('Ctrl Pts',(1.6934684849687,1.,1.34270948206319));
#21993=CARTESIAN_POINT('Ctrl Pts',(1.69979707754427,1.,1.34367237124483));
#21994=CARTESIAN_POINT('Ctrl Pts',(1.70614212266738,1.,1.34459924533831));
#21995=CARTESIAN_POINT('Ctrl Pts',(1.71250340686822,1.,1.34549029589416));
#21996=CARTESIAN_POINT('Ctrl Pts',(1.7188807715049,1.,1.34634568653227));
#21997=CARTESIAN_POINT('Ctrl Pts',(1.72527410680674,1.,1.34716554819527));
#21998=CARTESIAN_POINT('Ctrl Pts',(1.7304014965394,1.,1.34779309152035));
#21999=CARTESIAN_POINT('Ctrl Pts',(1.73425417885907,1.,1.34824783112887));
#22000=CARTESIAN_POINT('Ctrl Pts',(1.73682580585691,1.,1.34854391898045));
#22001=CARTESIAN_POINT('Ctrl Pts',(1.73811241238545,1.,1.34869019493419));
#22002=CARTESIAN_POINT('',(1.31362392696032,0.,1.15624053661742));
#22003=CARTESIAN_POINT('Origin',(0.,0.,0.));
#22004=CARTESIAN_POINT('',(1.15624053661742,1.,1.31362392696033));
#22005=CARTESIAN_POINT('Origin',(0.,1.,0.));
#22006=CARTESIAN_POINT('',(1.15624053661742,0.,1.31362392696032));
#22007=CARTESIAN_POINT('Ctrl Pts',(1.34869019493419,-1.,1.73811241238545));
#22008=CARTESIAN_POINT('Ctrl Pts',(1.34869019493419,1.,1.73811241238545));
#22009=CARTESIAN_POINT('Ctrl Pts',(1.34854391898145,-1.,1.73682580585819));
#22010=CARTESIAN_POINT('Ctrl Pts',(1.34854391898145,1.,1.73682580585819));
#22011=CARTESIAN_POINT('Ctrl Pts',(1.34824783113158,-1.,1.73425417886255));
#22012=CARTESIAN_POINT('Ctrl Pts',(1.34824783113158,1.,1.73425417886255));
#22013=CARTESIAN_POINT('Ctrl Pts',(1.3477930915247,-1.,1.73040149654497));
#22014=CARTESIAN_POINT('Ctrl Pts',(1.3477930915247,1.,1.73040149654497));
#22015=CARTESIAN_POINT('Ctrl Pts',(1.34716554820013,-1.,1.72527410681298));
#22016=CARTESIAN_POINT('Ctrl Pts',(1.34716554820013,1.,1.72527410681298));
#22017=CARTESIAN_POINT('Ctrl Pts',(1.34634568653586,-1.,1.7188807715095));
#22018=CARTESIAN_POINT('Ctrl Pts',(1.34634568653586,1.,1.7188807715095));
#22019=CARTESIAN_POINT('Ctrl Pts',(1.34549029589563,-1.,1.71250340687011));
#22020=CARTESIAN_POINT('Ctrl Pts',(1.34549029589563,1.,1.71250340687011));
#22021=CARTESIAN_POINT('Ctrl Pts',(1.34459924533783,-1.,1.70614212266676));
#22022=CARTESIAN_POINT('Ctrl Pts',(1.34459924533783,1.,1.70614212266676));
#22023=CARTESIAN_POINT('Ctrl Pts',(1.34367237124322,-1.,1.69979707754221));
#22024=CARTESIAN_POINT('Ctrl Pts',(1.34367237124322,1.,1.69979707754221));
#22025=CARTESIAN_POINT('Ctrl Pts',(1.34270948206139,-1.,1.6934684849664));
#22026=CARTESIAN_POINT('Ctrl Pts',(1.34270948206139,1.,1.6934684849664));
#22027=CARTESIAN_POINT('Ctrl Pts',(1.34171037484673,-1.,1.68715660868602));
#22028=CARTESIAN_POINT('Ctrl Pts',(1.34171037484673,1.,1.68715660868602));
#22029=CARTESIAN_POINT('Ctrl Pts',(1.3406748518516,-1.,1.68086176030308));
#22030=CARTESIAN_POINT('Ctrl Pts',(1.3406748518516,1.,1.68086176030308));
#22031=CARTESIAN_POINT('Ctrl Pts',(1.33960273470372,-1.,1.67458429426126));
#22032=CARTESIAN_POINT('Ctrl Pts',(1.33960273470372,1.,1.67458429426126));
#22033=CARTESIAN_POINT('Ctrl Pts',(1.33849388654458,-1.,1.66832460784078));
#22034=CARTESIAN_POINT('Ctrl Pts',(1.33849388654458,1.,1.66832460784078));
#22035=CARTESIAN_POINT('Ctrl Pts',(1.33734820885331,-1.,1.66208312542073));
#22036=CARTESIAN_POINT('Ctrl Pts',(1.33734820885331,1.,1.66208312542073));
#22037=CARTESIAN_POINT('Ctrl Pts',(1.33616559745217,-1.,1.65586025952651));
#22038=CARTESIAN_POINT('Ctrl Pts',(1.33616559745217,1.,1.65586025952651));
#22039=CARTESIAN_POINT('Ctrl Pts',(1.33494590468003,-1.,1.64965637286843));
#22040=CARTESIAN_POINT('Ctrl Pts',(1.33494590468003,1.,1.64965637286843));
#22041=CARTESIAN_POINT('Ctrl Pts',(1.33368890676554,-1.,1.64347174856007));
#22042=CARTESIAN_POINT('Ctrl Pts',(1.33368890676554,1.,1.64347174856007));
#22043=CARTESIAN_POINT('Ctrl Pts',(1.33239425103694,-1.,1.6373065347505));
#22044=CARTESIAN_POINT('Ctrl Pts',(1.33239425103694,1.,1.6373065347505));
#22045=CARTESIAN_POINT('Ctrl Pts',(1.33106149345618,-1.,1.63116079730887));
#22046=CARTESIAN_POINT('Ctrl Pts',(1.33106149345618,1.,1.63116079730887));
#22047=CARTESIAN_POINT('Ctrl Pts',(1.32969019505665,-1.,1.62503464209777));
#22048=CARTESIAN_POINT('Ctrl Pts',(1.32969019505665,1.,1.62503464209777));
#22049=CARTESIAN_POINT('Ctrl Pts',(1.32828000610448,-1.,1.61892832270723));
#22050=CARTESIAN_POINT('Ctrl Pts',(1.32828000610448,1.,1.61892832270723));
#22051=CARTESIAN_POINT('Ctrl Pts',(1.32683074483365,-1.,1.61284234015762));
#22052=CARTESIAN_POINT('Ctrl Pts',(1.32683074483365,1.,1.61284234015762));
#22053=CARTESIAN_POINT('Ctrl Pts',(1.32534250785794,-1.,1.6067775829097));
#22054=CARTESIAN_POINT('Ctrl Pts',(1.32534250785794,1.,1.6067775829097));
#22055=CARTESIAN_POINT('Ctrl Pts',(1.32381550858266,-1.,1.600735118587));
#22056=CARTESIAN_POINT('Ctrl Pts',(1.32381550858266,1.,1.600735118587));
#22057=CARTESIAN_POINT('Ctrl Pts',(1.32224985747686,-1.,1.59471591079408));
#22058=CARTESIAN_POINT('Ctrl Pts',(1.32224985747686,1.,1.59471591079408));
#22059=CARTESIAN_POINT('Ctrl Pts',(1.32064537110891,-1.,1.58872057258244));
#22060=CARTESIAN_POINT('Ctrl Pts',(1.32064537110891,1.,1.58872057258244));
#22061=CARTESIAN_POINT('Ctrl Pts',(1.31900135021428,-1.,1.58274907898829));
#22062=CARTESIAN_POINT('Ctrl Pts',(1.31900135021428,1.,1.58274907898829));
#22063=CARTESIAN_POINT('Ctrl Pts',(1.31731642317183,-1.,1.57680056505585));
#22064=CARTESIAN_POINT('Ctrl Pts',(1.31731642317183,1.,1.57680056505585));
#22065=CARTESIAN_POINT('Ctrl Pts',(1.31558903860015,-1.,1.57087397835721));
#22066=CARTESIAN_POINT('Ctrl Pts',(1.31558903860015,1.,1.57087397835721));
#22067=CARTESIAN_POINT('Ctrl Pts',(1.31381795281002,-1.,1.56496872402352));
#22068=CARTESIAN_POINT('Ctrl Pts',(1.31381795281002,1.,1.56496872402352));
#22069=CARTESIAN_POINT('Ctrl Pts',(1.31200264341696,-1.,1.55908521254822));
#22070=CARTESIAN_POINT('Ctrl Pts',(1.31200264341696,1.,1.55908521254822));
#22071=CARTESIAN_POINT('Ctrl Pts',(1.31014393684221,-1.,1.55322568759481));
#22072=CARTESIAN_POINT('Ctrl Pts',(1.31014393684221,1.,1.55322568759481));
#22073=CARTESIAN_POINT('Ctrl Pts',(1.30824393907471,-1.,1.54739413957183));
#22074=CARTESIAN_POINT('Ctrl Pts',(1.30824393907471,1.,1.54739413957183));
#22075=CARTESIAN_POINT('Ctrl Pts',(1.30630475189553,-1.,1.54159462645428));
#22076=CARTESIAN_POINT('Ctrl Pts',(1.30630475189553,1.,1.54159462645428));
#22077=CARTESIAN_POINT('Ctrl Pts',(1.30432735639487,-1.,1.53582981268976));
#22078=CARTESIAN_POINT('Ctrl Pts',(1.30432735639487,1.,1.53582981268976));
#22079=CARTESIAN_POINT('Ctrl Pts',(1.3023106439557,-1.,1.53009970283893));
#22080=CARTESIAN_POINT('Ctrl Pts',(1.3023106439557,1.,1.53009970283893));
#22081=CARTESIAN_POINT('Ctrl Pts',(1.30024984366334,-1.,1.5243995786107));
#22082=CARTESIAN_POINT('Ctrl Pts',(1.30024984366334,1.,1.5243995786107));
#22083=CARTESIAN_POINT('Ctrl Pts',(1.29813791800757,-1.,1.51872184912735));
#22084=CARTESIAN_POINT('Ctrl Pts',(1.29813791800757,1.,1.51872184912735));
#22085=CARTESIAN_POINT('Ctrl Pts',(1.29596850710518,-1.,1.51305994241412));
#22086=CARTESIAN_POINT('Ctrl Pts',(1.29596850710518,1.,1.51305994241412));
#22087=CARTESIAN_POINT('Ctrl Pts',(1.29373841372843,-1.,1.50741159078367));
#22088=CARTESIAN_POINT('Ctrl Pts',(1.29373841372843,1.,1.50741159078367));
#22089=CARTESIAN_POINT('Ctrl Pts',(1.29145022885171,-1.,1.50178230149764));
#22090=CARTESIAN_POINT('Ctrl Pts',(1.29145022885171,1.,1.50178230149764));
#22091=CARTESIAN_POINT('Ctrl Pts',(1.28911506584232,-1.,1.49618896881729));
#22092=CARTESIAN_POINT('Ctrl Pts',(1.28911506584232,1.,1.49618896881729));
#22093=CARTESIAN_POINT('Ctrl Pts',(1.28674676116415,-1.,1.4906522831275));
#22094=CARTESIAN_POINT('Ctrl Pts',(1.28674676116415,1.,1.4906522831275));
#22095=CARTESIAN_POINT('Ctrl Pts',(1.28435533880184,-1.,1.48518817118891));
#22096=CARTESIAN_POINT('Ctrl Pts',(1.28435533880184,1.,1.48518817118891));
#22097=CARTESIAN_POINT('Ctrl Pts',(1.28194158939522,-1.,1.47980070347102));
#22098=CARTESIAN_POINT('Ctrl Pts',(1.28194158939522,1.,1.47980070347102));
#22099=CARTESIAN_POINT('Ctrl Pts',(1.27948918248524,-1.,1.4744717526711));
#22100=CARTESIAN_POINT('Ctrl Pts',(1.27948918248524,1.,1.4744717526711));
#22101=CARTESIAN_POINT('Ctrl Pts',(1.27696414831144,-1.,1.46916035917197));
#22102=CARTESIAN_POINT('Ctrl Pts',(1.27696414831144,1.,1.46916035917197));
#22103=CARTESIAN_POINT('Ctrl Pts',(1.27433119897877,-1.,1.4638243133254));
#22104=CARTESIAN_POINT('Ctrl Pts',(1.27433119897877,1.,1.4638243133254));
#22105=CARTESIAN_POINT('Ctrl Pts',(1.27156805265312,-1.,1.45843906294725));
#22106=CARTESIAN_POINT('Ctrl Pts',(1.27156805265312,1.,1.45843906294725));
#22107=CARTESIAN_POINT('Ctrl Pts',(1.26867786804854,-1.,1.45301422764205));
#22108=CARTESIAN_POINT('Ctrl Pts',(1.26867786804854,1.,1.45301422764205));
#22109=CARTESIAN_POINT('Ctrl Pts',(1.26570925118767,-1.,1.44761985001544));
#22110=CARTESIAN_POINT('Ctrl Pts',(1.26570925118767,1.,1.44761985001544));
#22111=CARTESIAN_POINT('Ctrl Pts',(1.26273903323723,-1.,1.44236470511145));
#22112=CARTESIAN_POINT('Ctrl Pts',(1.26273903323723,1.,1.44236470511145));
#22113=CARTESIAN_POINT('Ctrl Pts',(1.25983531011894,-1.,1.43734919180719));
#22114=CARTESIAN_POINT('Ctrl Pts',(1.25983531011894,1.,1.43734919180719));
#22115=CARTESIAN_POINT('Ctrl Pts',(1.25702687965744,-1.,1.43262645609679));
#22116=CARTESIAN_POINT('Ctrl Pts',(1.25702687965744,1.,1.43262645609679));
#22117=CARTESIAN_POINT('Ctrl Pts',(1.25426945222783,-1.,1.42815938799555));
#22118=CARTESIAN_POINT('Ctrl Pts',(1.25426945222783,1.,1.42815938799555));
#22119=CARTESIAN_POINT('Ctrl Pts',(1.25141455570299,-1.,1.42378102115911));
#22120=CARTESIAN_POINT('Ctrl Pts',(1.25141455570299,1.,1.42378102115911));
#22121=CARTESIAN_POINT('Ctrl Pts',(1.24824430986911,-1.,1.41923722596421));
#22122=CARTESIAN_POINT('Ctrl Pts',(1.24824430986911,1.,1.41923722596421));
#22123=CARTESIAN_POINT('Ctrl Pts',(1.24450600513278,-1.,1.41422913175437));
#22124=CARTESIAN_POINT('Ctrl Pts',(1.24450600513278,1.,1.41422913175437));
#22125=CARTESIAN_POINT('Ctrl Pts',(1.23994455029421,-1.,1.40845295531151));
#22126=CARTESIAN_POINT('Ctrl Pts',(1.23994455029421,1.,1.40845295531151));
#22127=CARTESIAN_POINT('Ctrl Pts',(1.23434087289768,-1.,1.40164708205345));
#22128=CARTESIAN_POINT('Ctrl Pts',(1.23434087289768,1.,1.40164708205345));
#22129=CARTESIAN_POINT('Ctrl Pts',(1.22752961898063,-1.,1.39361389567257));
#22130=CARTESIAN_POINT('Ctrl Pts',(1.22752961898063,1.,1.39361389567257));
#22131=CARTESIAN_POINT('Ctrl Pts',(1.21938737278853,-1.,1.38420564525391));
#22132=CARTESIAN_POINT('Ctrl Pts',(1.21938737278853,1.,1.38420564525391));
#22133=CARTESIAN_POINT('Ctrl Pts',(1.20982812923113,-1.,1.37331915604962));
#22134=CARTESIAN_POINT('Ctrl Pts',(1.20982812923113,1.,1.37331915604962));
#22135=CARTESIAN_POINT('Ctrl Pts',(1.1987959077656,-1.,1.36088705040677));
#22136=CARTESIAN_POINT('Ctrl Pts',(1.1987959077656,1.,1.36088705040677));
#22137=CARTESIAN_POINT('Ctrl Pts',(1.18625865664915,-1.,1.34687053998157));
#22138=CARTESIAN_POINT('Ctrl Pts',(1.18625865664915,1.,1.34687053998157));
#22139=CARTESIAN_POINT('Ctrl Pts',(1.17501305787994,-1.,1.33437539344842));
#22140=CARTESIAN_POINT('Ctrl Pts',(1.17501305787994,1.,1.33437539344842));
#22141=CARTESIAN_POINT('Ctrl Pts',(1.16589330092532,-1.,1.32428080720544));
#22142=CARTESIAN_POINT('Ctrl Pts',(1.16589330092532,1.,1.32428080720544));
#22143=CARTESIAN_POINT('Ctrl Pts',(1.15950888730433,-1.,1.3172297721596));
#22144=CARTESIAN_POINT('Ctrl Pts',(1.15950888730433,1.,1.3172297721596));
#22145=CARTESIAN_POINT('Ctrl Pts',(1.15624053661742,-1.,1.31362392696033));
#22146=CARTESIAN_POINT('Ctrl Pts',(1.15624053661742,1.,1.31362392696033));
#22147=CARTESIAN_POINT('',(1.34869019493419,1.,1.73811241238545));
#22148=CARTESIAN_POINT('Ctrl Pts',(1.34869019493419,1.,1.73811241238545));
#22149=CARTESIAN_POINT('Ctrl Pts',(1.34854391898145,1.,1.73682580585819));
#22150=CARTESIAN_POINT('Ctrl Pts',(1.34824783113158,1.,1.73425417886255));
#22151=CARTESIAN_POINT('Ctrl Pts',(1.3477930915247,1.,1.73040149654497));
#22152=CARTESIAN_POINT('Ctrl Pts',(1.34716554820013,1.,1.72527410681298));
#22153=CARTESIAN_POINT('Ctrl Pts',(1.34634568653586,1.,1.7188807715095));
#22154=CARTESIAN_POINT('Ctrl Pts',(1.34549029589563,1.,1.71250340687011));
#22155=CARTESIAN_POINT('Ctrl Pts',(1.34459924533783,1.,1.70614212266676));
#22156=CARTESIAN_POINT('Ctrl Pts',(1.34367237124322,1.,1.69979707754221));
#22157=CARTESIAN_POINT('Ctrl Pts',(1.34270948206139,1.,1.6934684849664));
#22158=CARTESIAN_POINT('Ctrl Pts',(1.34171037484673,1.,1.68715660868602));
#22159=CARTESIAN_POINT('Ctrl Pts',(1.3406748518516,1.,1.68086176030308));
#22160=CARTESIAN_POINT('Ctrl Pts',(1.33960273470372,1.,1.67458429426126));
#22161=CARTESIAN_POINT('Ctrl Pts',(1.33849388654458,1.,1.66832460784078));
#22162=CARTESIAN_POINT('Ctrl Pts',(1.33734820885331,1.,1.66208312542073));
#22163=CARTESIAN_POINT('Ctrl Pts',(1.33616559745217,1.,1.65586025952651));
#22164=CARTESIAN_POINT('Ctrl Pts',(1.33494590468003,1.,1.64965637286843));
#22165=CARTESIAN_POINT('Ctrl Pts',(1.33368890676554,1.,1.64347174856007));
#22166=CARTESIAN_POINT('Ctrl Pts',(1.33239425103694,1.,1.6373065347505));
#22167=CARTESIAN_POINT('Ctrl Pts',(1.33106149345618,1.,1.63116079730887));
#22168=CARTESIAN_POINT('Ctrl Pts',(1.32969019505665,1.,1.62503464209777));
#22169=CARTESIAN_POINT('Ctrl Pts',(1.32828000610448,1.,1.61892832270723));
#22170=CARTESIAN_POINT('Ctrl Pts',(1.32683074483365,1.,1.61284234015762));
#22171=CARTESIAN_POINT('Ctrl Pts',(1.32534250785794,1.,1.6067775829097));
#22172=CARTESIAN_POINT('Ctrl Pts',(1.32381550858266,1.,1.600735118587));
#22173=CARTESIAN_POINT('Ctrl Pts',(1.32224985747686,1.,1.59471591079408));
#22174=CARTESIAN_POINT('Ctrl Pts',(1.32064537110891,1.,1.58872057258244));
#22175=CARTESIAN_POINT('Ctrl Pts',(1.31900135021428,1.,1.58274907898829));
#22176=CARTESIAN_POINT('Ctrl Pts',(1.31731642317183,1.,1.57680056505585));
#22177=CARTESIAN_POINT('Ctrl Pts',(1.31558903860015,1.,1.57087397835721));
#22178=CARTESIAN_POINT('Ctrl Pts',(1.31381795281002,1.,1.56496872402352));
#22179=CARTESIAN_POINT('Ctrl Pts',(1.31200264341696,1.,1.55908521254822));
#22180=CARTESIAN_POINT('Ctrl Pts',(1.31014393684221,1.,1.55322568759481));
#22181=CARTESIAN_POINT('Ctrl Pts',(1.30824393907471,1.,1.54739413957183));
#22182=CARTESIAN_POINT('Ctrl Pts',(1.30630475189553,1.,1.54159462645428));
#22183=CARTESIAN_POINT('Ctrl Pts',(1.30432735639487,1.,1.53582981268976));
#22184=CARTESIAN_POINT('Ctrl Pts',(1.3023106439557,1.,1.53009970283893));
#22185=CARTESIAN_POINT('Ctrl Pts',(1.30024984366334,1.,1.5243995786107));
#22186=CARTESIAN_POINT('Ctrl Pts',(1.29813791800757,1.,1.51872184912735));
#22187=CARTESIAN_POINT('Ctrl Pts',(1.29596850710518,1.,1.51305994241412));
#22188=CARTESIAN_POINT('Ctrl Pts',(1.29373841372843,1.,1.50741159078367));
#22189=CARTESIAN_POINT('Ctrl Pts',(1.29145022885171,1.,1.50178230149764));
#22190=CARTESIAN_POINT('Ctrl Pts',(1.28911506584232,1.,1.49618896881729));
#22191=CARTESIAN_POINT('Ctrl Pts',(1.28674676116415,1.,1.4906522831275));
#22192=CARTESIAN_POINT('Ctrl Pts',(1.28435533880184,1.,1.48518817118891));
#22193=CARTESIAN_POINT('Ctrl Pts',(1.28194158939522,1.,1.47980070347102));
#22194=CARTESIAN_POINT('Ctrl Pts',(1.27948918248524,1.,1.4744717526711));
#22195=CARTESIAN_POINT('Ctrl Pts',(1.27696414831144,1.,1.46916035917197));
#22196=CARTESIAN_POINT('Ctrl Pts',(1.27433119897877,1.,1.4638243133254));
#22197=CARTESIAN_POINT('Ctrl Pts',(1.27156805265312,1.,1.45843906294725));
#22198=CARTESIAN_POINT('Ctrl Pts',(1.26867786804854,1.,1.45301422764205));
#22199=CARTESIAN_POINT('Ctrl Pts',(1.26570925118767,1.,1.44761985001544));
#22200=CARTESIAN_POINT('Ctrl Pts',(1.26273903323723,1.,1.44236470511145));
#22201=CARTESIAN_POINT('Ctrl Pts',(1.25983531011894,1.,1.43734919180719));
#22202=CARTESIAN_POINT('Ctrl Pts',(1.25702687965744,1.,1.43262645609679));
#22203=CARTESIAN_POINT('Ctrl Pts',(1.25426945222783,1.,1.42815938799555));
#22204=CARTESIAN_POINT('Ctrl Pts',(1.25141455570299,1.,1.42378102115911));
#22205=CARTESIAN_POINT('Ctrl Pts',(1.24824430986911,1.,1.41923722596421));
#22206=CARTESIAN_POINT('Ctrl Pts',(1.24450600513278,1.,1.41422913175437));
#22207=CARTESIAN_POINT('Ctrl Pts',(1.23994455029421,1.,1.40845295531151));
#22208=CARTESIAN_POINT('Ctrl Pts',(1.23434087289768,1.,1.40164708205345));
#22209=CARTESIAN_POINT('Ctrl Pts',(1.22752961898063,1.,1.39361389567257));
#22210=CARTESIAN_POINT('Ctrl Pts',(1.21938737278853,1.,1.38420564525391));
#22211=CARTESIAN_POINT('Ctrl Pts',(1.20982812923113,1.,1.37331915604962));
#22212=CARTESIAN_POINT('Ctrl Pts',(1.1987959077656,1.,1.36088705040677));
#22213=CARTESIAN_POINT('Ctrl Pts',(1.18625865664915,1.,1.34687053998157));
#22214=CARTESIAN_POINT('Ctrl Pts',(1.17501305787994,1.,1.33437539344842));
#22215=CARTESIAN_POINT('Ctrl Pts',(1.16589330092532,1.,1.32428080720544));
#22216=CARTESIAN_POINT('Ctrl Pts',(1.15950888730433,1.,1.3172297721596));
#22217=CARTESIAN_POINT('Ctrl Pts',(1.15624053661742,1.,1.31362392696033));
#22218=CARTESIAN_POINT('',(1.34869019493419,0.,1.73811241238545));
#22219=CARTESIAN_POINT('Origin',(1.23627494547115,0.,1.81978687191668));
#22220=CARTESIAN_POINT('',(1.23627494547115,1.,1.81978687191668));
#22221=CARTESIAN_POINT('',(1.34869019493419,1.,1.73811241238545));
#22222=CARTESIAN_POINT('',(1.23627494547115,0.,1.81978687191668));
#22223=CARTESIAN_POINT('Ctrl Pts',(0.892032620296855,-1.,1.5055822144029));
#22224=CARTESIAN_POINT('Ctrl Pts',(0.892032620296855,1.,1.5055822144029));
#22225=CARTESIAN_POINT('Ctrl Pts',(0.894452006967538,-1.,1.50980486807181));
#22226=CARTESIAN_POINT('Ctrl Pts',(0.894452006967538,1.,1.50980486807181));
#22227=CARTESIAN_POINT('Ctrl Pts',(0.89918504749193,-1.,1.51805569591479));
#22228=CARTESIAN_POINT('Ctrl Pts',(0.89918504749193,1.,1.51805569591479));
#22229=CARTESIAN_POINT('Ctrl Pts',(0.905967409640498,-1.,1.52984849890434));
#22230=CARTESIAN_POINT('Ctrl Pts',(0.905967409640498,1.,1.52984849890434));
#22231=CARTESIAN_POINT('Ctrl Pts',(0.914375919046579,-1.,1.54440491152808));
#22232=CARTESIAN_POINT('Ctrl Pts',(0.914375919046579,1.,1.54440491152808));
#22233=CARTESIAN_POINT('Ctrl Pts',(0.923832188966322,-1.,1.56065988582509));
#22234=CARTESIAN_POINT('Ctrl Pts',(0.923832188966322,1.,1.56065988582509));
#22235=CARTESIAN_POINT('Ctrl Pts',(0.932246680128848,-1.,1.57499388385561));
#22236=CARTESIAN_POINT('Ctrl Pts',(0.932246680128848,1.,1.57499388385561));
#22237=CARTESIAN_POINT('Ctrl Pts',(0.939646377909319,-1.,1.58744937489796));
#22238=CARTESIAN_POINT('Ctrl Pts',(0.939646377909319,1.,1.58744937489796));
#22239=CARTESIAN_POINT('Ctrl Pts',(0.946078063325795,-1.,1.59810042045408));
#22240=CARTESIAN_POINT('Ctrl Pts',(0.946078063325795,1.,1.59810042045408));
#22241=CARTESIAN_POINT('Ctrl Pts',(0.951613284361247,-1.,1.60706069897794));
#22242=CARTESIAN_POINT('Ctrl Pts',(0.951613284361247,1.,1.60706069897794));
#22243=CARTESIAN_POINT('Ctrl Pts',(0.956354422921572,-1.,1.61449324337233));
#22244=CARTESIAN_POINT('Ctrl Pts',(0.956354422921572,1.,1.61449324337233));
#22245=CARTESIAN_POINT('Ctrl Pts',(0.960438326099958,-1.,1.62061638139929));
#22246=CARTESIAN_POINT('Ctrl Pts',(0.960438326099958,1.,1.62061638139929));
#22247=CARTESIAN_POINT('Ctrl Pts',(0.964046107037821,-1.,1.6257193066974));
#22248=CARTESIAN_POINT('Ctrl Pts',(0.964046107037821,1.,1.6257193066974));
#22249=CARTESIAN_POINT('Ctrl Pts',(0.967387853228041,-1.,1.63013849959083));
#22250=CARTESIAN_POINT('Ctrl Pts',(0.967387853228041,1.,1.63013849959083));
#22251=CARTESIAN_POINT('Ctrl Pts',(0.970669715996356,-1.,1.63420665729609));
#22252=CARTESIAN_POINT('Ctrl Pts',(0.970669715996356,1.,1.63420665729609));
#22253=CARTESIAN_POINT('Ctrl Pts',(0.974066058287501,-1.,1.63820952658157));
#22254=CARTESIAN_POINT('Ctrl Pts',(0.974066058287501,1.,1.63820952658157));
#22255=CARTESIAN_POINT('Ctrl Pts',(0.977689794120296,-1.,1.64233990826831));
#22256=CARTESIAN_POINT('Ctrl Pts',(0.977689794120296,1.,1.64233990826831));
#22257=CARTESIAN_POINT('Ctrl Pts',(0.981562530940574,-1.,1.64665139190834));
#22258=CARTESIAN_POINT('Ctrl Pts',(0.981562530940574,1.,1.64665139190834));
#22259=CARTESIAN_POINT('Ctrl Pts',(0.985642622921626,-1.,1.6511001661277));
#22260=CARTESIAN_POINT('Ctrl Pts',(0.985642622921626,1.,1.6511001661277));
#22261=CARTESIAN_POINT('Ctrl Pts',(0.98985562785445,-1.,1.65559044289746));
#22262=CARTESIAN_POINT('Ctrl Pts',(0.98985562785445,1.,1.65559044289746));
#22263=CARTESIAN_POINT('Ctrl Pts',(0.994121836661115,-1.,1.66001553809916));
#22264=CARTESIAN_POINT('Ctrl Pts',(0.994121836661115,1.,1.66001553809916));
#22265=CARTESIAN_POINT('Ctrl Pts',(0.998389654952317,-1.,1.66430758030304));
#22266=CARTESIAN_POINT('Ctrl Pts',(0.998389654952317,1.,1.66430758030304));
#22267=CARTESIAN_POINT('Ctrl Pts',(1.00265091003682,-1.,1.66846059277231));
#22268=CARTESIAN_POINT('Ctrl Pts',(1.00265091003682,1.,1.66846059277231));
#22269=CARTESIAN_POINT('Ctrl Pts',(1.00692206696387,-1.,1.67250335383248));
#22270=CARTESIAN_POINT('Ctrl Pts',(1.00692206696387,1.,1.67250335383248));
#22271=CARTESIAN_POINT('Ctrl Pts',(1.01123236493507,-1.,1.67648246776457));
#22272=CARTESIAN_POINT('Ctrl Pts',(1.01123236493507,1.,1.67648246776457));
#22273=CARTESIAN_POINT('Ctrl Pts',(1.01561026162786,-1.,1.6804428989482));
#22274=CARTESIAN_POINT('Ctrl Pts',(1.01561026162786,1.,1.6804428989482));
#22275=CARTESIAN_POINT('Ctrl Pts',(1.02006795074222,-1.,1.68440578021739));
#22276=CARTESIAN_POINT('Ctrl Pts',(1.02006795074222,1.,1.68440578021739));
#22277=CARTESIAN_POINT('Ctrl Pts',(1.02460180535272,-1.,1.68836910178475));
#22278=CARTESIAN_POINT('Ctrl Pts',(1.02460180535272,1.,1.68836910178475));
#22279=CARTESIAN_POINT('Ctrl Pts',(1.02919977579155,-1.,1.69231840863471));
#22280=CARTESIAN_POINT('Ctrl Pts',(1.02919977579155,1.,1.69231840863471));
#22281=CARTESIAN_POINT('Ctrl Pts',(1.03384646003587,-1.,1.69623414782769));
#22282=CARTESIAN_POINT('Ctrl Pts',(1.03384646003587,1.,1.69623414782769));
#22283=CARTESIAN_POINT('Ctrl Pts',(1.03852922490782,-1.,1.70010052930951));
#22284=CARTESIAN_POINT('Ctrl Pts',(1.03852922490782,1.,1.70010052930951));
#22285=CARTESIAN_POINT('Ctrl Pts',(1.04324363334546,-1.,1.70391338707969));
#22286=CARTESIAN_POINT('Ctrl Pts',(1.04324363334546,1.,1.70391338707969));
#22287=CARTESIAN_POINT('Ctrl Pts',(1.0479908540499,-1.,1.70767646263641));
#22288=CARTESIAN_POINT('Ctrl Pts',(1.0479908540499,1.,1.70767646263641));
#22289=CARTESIAN_POINT('Ctrl Pts',(1.05277517202853,-1.,1.71139783543986));
#22290=CARTESIAN_POINT('Ctrl Pts',(1.05277517202853,1.,1.71139783543986));
#22291=CARTESIAN_POINT('Ctrl Pts',(1.05760163192481,-1.,1.71508654427022));
#22292=CARTESIAN_POINT('Ctrl Pts',(1.05760163192481,1.,1.71508654427022));
#22293=CARTESIAN_POINT('Ctrl Pts',(1.06247324680649,-1.,1.71874858456908));
#22294=CARTESIAN_POINT('Ctrl Pts',(1.06247324680649,1.,1.71874858456908));
#22295=CARTESIAN_POINT('Ctrl Pts',(1.06738966975463,-1.,1.72238500928456));
#22296=CARTESIAN_POINT('Ctrl Pts',(1.06738966975463,1.,1.72238500928456));
#22297=CARTESIAN_POINT('Ctrl Pts',(1.07234866990252,-1.,1.72599406198489));
#22298=CARTESIAN_POINT('Ctrl Pts',(1.07234866990252,1.,1.72599406198489));
#22299=CARTESIAN_POINT('Ctrl Pts',(1.0773470373727,-1.,1.72957248977424));
#22300=CARTESIAN_POINT('Ctrl Pts',(1.0773470373727,1.,1.72957248977424));
#22301=CARTESIAN_POINT('Ctrl Pts',(1.08238162784749,-1.,1.73311705663407));
#22302=CARTESIAN_POINT('Ctrl Pts',(1.08238162784749,1.,1.73311705663407));
#22303=CARTESIAN_POINT('Ctrl Pts',(1.08745056285429,-1.,1.73662628326093));
#22304=CARTESIAN_POINT('Ctrl Pts',(1.08745056285429,1.,1.73662628326093));
#22305=CARTESIAN_POINT('Ctrl Pts',(1.09255329056496,-1.,1.74010053962252));
#22306=CARTESIAN_POINT('Ctrl Pts',(1.09255329056496,1.,1.74010053962252));
#22307=CARTESIAN_POINT('Ctrl Pts',(1.09768999241229,-1.,1.74354119236212));
#22308=CARTESIAN_POINT('Ctrl Pts',(1.09768999241229,1.,1.74354119236212));
#22309=CARTESIAN_POINT('Ctrl Pts',(1.10286118991144,-1.,1.74695004214924));
#22310=CARTESIAN_POINT('Ctrl Pts',(1.10286118991144,1.,1.74695004214924));
#22311=CARTESIAN_POINT('Ctrl Pts',(1.10806728183003,-1.,1.75032866075914));
#22312=CARTESIAN_POINT('Ctrl Pts',(1.10806728183003,1.,1.75032866075914));
#22313=CARTESIAN_POINT('Ctrl Pts',(1.11330807582542,-1.,1.75367772094617));
#22314=CARTESIAN_POINT('Ctrl Pts',(1.11330807582542,1.,1.75367772094617));
#22315=CARTESIAN_POINT('Ctrl Pts',(1.11858293216752,-1.,1.75699720772089));
#22316=CARTESIAN_POINT('Ctrl Pts',(1.11858293216752,1.,1.75699720772089));
#22317=CARTESIAN_POINT('Ctrl Pts',(1.12389096855078,-1.,1.76028671825084));
#22318=CARTESIAN_POINT('Ctrl Pts',(1.12389096855078,1.,1.76028671825084));
#22319=CARTESIAN_POINT('Ctrl Pts',(1.12923123555076,-1.,1.76354571966171));
#22320=CARTESIAN_POINT('Ctrl Pts',(1.12923123555076,1.,1.76354571966171));
#22321=CARTESIAN_POINT('Ctrl Pts',(1.13460291804634,-1.,1.76677384551883));
#22322=CARTESIAN_POINT('Ctrl Pts',(1.13460291804634,1.,1.76677384551883));
#22323=CARTESIAN_POINT('Ctrl Pts',(1.14000548337,-1.,1.76997111386806));
#22324=CARTESIAN_POINT('Ctrl Pts',(1.14000548337,1.,1.76997111386806));
#22325=CARTESIAN_POINT('Ctrl Pts',(1.14543858226948,-1.,1.77313777896234));
#22326=CARTESIAN_POINT('Ctrl Pts',(1.14543858226948,1.,1.77313777896234));
#22327=CARTESIAN_POINT('Ctrl Pts',(1.15090197841531,-1.,1.77627422557034));
#22328=CARTESIAN_POINT('Ctrl Pts',(1.15090197841531,1.,1.77627422557034));
#22329=CARTESIAN_POINT('Ctrl Pts',(1.15639547194689,-1.,1.77938085564261));
#22330=CARTESIAN_POINT('Ctrl Pts',(1.15639547194689,1.,1.77938085564261));
#22331=CARTESIAN_POINT('Ctrl Pts',(1.16191881298458,-1.,1.78245795880949));
#22332=CARTESIAN_POINT('Ctrl Pts',(1.16191881298458,1.,1.78245795880949));
#22333=CARTESIAN_POINT('Ctrl Pts',(1.16747166312239,-1.,1.78550566040349));
#22334=CARTESIAN_POINT('Ctrl Pts',(1.16747166312239,1.,1.78550566040349));
#22335=CARTESIAN_POINT('Ctrl Pts',(1.17305363177265,-1.,1.78852398877523));
#22336=CARTESIAN_POINT('Ctrl Pts',(1.17305363177265,1.,1.78852398877523));
#22337=CARTESIAN_POINT('Ctrl Pts',(1.17866429440781,-1.,1.79151291552646));
#22338=CARTESIAN_POINT('Ctrl Pts',(1.17866429440781,1.,1.79151291552646));
#22339=CARTESIAN_POINT('Ctrl Pts',(1.18430321697471,-1.,1.79447240321572));
#22340=CARTESIAN_POINT('Ctrl Pts',(1.18430321697471,1.,1.79447240321572));
#22341=CARTESIAN_POINT('Ctrl Pts',(1.1899699793456,-1.,1.79740245923649));
#22342=CARTESIAN_POINT('Ctrl Pts',(1.1899699793456,1.,1.79740245923649));
#22343=CARTESIAN_POINT('Ctrl Pts',(1.19566418930405,-1.,1.80030314370121));
#22344=CARTESIAN_POINT('Ctrl Pts',(1.19566418930405,1.,1.80030314370121));
#22345=CARTESIAN_POINT('Ctrl Pts',(1.2013854893912,-1.,1.8031745483882));
#22346=CARTESIAN_POINT('Ctrl Pts',(1.2013854893912,1.,1.8031745483882));
#22347=CARTESIAN_POINT('Ctrl Pts',(1.20713356605519,-1.,1.80601678480772));
#22348=CARTESIAN_POINT('Ctrl Pts',(1.20713356605519,1.,1.80601678480772));
#22349=CARTESIAN_POINT('Ctrl Pts',(1.2129081570818,-1.,1.80882996916931));
#22350=CARTESIAN_POINT('Ctrl Pts',(1.2129081570818,1.,1.80882996916931));
#22351=CARTESIAN_POINT('Ctrl Pts',(1.2187090610323,-1.,1.81161420806172));
#22352=CARTESIAN_POINT('Ctrl Pts',(1.2187090610323,1.,1.81161420806172));
#22353=CARTESIAN_POINT('Ctrl Pts',(1.22453613304507,-1.,1.81436959209778));
#22354=CARTESIAN_POINT('Ctrl Pts',(1.22453613304507,1.,1.81436959209778));
#22355=CARTESIAN_POINT('Ctrl Pts',(1.22921864890975,-1.,1.81655087183054));
#22356=CARTESIAN_POINT('Ctrl Pts',(1.22921864890975,1.,1.81655087183054));
#22357=CARTESIAN_POINT('Ctrl Pts',(1.23274224526804,-1.,1.81817389920914));
#22358=CARTESIAN_POINT('Ctrl Pts',(1.23274224526804,1.,1.81817389920914));
#22359=CARTESIAN_POINT('Ctrl Pts',(1.23509651170384,-1.,1.81925017193531));
#22360=CARTESIAN_POINT('Ctrl Pts',(1.23509651170384,1.,1.81925017193531));
#22361=CARTESIAN_POINT('Ctrl Pts',(1.23627494547115,-1.,1.81978687191668));
#22362=CARTESIAN_POINT('Ctrl Pts',(1.23627494547115,1.,1.81978687191668));
#22363=CARTESIAN_POINT('',(0.892032620296855,1.,1.5055822144029));
#22364=CARTESIAN_POINT('Ctrl Pts',(0.892032620296855,1.,1.5055822144029));
#22365=CARTESIAN_POINT('Ctrl Pts',(0.894452006967538,1.,1.50980486807181));
#22366=CARTESIAN_POINT('Ctrl Pts',(0.89918504749193,1.,1.51805569591479));
#22367=CARTESIAN_POINT('Ctrl Pts',(0.905967409640498,1.,1.52984849890434));
#22368=CARTESIAN_POINT('Ctrl Pts',(0.914375919046579,1.,1.54440491152808));
#22369=CARTESIAN_POINT('Ctrl Pts',(0.923832188966322,1.,1.56065988582509));
#22370=CARTESIAN_POINT('Ctrl Pts',(0.932246680128848,1.,1.57499388385561));
#22371=CARTESIAN_POINT('Ctrl Pts',(0.939646377909319,1.,1.58744937489796));
#22372=CARTESIAN_POINT('Ctrl Pts',(0.946078063325795,1.,1.59810042045408));
#22373=CARTESIAN_POINT('Ctrl Pts',(0.951613284361247,1.,1.60706069897794));
#22374=CARTESIAN_POINT('Ctrl Pts',(0.956354422921572,1.,1.61449324337233));
#22375=CARTESIAN_POINT('Ctrl Pts',(0.960438326099958,1.,1.62061638139929));
#22376=CARTESIAN_POINT('Ctrl Pts',(0.964046107037821,1.,1.6257193066974));
#22377=CARTESIAN_POINT('Ctrl Pts',(0.967387853228041,1.,1.63013849959083));
#22378=CARTESIAN_POINT('Ctrl Pts',(0.970669715996356,1.,1.63420665729609));
#22379=CARTESIAN_POINT('Ctrl Pts',(0.974066058287501,1.,1.63820952658157));
#22380=CARTESIAN_POINT('Ctrl Pts',(0.977689794120296,1.,1.64233990826831));
#22381=CARTESIAN_POINT('Ctrl Pts',(0.981562530940574,1.,1.64665139190834));
#22382=CARTESIAN_POINT('Ctrl Pts',(0.985642622921626,1.,1.6511001661277));
#22383=CARTESIAN_POINT('Ctrl Pts',(0.98985562785445,1.,1.65559044289746));
#22384=CARTESIAN_POINT('Ctrl Pts',(0.994121836661115,1.,1.66001553809916));
#22385=CARTESIAN_POINT('Ctrl Pts',(0.998389654952317,1.,1.66430758030304));
#22386=CARTESIAN_POINT('Ctrl Pts',(1.00265091003682,1.,1.66846059277231));
#22387=CARTESIAN_POINT('Ctrl Pts',(1.00692206696387,1.,1.67250335383248));
#22388=CARTESIAN_POINT('Ctrl Pts',(1.01123236493507,1.,1.67648246776457));
#22389=CARTESIAN_POINT('Ctrl Pts',(1.01561026162786,1.,1.6804428989482));
#22390=CARTESIAN_POINT('Ctrl Pts',(1.02006795074222,1.,1.68440578021739));
#22391=CARTESIAN_POINT('Ctrl Pts',(1.02460180535272,1.,1.68836910178475));
#22392=CARTESIAN_POINT('Ctrl Pts',(1.02919977579155,1.,1.69231840863471));
#22393=CARTESIAN_POINT('Ctrl Pts',(1.03384646003587,1.,1.69623414782769));
#22394=CARTESIAN_POINT('Ctrl Pts',(1.03852922490782,1.,1.70010052930951));
#22395=CARTESIAN_POINT('Ctrl Pts',(1.04324363334546,1.,1.70391338707969));
#22396=CARTESIAN_POINT('Ctrl Pts',(1.0479908540499,1.,1.70767646263641));
#22397=CARTESIAN_POINT('Ctrl Pts',(1.05277517202853,1.,1.71139783543986));
#22398=CARTESIAN_POINT('Ctrl Pts',(1.05760163192481,1.,1.71508654427022));
#22399=CARTESIAN_POINT('Ctrl Pts',(1.06247324680649,1.,1.71874858456908));
#22400=CARTESIAN_POINT('Ctrl Pts',(1.06738966975463,1.,1.72238500928456));
#22401=CARTESIAN_POINT('Ctrl Pts',(1.07234866990252,1.,1.72599406198489));
#22402=CARTESIAN_POINT('Ctrl Pts',(1.0773470373727,1.,1.72957248977424));
#22403=CARTESIAN_POINT('Ctrl Pts',(1.08238162784749,1.,1.73311705663407));
#22404=CARTESIAN_POINT('Ctrl Pts',(1.08745056285429,1.,1.73662628326093));
#22405=CARTESIAN_POINT('Ctrl Pts',(1.09255329056496,1.,1.74010053962252));
#22406=CARTESIAN_POINT('Ctrl Pts',(1.09768999241229,1.,1.74354119236212));
#22407=CARTESIAN_POINT('Ctrl Pts',(1.10286118991144,1.,1.74695004214924));
#22408=CARTESIAN_POINT('Ctrl Pts',(1.10806728183003,1.,1.75032866075914));
#22409=CARTESIAN_POINT('Ctrl Pts',(1.11330807582542,1.,1.75367772094617));
#22410=CARTESIAN_POINT('Ctrl Pts',(1.11858293216752,1.,1.75699720772089));
#22411=CARTESIAN_POINT('Ctrl Pts',(1.12389096855078,1.,1.76028671825084));
#22412=CARTESIAN_POINT('Ctrl Pts',(1.12923123555076,1.,1.76354571966171));
#22413=CARTESIAN_POINT('Ctrl Pts',(1.13460291804634,1.,1.76677384551883));
#22414=CARTESIAN_POINT('Ctrl Pts',(1.14000548337,1.,1.76997111386806));
#22415=CARTESIAN_POINT('Ctrl Pts',(1.14543858226948,1.,1.77313777896234));
#22416=CARTESIAN_POINT('Ctrl Pts',(1.15090197841531,1.,1.77627422557034));
#22417=CARTESIAN_POINT('Ctrl Pts',(1.15639547194689,1.,1.77938085564261));
#22418=CARTESIAN_POINT('Ctrl Pts',(1.16191881298458,1.,1.78245795880949));
#22419=CARTESIAN_POINT('Ctrl Pts',(1.16747166312239,1.,1.78550566040349));
#22420=CARTESIAN_POINT('Ctrl Pts',(1.17305363177265,1.,1.78852398877523));
#22421=CARTESIAN_POINT('Ctrl Pts',(1.17866429440781,1.,1.79151291552646));
#22422=CARTESIAN_POINT('Ctrl Pts',(1.18430321697471,1.,1.79447240321572));
#22423=CARTESIAN_POINT('Ctrl Pts',(1.1899699793456,1.,1.79740245923649));
#22424=CARTESIAN_POINT('Ctrl Pts',(1.19566418930405,1.,1.80030314370121));
#22425=CARTESIAN_POINT('Ctrl Pts',(1.2013854893912,1.,1.8031745483882));
#22426=CARTESIAN_POINT('Ctrl Pts',(1.20713356605519,1.,1.80601678480772));
#22427=CARTESIAN_POINT('Ctrl Pts',(1.2129081570818,1.,1.80882996916931));
#22428=CARTESIAN_POINT('Ctrl Pts',(1.2187090610323,1.,1.81161420806172));
#22429=CARTESIAN_POINT('Ctrl Pts',(1.22453613304507,1.,1.81436959209778));
#22430=CARTESIAN_POINT('Ctrl Pts',(1.22921864890975,1.,1.81655087183054));
#22431=CARTESIAN_POINT('Ctrl Pts',(1.23274224526804,1.,1.81817389920914));
#22432=CARTESIAN_POINT('Ctrl Pts',(1.23509651170384,1.,1.81925017193531));
#22433=CARTESIAN_POINT('Ctrl Pts',(1.23627494547115,1.,1.81978687191668));
#22434=CARTESIAN_POINT('',(0.892032620296854,0.,1.5055822144029));
#22435=CARTESIAN_POINT('Origin',(0.,0.,0.));
#22436=CARTESIAN_POINT('',(0.693717979106305,1.,1.60662857109684));
#22437=CARTESIAN_POINT('Origin',(0.,1.,0.));
#22438=CARTESIAN_POINT('',(0.693717979106305,0.,1.60662857109684));
#22439=CARTESIAN_POINT('Ctrl Pts',(0.7455743247944,-1.,2.0698113262342));
#22440=CARTESIAN_POINT('Ctrl Pts',(0.7455743247944,1.,2.0698113262342));
#22441=CARTESIAN_POINT('Ctrl Pts',(0.745832791378367,-1.,2.06854248895728));
#22442=CARTESIAN_POINT('Ctrl Pts',(0.745832791378367,1.,2.06854248895728));
#22443=CARTESIAN_POINT('Ctrl Pts',(0.7463458715442,-1.,2.06600523016815));
#22444=CARTESIAN_POINT('Ctrl Pts',(0.7463458715442,1.,2.06600523016815));
#22445=CARTESIAN_POINT('Ctrl Pts',(0.747103932787919,-1.,2.06220058927826));
#22446=CARTESIAN_POINT('Ctrl Pts',(0.747103932787919,1.,2.06220058927826));
#22447=CARTESIAN_POINT('Ctrl Pts',(0.748091554183802,-1.,2.05713023031007));
#22448=CARTESIAN_POINT('Ctrl Pts',(0.748091554183802,1.,2.05713023031007));
#22449=CARTESIAN_POINT('Ctrl Pts',(0.749287468665046,-1.,2.05079645592154));
#22450=CARTESIAN_POINT('Ctrl Pts',(0.749287468665046,1.,2.05079645592154));
#22451=CARTESIAN_POINT('Ctrl Pts',(0.750444657875575,-1.,2.04446689147979));
#22452=CARTESIAN_POINT('Ctrl Pts',(0.750444657875575,1.,2.04446689147979));
#22453=CARTESIAN_POINT('Ctrl Pts',(0.751562963361115,-1.,2.03814160092099));
#22454=CARTESIAN_POINT('Ctrl Pts',(0.751562963361115,1.,2.03814160092099));
#22455=CARTESIAN_POINT('Ctrl Pts',(0.75264218048721,-1.,2.03182068456221));
#22456=CARTESIAN_POINT('Ctrl Pts',(0.75264218048721,1.,2.03182068456221));
#22457=CARTESIAN_POINT('Ctrl Pts',(0.753682061112768,-1.,2.02550428623313));
#22458=CARTESIAN_POINT('Ctrl Pts',(0.753682061112768,1.,2.02550428623313));
#22459=CARTESIAN_POINT('Ctrl Pts',(0.754682330722816,-1.,2.01919259405809));
#22460=CARTESIAN_POINT('Ctrl Pts',(0.754682330722816,1.,2.01919259405809));
#22461=CARTESIAN_POINT('Ctrl Pts',(0.755642704957865,-1.,2.01288584328084));
#22462=CARTESIAN_POINT('Ctrl Pts',(0.755642704957865,1.,2.01288584328084));
#22463=CARTESIAN_POINT('Ctrl Pts',(0.75656290464667,-1.,2.0065843158773));
#22464=CARTESIAN_POINT('Ctrl Pts',(0.75656290464667,1.,2.0065843158773));
#22465=CARTESIAN_POINT('Ctrl Pts',(0.757442676862724,-1.,2.00028834739178));
#22466=CARTESIAN_POINT('Ctrl Pts',(0.757442676862724,1.,2.00028834739178));
#22467=CARTESIAN_POINT('Ctrl Pts',(0.758281796766761,-1.,1.99399831098817));
#22468=CARTESIAN_POINT('Ctrl Pts',(0.758281796766761,1.,1.99399831098817));
#22469=CARTESIAN_POINT('Ctrl Pts',(0.759080037802488,-1.,1.98771456680874));
#22470=CARTESIAN_POINT('Ctrl Pts',(0.759080037802488,1.,1.98771456680874));
#22471=CARTESIAN_POINT('Ctrl Pts',(0.75983714745219,-1.,1.98143741418172));
#22472=CARTESIAN_POINT('Ctrl Pts',(0.75983714745219,1.,1.98143741418172));
#22473=CARTESIAN_POINT('Ctrl Pts',(0.760552825409757,-1.,1.97516705321494));
#22474=CARTESIAN_POINT('Ctrl Pts',(0.760552825409757,1.,1.97516705321494));
#22475=CARTESIAN_POINT('Ctrl Pts',(0.76122669048382,-1.,1.96890351582499));
#22476=CARTESIAN_POINT('Ctrl Pts',(0.76122669048382,1.,1.96890351582499));
#22477=CARTESIAN_POINT('Ctrl Pts',(0.761858300014423,-1.,1.96264672744186));
#22478=CARTESIAN_POINT('Ctrl Pts',(0.761858300014423,1.,1.96264672744186));
#22479=CARTESIAN_POINT('Ctrl Pts',(0.762447203806178,-1.,1.95639665309869));
#22480=CARTESIAN_POINT('Ctrl Pts',(0.762447203806178,1.,1.95639665309869));
#22481=CARTESIAN_POINT('Ctrl Pts',(0.762992990878769,-1.,1.95015342590024));
#22482=CARTESIAN_POINT('Ctrl Pts',(0.762992990878769,1.,1.95015342590024));
#22483=CARTESIAN_POINT('Ctrl Pts',(0.763495333538629,-1.,1.9439174661764));
#22484=CARTESIAN_POINT('Ctrl Pts',(0.763495333538629,1.,1.9439174661764));
#22485=CARTESIAN_POINT('Ctrl Pts',(0.763954049121458,-1.,1.93768964875886));
#22486=CARTESIAN_POINT('Ctrl Pts',(0.763954049121458,1.,1.93768964875886));
#22487=CARTESIAN_POINT('Ctrl Pts',(0.76436901067394,-1.,1.93147105496382));
#22488=CARTESIAN_POINT('Ctrl Pts',(0.76436901067394,1.,1.93147105496382));
#22489=CARTESIAN_POINT('Ctrl Pts',(0.764740025488211,-1.,1.92526263537048));
#22490=CARTESIAN_POINT('Ctrl Pts',(0.764740025488211,1.,1.92526263537048));
#22491=CARTESIAN_POINT('Ctrl Pts',(0.765066729667088,-1.,1.91906491634196));
#22492=CARTESIAN_POINT('Ctrl Pts',(0.765066729667088,1.,1.91906491634196));
#22493=CARTESIAN_POINT('Ctrl Pts',(0.765348465884722,-1.,1.91287765805169));
#22494=CARTESIAN_POINT('Ctrl Pts',(0.765348465884722,1.,1.91287765805169));
#22495=CARTESIAN_POINT('Ctrl Pts',(0.765584196937919,-1.,1.90669961402356));
#22496=CARTESIAN_POINT('Ctrl Pts',(0.765584196937919,1.,1.90669961402356));
#22497=CARTESIAN_POINT('Ctrl Pts',(0.765772772593386,-1.,1.90052930393596));
#22498=CARTESIAN_POINT('Ctrl Pts',(0.765772772593386,1.,1.90052930393596));
#22499=CARTESIAN_POINT('Ctrl Pts',(0.765913193856978,-1.,1.89436577771388));
#22500=CARTESIAN_POINT('Ctrl Pts',(0.765913193856978,1.,1.89436577771388));
#22501=CARTESIAN_POINT('Ctrl Pts',(0.766004837062091,-1.,1.88820926433409));
#22502=CARTESIAN_POINT('Ctrl Pts',(0.766004837062091,1.,1.88820926433409));
#22503=CARTESIAN_POINT('Ctrl Pts',(0.766047794851864,-1.,1.88206215302561));
#22504=CARTESIAN_POINT('Ctrl Pts',(0.766047794851864,1.,1.88206215302561));
#22505=CARTESIAN_POINT('Ctrl Pts',(0.766042837036744,-1.,1.87592888967883));
#22506=CARTESIAN_POINT('Ctrl Pts',(0.766042837036744,1.,1.87592888967883));
#22507=CARTESIAN_POINT('Ctrl Pts',(0.765990708546091,-1.,1.86981398314341));
#22508=CARTESIAN_POINT('Ctrl Pts',(0.765990708546091,1.,1.86981398314341));
#22509=CARTESIAN_POINT('Ctrl Pts',(0.765891519092547,-1.,1.86372027063312));
#22510=CARTESIAN_POINT('Ctrl Pts',(0.765891519092547,1.,1.86372027063312));
#22511=CARTESIAN_POINT('Ctrl Pts',(0.765744212909318,-1.,1.85764741390394));
#22512=CARTESIAN_POINT('Ctrl Pts',(0.765744212909318,1.,1.85764741390394));
#22513=CARTESIAN_POINT('Ctrl Pts',(0.765545710619062,-1.,1.85158945130063));
#22514=CARTESIAN_POINT('Ctrl Pts',(0.765545710619062,1.,1.85158945130063));
#22515=CARTESIAN_POINT('Ctrl Pts',(0.765291664862029,-1.,1.84553698875924));
#22516=CARTESIAN_POINT('Ctrl Pts',(0.765291664862029,1.,1.84553698875924));
#22517=CARTESIAN_POINT('Ctrl Pts',(0.764978057881737,-1.,1.83948181064835));
#22518=CARTESIAN_POINT('Ctrl Pts',(0.764978057881737,1.,1.83948181064835));
#22519=CARTESIAN_POINT('Ctrl Pts',(0.764602549687853,-1.,1.83342077227142));
#22520=CARTESIAN_POINT('Ctrl Pts',(0.764602549687853,1.,1.83342077227142));
#22521=CARTESIAN_POINT('Ctrl Pts',(0.764165902605995,-1.,1.82735991200065));
#22522=CARTESIAN_POINT('Ctrl Pts',(0.764165902605995,1.,1.82735991200065));
#22523=CARTESIAN_POINT('Ctrl Pts',(0.763673465462726,-1.,1.82131873145266));
#22524=CARTESIAN_POINT('Ctrl Pts',(0.763673465462726,1.,1.82131873145266));
#22525=CARTESIAN_POINT('Ctrl Pts',(0.763132003836634,-1.,1.8153211840553));
#22526=CARTESIAN_POINT('Ctrl Pts',(0.763132003836634,1.,1.8153211840553));
#22527=CARTESIAN_POINT('Ctrl Pts',(0.762546129463938,-1.,1.80938551463965));
#22528=CARTESIAN_POINT('Ctrl Pts',(0.762546129463938,1.,1.80938551463965));
#22529=CARTESIAN_POINT('Ctrl Pts',(0.761915336443547,-1.,1.80351583877342));
#22530=CARTESIAN_POINT('Ctrl Pts',(0.761915336443547,1.,1.80351583877342));
#22531=CARTESIAN_POINT('Ctrl Pts',(0.761229695230558,-1.,1.79768986997783));
#22532=CARTESIAN_POINT('Ctrl Pts',(0.761229695230558,1.,1.79768986997783));
#22533=CARTESIAN_POINT('Ctrl Pts',(0.760469555880749,-1.,1.7918581561088));
#22534=CARTESIAN_POINT('Ctrl Pts',(0.760469555880749,1.,1.7918581561088));
#22535=CARTESIAN_POINT('Ctrl Pts',(0.759614401110189,-1.,1.78596964884604));
#22536=CARTESIAN_POINT('Ctrl Pts',(0.759614401110189,1.,1.78596964884604));
#22537=CARTESIAN_POINT('Ctrl Pts',(0.758650626677518,-1.,1.77999411220945));
#22538=CARTESIAN_POINT('Ctrl Pts',(0.758650626677518,1.,1.77999411220945));
#22539=CARTESIAN_POINT('Ctrl Pts',(0.757578264077028,-1.,1.77394167108292));
#22540=CARTESIAN_POINT('Ctrl Pts',(0.757578264077028,1.,1.77394167108292));
#22541=CARTESIAN_POINT('Ctrl Pts',(0.75642189602781,-1.,1.76789396002998));
#22542=CARTESIAN_POINT('Ctrl Pts',(0.75642189602781,1.,1.76789396002998));
#22543=CARTESIAN_POINT('Ctrl Pts',(0.755220979974461,-1.,1.76197817240128));
#22544=CARTESIAN_POINT('Ctrl Pts',(0.755220979974461,1.,1.76197817240128));
#22545=CARTESIAN_POINT('Ctrl Pts',(0.754009254027828,-1.,1.75631083600019));
#22546=CARTESIAN_POINT('Ctrl Pts',(0.754009254027828,1.,1.75631083600019));
#22547=CARTESIAN_POINT('Ctrl Pts',(0.752797683531314,-1.,1.75095139468794));
#22548=CARTESIAN_POINT('Ctrl Pts',(0.752797683531314,1.,1.75095139468794));
#22549=CARTESIAN_POINT('Ctrl Pts',(0.751555614164482,-1.,1.74585086852502));
#22550=CARTESIAN_POINT('Ctrl Pts',(0.751555614164482,1.,1.74585086852502));
#22551=CARTESIAN_POINT('Ctrl Pts',(0.750193435981249,-1.,1.74080458267114));
#22552=CARTESIAN_POINT('Ctrl Pts',(0.750193435981249,1.,1.74080458267114));
#22553=CARTESIAN_POINT('Ctrl Pts',(0.74858246295687,-1.,1.7355035168033));
#22554=CARTESIAN_POINT('Ctrl Pts',(0.74858246295687,1.,1.7355035168033));
#22555=CARTESIAN_POINT('Ctrl Pts',(0.746574710097752,-1.,1.72958533647714));
#22556=CARTESIAN_POINT('Ctrl Pts',(0.746574710097752,1.,1.72958533647714));
#22557=CARTESIAN_POINT('Ctrl Pts',(0.744021445433093,-1.,1.72268229916769));
#22558=CARTESIAN_POINT('Ctrl Pts',(0.744021445433093,1.,1.72268229916769));
#22559=CARTESIAN_POINT('Ctrl Pts',(0.74079516202821,-1.,1.71447789751001));
#22560=CARTESIAN_POINT('Ctrl Pts',(0.74079516202821,1.,1.71447789751001));
#22561=CARTESIAN_POINT('Ctrl Pts',(0.736799665716932,-1.,1.70473309004249));
#22562=CARTESIAN_POINT('Ctrl Pts',(0.736799665716932,1.,1.70473309004249));
#22563=CARTESIAN_POINT('Ctrl Pts',(0.731963238685357,-1.,1.69326921972915));
#22564=CARTESIAN_POINT('Ctrl Pts',(0.731963238685357,1.,1.69326921972915));
#22565=CARTESIAN_POINT('Ctrl Pts',(0.726235967982445,-1.,1.67996158451922));
#22566=CARTESIAN_POINT('Ctrl Pts',(0.726235967982445,1.,1.67996158451922));
#22567=CARTESIAN_POINT('Ctrl Pts',(0.719585433787949,-1.,1.66472880551777));
#22568=CARTESIAN_POINT('Ctrl Pts',(0.719585433787949,1.,1.66472880551777));
#22569=CARTESIAN_POINT('Ctrl Pts',(0.711993139340447,-1.,1.64752408828442));
#22570=CARTESIAN_POINT('Ctrl Pts',(0.711993139340447,1.,1.64752408828442));
#22571=CARTESIAN_POINT('Ctrl Pts',(0.705159151977294,-1.,1.6321654166204));
#22572=CARTESIAN_POINT('Ctrl Pts',(0.705159151977294,1.,1.6321654166204));
#22573=CARTESIAN_POINT('Ctrl Pts',(0.699605146398836,-1.,1.61974673471117));
#22574=CARTESIAN_POINT('Ctrl Pts',(0.699605146398836,1.,1.61974673471117));
#22575=CARTESIAN_POINT('Ctrl Pts',(0.69571209787897,-1.,1.61106790957619));
#22576=CARTESIAN_POINT('Ctrl Pts',(0.69571209787897,1.,1.61106790957619));
#22577=CARTESIAN_POINT('Ctrl Pts',(0.693717979106305,-1.,1.60662857109684));
#22578=CARTESIAN_POINT('Ctrl Pts',(0.693717979106305,1.,1.60662857109684));
#22579=CARTESIAN_POINT('',(0.7455743247944,1.,2.0698113262342));
#22580=CARTESIAN_POINT('Ctrl Pts',(0.7455743247944,1.,2.0698113262342));
#22581=CARTESIAN_POINT('Ctrl Pts',(0.745832791378367,1.,2.06854248895728));
#22582=CARTESIAN_POINT('Ctrl Pts',(0.7463458715442,1.,2.06600523016815));
#22583=CARTESIAN_POINT('Ctrl Pts',(0.747103932787919,1.,2.06220058927826));
#22584=CARTESIAN_POINT('Ctrl Pts',(0.748091554183802,1.,2.05713023031007));
#22585=CARTESIAN_POINT('Ctrl Pts',(0.749287468665046,1.,2.05079645592154));
#22586=CARTESIAN_POINT('Ctrl Pts',(0.750444657875575,1.,2.04446689147979));
#22587=CARTESIAN_POINT('Ctrl Pts',(0.751562963361115,1.,2.03814160092099));
#22588=CARTESIAN_POINT('Ctrl Pts',(0.75264218048721,1.,2.03182068456221));
#22589=CARTESIAN_POINT('Ctrl Pts',(0.753682061112768,1.,2.02550428623313));
#22590=CARTESIAN_POINT('Ctrl Pts',(0.754682330722816,1.,2.01919259405809));
#22591=CARTESIAN_POINT('Ctrl Pts',(0.755642704957865,1.,2.01288584328084));
#22592=CARTESIAN_POINT('Ctrl Pts',(0.75656290464667,1.,2.0065843158773));
#22593=CARTESIAN_POINT('Ctrl Pts',(0.757442676862724,1.,2.00028834739178));
#22594=CARTESIAN_POINT('Ctrl Pts',(0.758281796766761,1.,1.99399831098817));
#22595=CARTESIAN_POINT('Ctrl Pts',(0.759080037802488,1.,1.98771456680874));
#22596=CARTESIAN_POINT('Ctrl Pts',(0.75983714745219,1.,1.98143741418172));
#22597=CARTESIAN_POINT('Ctrl Pts',(0.760552825409757,1.,1.97516705321494));
#22598=CARTESIAN_POINT('Ctrl Pts',(0.76122669048382,1.,1.96890351582499));
#22599=CARTESIAN_POINT('Ctrl Pts',(0.761858300014423,1.,1.96264672744186));
#22600=CARTESIAN_POINT('Ctrl Pts',(0.762447203806178,1.,1.95639665309869));
#22601=CARTESIAN_POINT('Ctrl Pts',(0.762992990878769,1.,1.95015342590024));
#22602=CARTESIAN_POINT('Ctrl Pts',(0.763495333538629,1.,1.9439174661764));
#22603=CARTESIAN_POINT('Ctrl Pts',(0.763954049121458,1.,1.93768964875886));
#22604=CARTESIAN_POINT('Ctrl Pts',(0.76436901067394,1.,1.93147105496382));
#22605=CARTESIAN_POINT('Ctrl Pts',(0.764740025488211,1.,1.92526263537048));
#22606=CARTESIAN_POINT('Ctrl Pts',(0.765066729667088,1.,1.91906491634196));
#22607=CARTESIAN_POINT('Ctrl Pts',(0.765348465884722,1.,1.91287765805169));
#22608=CARTESIAN_POINT('Ctrl Pts',(0.765584196937919,1.,1.90669961402356));
#22609=CARTESIAN_POINT('Ctrl Pts',(0.765772772593386,1.,1.90052930393596));
#22610=CARTESIAN_POINT('Ctrl Pts',(0.765913193856978,1.,1.89436577771388));
#22611=CARTESIAN_POINT('Ctrl Pts',(0.766004837062091,1.,1.88820926433409));
#22612=CARTESIAN_POINT('Ctrl Pts',(0.766047794851864,1.,1.88206215302561));
#22613=CARTESIAN_POINT('Ctrl Pts',(0.766042837036744,1.,1.87592888967883));
#22614=CARTESIAN_POINT('Ctrl Pts',(0.765990708546091,1.,1.86981398314341));
#22615=CARTESIAN_POINT('Ctrl Pts',(0.765891519092547,1.,1.86372027063312));
#22616=CARTESIAN_POINT('Ctrl Pts',(0.765744212909318,1.,1.85764741390394));
#22617=CARTESIAN_POINT('Ctrl Pts',(0.765545710619062,1.,1.85158945130063));
#22618=CARTESIAN_POINT('Ctrl Pts',(0.765291664862029,1.,1.84553698875924));
#22619=CARTESIAN_POINT('Ctrl Pts',(0.764978057881737,1.,1.83948181064835));
#22620=CARTESIAN_POINT('Ctrl Pts',(0.764602549687853,1.,1.83342077227142));
#22621=CARTESIAN_POINT('Ctrl Pts',(0.764165902605995,1.,1.82735991200065));
#22622=CARTESIAN_POINT('Ctrl Pts',(0.763673465462726,1.,1.82131873145266));
#22623=CARTESIAN_POINT('Ctrl Pts',(0.763132003836634,1.,1.8153211840553));
#22624=CARTESIAN_POINT('Ctrl Pts',(0.762546129463938,1.,1.80938551463965));
#22625=CARTESIAN_POINT('Ctrl Pts',(0.761915336443547,1.,1.80351583877342));
#22626=CARTESIAN_POINT('Ctrl Pts',(0.761229695230558,1.,1.79768986997783));
#22627=CARTESIAN_POINT('Ctrl Pts',(0.760469555880749,1.,1.7918581561088));
#22628=CARTESIAN_POINT('Ctrl Pts',(0.759614401110189,1.,1.78596964884604));
#22629=CARTESIAN_POINT('Ctrl Pts',(0.758650626677518,1.,1.77999411220945));
#22630=CARTESIAN_POINT('Ctrl Pts',(0.757578264077028,1.,1.77394167108292));
#22631=CARTESIAN_POINT('Ctrl Pts',(0.75642189602781,1.,1.76789396002998));
#22632=CARTESIAN_POINT('Ctrl Pts',(0.755220979974461,1.,1.76197817240128));
#22633=CARTESIAN_POINT('Ctrl Pts',(0.754009254027828,1.,1.75631083600019));
#22634=CARTESIAN_POINT('Ctrl Pts',(0.752797683531314,1.,1.75095139468794));
#22635=CARTESIAN_POINT('Ctrl Pts',(0.751555614164482,1.,1.74585086852502));
#22636=CARTESIAN_POINT('Ctrl Pts',(0.750193435981249,1.,1.74080458267114));
#22637=CARTESIAN_POINT('Ctrl Pts',(0.74858246295687,1.,1.7355035168033));
#22638=CARTESIAN_POINT('Ctrl Pts',(0.746574710097752,1.,1.72958533647714));
#22639=CARTESIAN_POINT('Ctrl Pts',(0.744021445433093,1.,1.72268229916769));
#22640=CARTESIAN_POINT('Ctrl Pts',(0.74079516202821,1.,1.71447789751001));
#22641=CARTESIAN_POINT('Ctrl Pts',(0.736799665716932,1.,1.70473309004249));
#22642=CARTESIAN_POINT('Ctrl Pts',(0.731963238685357,1.,1.69326921972915));
#22643=CARTESIAN_POINT('Ctrl Pts',(0.726235967982445,1.,1.67996158451922));
#22644=CARTESIAN_POINT('Ctrl Pts',(0.719585433787949,1.,1.66472880551777));
#22645=CARTESIAN_POINT('Ctrl Pts',(0.711993139340447,1.,1.64752408828442));
#22646=CARTESIAN_POINT('Ctrl Pts',(0.705159151977294,1.,1.6321654166204));
#22647=CARTESIAN_POINT('Ctrl Pts',(0.699605146398836,1.,1.61974673471117));
#22648=CARTESIAN_POINT('Ctrl Pts',(0.69571209787897,1.,1.61106790957619));
#22649=CARTESIAN_POINT('Ctrl Pts',(0.693717979106305,1.,1.60662857109684));
#22650=CARTESIAN_POINT('',(0.7455743247944,0.,2.0698113262342));
#22651=CARTESIAN_POINT('Origin',(0.61342227326009,0.,2.11275013067528));
#22652=CARTESIAN_POINT('',(0.61342227326009,1.,2.11275013067528));
#22653=CARTESIAN_POINT('',(0.7455743247944,1.,2.0698113262342));
#22654=CARTESIAN_POINT('',(0.61342227326009,0.,2.11275013067528));
#22655=CARTESIAN_POINT('Ctrl Pts',(0.383122945602004,-1.,1.7075470150345));
#22656=CARTESIAN_POINT('Ctrl Pts',(0.383122945602004,1.,1.7075470150345));
#22657=CARTESIAN_POINT('Ctrl Pts',(0.384119047315541,-1.,1.71231062891958));
#22658=CARTESIAN_POINT('Ctrl Pts',(0.384119047315541,1.,1.71231062891958));
#22659=CARTESIAN_POINT('Ctrl Pts',(0.38607079032701,-1.,1.72162022246158));
#22660=CARTESIAN_POINT('Ctrl Pts',(0.38607079032701,1.,1.72162022246158));
#22661=CARTESIAN_POINT('Ctrl Pts',(0.388877023509191,-1.,1.7349317097561));
#22662=CARTESIAN_POINT('Ctrl Pts',(0.388877023509191,1.,1.7349317097561));
#22663=CARTESIAN_POINT('Ctrl Pts',(0.392375812294307,-1.,1.75137405313962));
#22664=CARTESIAN_POINT('Ctrl Pts',(0.392375812294307,1.,1.75137405313962));
#22665=CARTESIAN_POINT('Ctrl Pts',(0.39634619612042,-1.,1.7697556004756));
#22666=CARTESIAN_POINT('Ctrl Pts',(0.39634619612042,1.,1.7697556004756));
#22667=CARTESIAN_POINT('Ctrl Pts',(0.39991940378308,-1.,1.78598826347533));
#22668=CARTESIAN_POINT('Ctrl Pts',(0.39991940378308,1.,1.78598826347533));
#22669=CARTESIAN_POINT('Ctrl Pts',(0.403107976170441,-1.,1.80012077176221));
#22670=CARTESIAN_POINT('Ctrl Pts',(0.403107976170441,1.,1.80012077176221));
#22671=CARTESIAN_POINT('Ctrl Pts',(0.405933518411838,-1.,1.81223801813988));
#22672=CARTESIAN_POINT('Ctrl Pts',(0.405933518411838,1.,1.81223801813988));
#22673=CARTESIAN_POINT('Ctrl Pts',(0.408428948108533,-1.,1.8224702267854));
#22674=CARTESIAN_POINT('Ctrl Pts',(0.408428948108533,1.,1.8224702267854));
#22675=CARTESIAN_POINT('Ctrl Pts',(0.410641256301674,-1.,1.83100408895216));
#22676=CARTESIAN_POINT('Ctrl Pts',(0.410641256301674,1.,1.83100408895216));
#22677=CARTESIAN_POINT('Ctrl Pts',(0.412633125322161,-1.,1.83808953475839));
#22678=CARTESIAN_POINT('Ctrl Pts',(0.412633125322161,1.,1.83808953475839));
#22679=CARTESIAN_POINT('Ctrl Pts',(0.41448743825434,-1.,1.8440575707371));
#22680=CARTESIAN_POINT('Ctrl Pts',(0.41448743825434,1.,1.8440575707371));
#22681=CARTESIAN_POINT('Ctrl Pts',(0.416300022038864,-1.,1.84929312929882));
#22682=CARTESIAN_POINT('Ctrl Pts',(0.416300022038864,1.,1.84929312929882));
#22683=CARTESIAN_POINT('Ctrl Pts',(0.418164129143534,-1.,1.85417632856234));
#22684=CARTESIAN_POINT('Ctrl Pts',(0.418164129143534,1.,1.85417632856234));
#22685=CARTESIAN_POINT('Ctrl Pts',(0.420157287975619,-1.,1.85903281096686));
#22686=CARTESIAN_POINT('Ctrl Pts',(0.420157287975619,1.,1.85903281096686));
#22687=CARTESIAN_POINT('Ctrl Pts',(0.422327307418275,-1.,1.86408083334028));
#22688=CARTESIAN_POINT('Ctrl Pts',(0.422327307418275,1.,1.86408083334028));
#22689=CARTESIAN_POINT('Ctrl Pts',(0.424678177291358,-1.,1.86937803944323));
#22690=CARTESIAN_POINT('Ctrl Pts',(0.424678177291358,1.,1.86937803944323));
#22691=CARTESIAN_POINT('Ctrl Pts',(0.427183828519102,-1.,1.87486989291484));
#22692=CARTESIAN_POINT('Ctrl Pts',(0.427183828519102,1.,1.87486989291484));
#22693=CARTESIAN_POINT('Ctrl Pts',(0.429803062482344,-1.,1.88044229001832));
#22694=CARTESIAN_POINT('Ctrl Pts',(0.429803062482344,1.,1.88044229001832));
#22695=CARTESIAN_POINT('Ctrl Pts',(0.432493038548748,-1.,1.88596913666793));
#22696=CARTESIAN_POINT('Ctrl Pts',(0.432493038548748,1.,1.88596913666793));
#22697=CARTESIAN_POINT('Ctrl Pts',(0.435225660963383,-1.,1.89136993975504));
#22698=CARTESIAN_POINT('Ctrl Pts',(0.435225660963383,1.,1.89136993975504));
#22699=CARTESIAN_POINT('Ctrl Pts',(0.437995003948244,-1.,1.89663648956466));
#22700=CARTESIAN_POINT('Ctrl Pts',(0.437995003948244,1.,1.89663648956466));
#22701=CARTESIAN_POINT('Ctrl Pts',(0.440807833704038,-1.,1.90180124389086));
#22702=CARTESIAN_POINT('Ctrl Pts',(0.440807833704038,1.,1.90180124389086));
#22703=CARTESIAN_POINT('Ctrl Pts',(0.44367755684915,-1.,1.90691756144898));
#22704=CARTESIAN_POINT('Ctrl Pts',(0.44367755684915,1.,1.90691756144898));
#22705=CARTESIAN_POINT('Ctrl Pts',(0.446617343485711,-1.,1.9120369998112));
#22706=CARTESIAN_POINT('Ctrl Pts',(0.446617343485711,1.,1.9120369998112));
#22707=CARTESIAN_POINT('Ctrl Pts',(0.449632260106662,-1.,1.91718342555755));
#22708=CARTESIAN_POINT('Ctrl Pts',(0.449632260106662,1.,1.91718342555755));
#22709=CARTESIAN_POINT('Ctrl Pts',(0.452719478359432,-1.,1.92235380648502));
#22710=CARTESIAN_POINT('Ctrl Pts',(0.452719478359432,1.,1.92235380648502));
#22711=CARTESIAN_POINT('Ctrl Pts',(0.45587200517437,-1.,1.92753067150476));
#22712=CARTESIAN_POINT('Ctrl Pts',(0.45587200517437,1.,1.92753067150476));
#22713=CARTESIAN_POINT('Ctrl Pts',(0.459081234547926,-1.,1.93269066517934));
#22714=CARTESIAN_POINT('Ctrl Pts',(0.459081234547926,1.,1.93269066517934));
#22715=CARTESIAN_POINT('Ctrl Pts',(0.462340031009056,-1.,1.93781486640821));
#22716=CARTESIAN_POINT('Ctrl Pts',(0.462340031009056,1.,1.93781486640821));
#22717=CARTESIAN_POINT('Ctrl Pts',(0.46564546202603,-1.,1.9428979419619));
#22718=CARTESIAN_POINT('Ctrl Pts',(0.46564546202603,1.,1.9428979419619));
#22719=CARTESIAN_POINT('Ctrl Pts',(0.468997482913135,-1.,1.94794381136514));
#22720=CARTESIAN_POINT('Ctrl Pts',(0.468997482913135,1.,1.94794381136514));
#22721=CARTESIAN_POINT('Ctrl Pts',(0.472397672264072,-1.,1.95296148278133));
#22722=CARTESIAN_POINT('Ctrl Pts',(0.472397672264072,1.,1.95296148278133));
#22723=CARTESIAN_POINT('Ctrl Pts',(0.475848034683176,-1.,1.95796111148177));
#22724=CARTESIAN_POINT('Ctrl Pts',(0.475848034683176,1.,1.95796111148177));
#22725=CARTESIAN_POINT('Ctrl Pts',(0.479349583074855,-1.,1.96294933055943));
#22726=CARTESIAN_POINT('Ctrl Pts',(0.479349583074855,1.,1.96294933055943));
#22727=CARTESIAN_POINT('Ctrl Pts',(0.48290166212069,-1.,1.96792703422362));
#22728=CARTESIAN_POINT('Ctrl Pts',(0.48290166212069,1.,1.96792703422362));
#22729=CARTESIAN_POINT('Ctrl Pts',(0.486502692907658,-1.,1.97289186263272));
#22730=CARTESIAN_POINT('Ctrl Pts',(0.486502692907658,1.,1.97289186263272));
#22731=CARTESIAN_POINT('Ctrl Pts',(0.490150627860952,-1.,1.97783973019229));
#22732=CARTESIAN_POINT('Ctrl Pts',(0.490150627860952,1.,1.97783973019229));
#22733=CARTESIAN_POINT('Ctrl Pts',(0.493843476541494,-1.,1.98276658761821));
#22734=CARTESIAN_POINT('Ctrl Pts',(0.493843476541494,1.,1.98276658761821));
#22735=CARTESIAN_POINT('Ctrl Pts',(0.497579909545574,-1.,1.98767044752932));
#22736=CARTESIAN_POINT('Ctrl Pts',(0.497579909545574,1.,1.98767044752932));
#22737=CARTESIAN_POINT('Ctrl Pts',(0.501359287727146,-1.,1.99255149126155));
#22738=CARTESIAN_POINT('Ctrl Pts',(0.501359287727146,1.,1.99255149126155));
#22739=CARTESIAN_POINT('Ctrl Pts',(0.505181361323026,-1.,1.99741107463572));
#22740=CARTESIAN_POINT('Ctrl Pts',(0.505181361323026,1.,1.99741107463572));
#22741=CARTESIAN_POINT('Ctrl Pts',(0.509046069886157,-1.,2.00225107134734));
#22742=CARTESIAN_POINT('Ctrl Pts',(0.509046069886157,1.,2.00225107134734));
#22743=CARTESIAN_POINT('Ctrl Pts',(0.512953306961792,-1.,2.00707309946949));
#22744=CARTESIAN_POINT('Ctrl Pts',(0.512953306961792,1.,2.00707309946949));
#22745=CARTESIAN_POINT('Ctrl Pts',(0.516902681728687,-1.,2.01187773939242));
#22746=CARTESIAN_POINT('Ctrl Pts',(0.516902681728687,1.,2.01187773939242));
#22747=CARTESIAN_POINT('Ctrl Pts',(0.52089359039937,-1.,2.01666477917286));
#22748=CARTESIAN_POINT('Ctrl Pts',(0.52089359039937,1.,2.01666477917286));
#22749=CARTESIAN_POINT('Ctrl Pts',(0.524925318333476,-1.,2.02143356304698));
#22750=CARTESIAN_POINT('Ctrl Pts',(0.524925318333476,1.,2.02143356304698));
#22751=CARTESIAN_POINT('Ctrl Pts',(0.528997127241914,-1.,2.0261832908329));
#22752=CARTESIAN_POINT('Ctrl Pts',(0.528997127241914,1.,2.0261832908329));
#22753=CARTESIAN_POINT('Ctrl Pts',(0.533108355132976,-1.,2.03091336214426));
#22754=CARTESIAN_POINT('Ctrl Pts',(0.533108355132976,1.,2.03091336214426));
#22755=CARTESIAN_POINT('Ctrl Pts',(0.537258489833262,-1.,2.03562362954037));
#22756=CARTESIAN_POINT('Ctrl Pts',(0.537258489833262,1.,2.03562362954037));
#22757=CARTESIAN_POINT('Ctrl Pts',(0.541447120615659,-1.,2.04031422690527));
#22758=CARTESIAN_POINT('Ctrl Pts',(0.541447120615659,1.,2.04031422690527));
#22759=CARTESIAN_POINT('Ctrl Pts',(0.54567390381743,-1.,2.04498544714588));
#22760=CARTESIAN_POINT('Ctrl Pts',(0.54567390381743,1.,2.04498544714588));
#22761=CARTESIAN_POINT('Ctrl Pts',(0.549938525150295,-1.,2.04963761077958));
#22762=CARTESIAN_POINT('Ctrl Pts',(0.549938525150295,1.,2.04963761077958));
#22763=CARTESIAN_POINT('Ctrl Pts',(0.554240657463906,-1.,2.05427091604413));
#22764=CARTESIAN_POINT('Ctrl Pts',(0.554240657463906,1.,2.05427091604413));
#22765=CARTESIAN_POINT('Ctrl Pts',(0.558579940185151,-1.,2.05888537756462));
#22766=CARTESIAN_POINT('Ctrl Pts',(0.558579940185151,1.,2.05888537756462));
#22767=CARTESIAN_POINT('Ctrl Pts',(0.562955993082261,-1.,2.06348090160589));
#22768=CARTESIAN_POINT('Ctrl Pts',(0.562955993082261,1.,2.06348090160589));
#22769=CARTESIAN_POINT('Ctrl Pts',(0.567368421181087,-1.,2.06805732997334));
#22770=CARTESIAN_POINT('Ctrl Pts',(0.567368421181087,1.,2.06805732997334));
#22771=CARTESIAN_POINT('Ctrl Pts',(0.571816823242602,-1.,2.07261449292824));
#22772=CARTESIAN_POINT('Ctrl Pts',(0.571816823242602,1.,2.07261449292824));
#22773=CARTESIAN_POINT('Ctrl Pts',(0.576300797416844,-1.,2.07715226767559));
#22774=CARTESIAN_POINT('Ctrl Pts',(0.576300797416844,1.,2.07715226767559));
#22775=CARTESIAN_POINT('Ctrl Pts',(0.580819952108063,-1.,2.08167059018418));
#22776=CARTESIAN_POINT('Ctrl Pts',(0.580819952108063,1.,2.08167059018418));
#22777=CARTESIAN_POINT('Ctrl Pts',(0.585373918991617,-1.,2.08616943727951));
#22778=CARTESIAN_POINT('Ctrl Pts',(0.585373918991617,1.,2.08616943727951));
#22779=CARTESIAN_POINT('Ctrl Pts',(0.589962365403406,-1.,2.09064881812129));
#22780=CARTESIAN_POINT('Ctrl Pts',(0.589962365403406,1.,2.09064881812129));
#22781=CARTESIAN_POINT('Ctrl Pts',(0.594585006052162,-1.,2.0951087622027));
#22782=CARTESIAN_POINT('Ctrl Pts',(0.594585006052162,1.,2.0951087622027));
#22783=CARTESIAN_POINT('Ctrl Pts',(0.599241616420533,-1.,2.0995493086477));
#22784=CARTESIAN_POINT('Ctrl Pts',(0.599241616420533,1.,2.0995493086477));
#22785=CARTESIAN_POINT('Ctrl Pts',(0.60393203073603,-1.,2.10397049886949));
#22786=CARTESIAN_POINT('Ctrl Pts',(0.60393203073603,1.,2.10397049886949));
#22787=CARTESIAN_POINT('Ctrl Pts',(0.607711315454876,-1.,2.1074919961518));
#22788=CARTESIAN_POINT('Ctrl Pts',(0.607711315454876,1.,2.1074919961518));
#22789=CARTESIAN_POINT('Ctrl Pts',(0.610560911689898,-1.,2.11012443807238));
#22790=CARTESIAN_POINT('Ctrl Pts',(0.610560911689898,1.,2.11012443807238));
#22791=CARTESIAN_POINT('Ctrl Pts',(0.6124673655618,-1.,2.11187554259986));
#22792=CARTESIAN_POINT('Ctrl Pts',(0.6124673655618,1.,2.11187554259986));
#22793=CARTESIAN_POINT('Ctrl Pts',(0.61342227326009,-1.,2.11275013067528));
#22794=CARTESIAN_POINT('Ctrl Pts',(0.61342227326009,1.,2.11275013067528));
#22795=CARTESIAN_POINT('',(0.383122945602004,1.,1.7075470150345));
#22796=CARTESIAN_POINT('Ctrl Pts',(0.383122945602004,1.,1.7075470150345));
#22797=CARTESIAN_POINT('Ctrl Pts',(0.384119047315541,1.,1.71231062891958));
#22798=CARTESIAN_POINT('Ctrl Pts',(0.38607079032701,1.,1.72162022246158));
#22799=CARTESIAN_POINT('Ctrl Pts',(0.388877023509191,1.,1.7349317097561));
#22800=CARTESIAN_POINT('Ctrl Pts',(0.392375812294307,1.,1.75137405313962));
#22801=CARTESIAN_POINT('Ctrl Pts',(0.39634619612042,1.,1.7697556004756));
#22802=CARTESIAN_POINT('Ctrl Pts',(0.39991940378308,1.,1.78598826347533));
#22803=CARTESIAN_POINT('Ctrl Pts',(0.403107976170441,1.,1.80012077176221));
#22804=CARTESIAN_POINT('Ctrl Pts',(0.405933518411838,1.,1.81223801813988));
#22805=CARTESIAN_POINT('Ctrl Pts',(0.408428948108533,1.,1.8224702267854));
#22806=CARTESIAN_POINT('Ctrl Pts',(0.410641256301674,1.,1.83100408895216));
#22807=CARTESIAN_POINT('Ctrl Pts',(0.412633125322161,1.,1.83808953475839));
#22808=CARTESIAN_POINT('Ctrl Pts',(0.41448743825434,1.,1.8440575707371));
#22809=CARTESIAN_POINT('Ctrl Pts',(0.416300022038864,1.,1.84929312929882));
#22810=CARTESIAN_POINT('Ctrl Pts',(0.418164129143534,1.,1.85417632856234));
#22811=CARTESIAN_POINT('Ctrl Pts',(0.420157287975619,1.,1.85903281096686));
#22812=CARTESIAN_POINT('Ctrl Pts',(0.422327307418275,1.,1.86408083334028));
#22813=CARTESIAN_POINT('Ctrl Pts',(0.424678177291358,1.,1.86937803944323));
#22814=CARTESIAN_POINT('Ctrl Pts',(0.427183828519102,1.,1.87486989291484));
#22815=CARTESIAN_POINT('Ctrl Pts',(0.429803062482344,1.,1.88044229001832));
#22816=CARTESIAN_POINT('Ctrl Pts',(0.432493038548748,1.,1.88596913666793));
#22817=CARTESIAN_POINT('Ctrl Pts',(0.435225660963383,1.,1.89136993975504));
#22818=CARTESIAN_POINT('Ctrl Pts',(0.437995003948244,1.,1.89663648956466));
#22819=CARTESIAN_POINT('Ctrl Pts',(0.440807833704038,1.,1.90180124389086));
#22820=CARTESIAN_POINT('Ctrl Pts',(0.44367755684915,1.,1.90691756144898));
#22821=CARTESIAN_POINT('Ctrl Pts',(0.446617343485711,1.,1.9120369998112));
#22822=CARTESIAN_POINT('Ctrl Pts',(0.449632260106662,1.,1.91718342555755));
#22823=CARTESIAN_POINT('Ctrl Pts',(0.452719478359432,1.,1.92235380648502));
#22824=CARTESIAN_POINT('Ctrl Pts',(0.45587200517437,1.,1.92753067150476));
#22825=CARTESIAN_POINT('Ctrl Pts',(0.459081234547926,1.,1.93269066517934));
#22826=CARTESIAN_POINT('Ctrl Pts',(0.462340031009056,1.,1.93781486640821));
#22827=CARTESIAN_POINT('Ctrl Pts',(0.46564546202603,1.,1.9428979419619));
#22828=CARTESIAN_POINT('Ctrl Pts',(0.468997482913135,1.,1.94794381136514));
#22829=CARTESIAN_POINT('Ctrl Pts',(0.472397672264072,1.,1.95296148278133));
#22830=CARTESIAN_POINT('Ctrl Pts',(0.475848034683176,1.,1.95796111148177));
#22831=CARTESIAN_POINT('Ctrl Pts',(0.479349583074855,1.,1.96294933055943));
#22832=CARTESIAN_POINT('Ctrl Pts',(0.48290166212069,1.,1.96792703422362));
#22833=CARTESIAN_POINT('Ctrl Pts',(0.486502692907658,1.,1.97289186263272));
#22834=CARTESIAN_POINT('Ctrl Pts',(0.490150627860952,1.,1.97783973019229));
#22835=CARTESIAN_POINT('Ctrl Pts',(0.493843476541494,1.,1.98276658761821));
#22836=CARTESIAN_POINT('Ctrl Pts',(0.497579909545574,1.,1.98767044752932));
#22837=CARTESIAN_POINT('Ctrl Pts',(0.501359287727146,1.,1.99255149126155));
#22838=CARTESIAN_POINT('Ctrl Pts',(0.505181361323026,1.,1.99741107463572));
#22839=CARTESIAN_POINT('Ctrl Pts',(0.509046069886157,1.,2.00225107134734));
#22840=CARTESIAN_POINT('Ctrl Pts',(0.512953306961792,1.,2.00707309946949));
#22841=CARTESIAN_POINT('Ctrl Pts',(0.516902681728687,1.,2.01187773939242));
#22842=CARTESIAN_POINT('Ctrl Pts',(0.52089359039937,1.,2.01666477917286));
#22843=CARTESIAN_POINT('Ctrl Pts',(0.524925318333476,1.,2.02143356304698));
#22844=CARTESIAN_POINT('Ctrl Pts',(0.528997127241914,1.,2.0261832908329));
#22845=CARTESIAN_POINT('Ctrl Pts',(0.533108355132976,1.,2.03091336214426));
#22846=CARTESIAN_POINT('Ctrl Pts',(0.537258489833262,1.,2.03562362954037));
#22847=CARTESIAN_POINT('Ctrl Pts',(0.541447120615659,1.,2.04031422690527));
#22848=CARTESIAN_POINT('Ctrl Pts',(0.54567390381743,1.,2.04498544714588));
#22849=CARTESIAN_POINT('Ctrl Pts',(0.549938525150295,1.,2.04963761077958));
#22850=CARTESIAN_POINT('Ctrl Pts',(0.554240657463906,1.,2.05427091604413));
#22851=CARTESIAN_POINT('Ctrl Pts',(0.558579940185151,1.,2.05888537756462));
#22852=CARTESIAN_POINT('Ctrl Pts',(0.562955993082261,1.,2.06348090160589));
#22853=CARTESIAN_POINT('Ctrl Pts',(0.567368421181087,1.,2.06805732997334));
#22854=CARTESIAN_POINT('Ctrl Pts',(0.571816823242602,1.,2.07261449292824));
#22855=CARTESIAN_POINT('Ctrl Pts',(0.576300797416844,1.,2.07715226767559));
#22856=CARTESIAN_POINT('Ctrl Pts',(0.580819952108063,1.,2.08167059018418));
#22857=CARTESIAN_POINT('Ctrl Pts',(0.585373918991617,1.,2.08616943727951));
#22858=CARTESIAN_POINT('Ctrl Pts',(0.589962365403406,1.,2.09064881812129));
#22859=CARTESIAN_POINT('Ctrl Pts',(0.594585006052162,1.,2.0951087622027));
#22860=CARTESIAN_POINT('Ctrl Pts',(0.599241616420533,1.,2.0995493086477));
#22861=CARTESIAN_POINT('Ctrl Pts',(0.60393203073603,1.,2.10397049886949));
#22862=CARTESIAN_POINT('Ctrl Pts',(0.607711315454876,1.,2.1074919961518));
#22863=CARTESIAN_POINT('Ctrl Pts',(0.610560911689898,1.,2.11012443807238));
#22864=CARTESIAN_POINT('Ctrl Pts',(0.6124673655618,1.,2.11187554259986));
#22865=CARTESIAN_POINT('Ctrl Pts',(0.61342227326009,1.,2.11275013067528));
#22866=CARTESIAN_POINT('',(0.383122945602003,0.,1.7075470150345));
#22867=CARTESIAN_POINT('Origin',(0.,0.,0.));
#22868=CARTESIAN_POINT('',(0.163289472382896,1.,1.74236521665491));
#22869=CARTESIAN_POINT('Origin',(0.,1.,0.));
#22870=CARTESIAN_POINT('',(0.163289472382896,0.,1.74236521665491));
#22871=CARTESIAN_POINT('Ctrl Pts',(0.0694764450219578,-1.,2.19890268624765));
#22872=CARTESIAN_POINT('Ctrl Pts',(0.0694764450219578,1.,2.19890268624765));
#22873=CARTESIAN_POINT('Ctrl Pts',(0.0701143536325487,-1.,2.19777582085423));
#22874=CARTESIAN_POINT('Ctrl Pts',(0.0701143536325487,1.,2.19777582085423));
#22875=CARTESIAN_POINT('Ctrl Pts',(0.0713863779526151,-1.,2.19552129484002));
#22876=CARTESIAN_POINT('Ctrl Pts',(0.0713863779526151,1.,2.19552129484002));
#22877=CARTESIAN_POINT('Ctrl Pts',(0.0732830357306722,-1.,2.19213712013662));
#22878=CARTESIAN_POINT('Ctrl Pts',(0.0732830357306722,1.,2.19213712013662));
#22879=CARTESIAN_POINT('Ctrl Pts',(0.0757891465836145,-1.,2.1876201139953));
#22880=CARTESIAN_POINT('Ctrl Pts',(0.0757891465836145,1.,2.1876201139953));
#22881=CARTESIAN_POINT('Ctrl Pts',(0.078883772768524,-1.,2.18196589448887));
#22882=CARTESIAN_POINT('Ctrl Pts',(0.078883772768524,1.,2.18196589448887));
#22883=CARTESIAN_POINT('Ctrl Pts',(0.0819402680872763,-1.,2.176303712113));
#22884=CARTESIAN_POINT('Ctrl Pts',(0.0819402680872763,1.,2.176303712113));
#22885=CARTESIAN_POINT('Ctrl Pts',(0.084958462083537,-1.,2.17063357870952));
#22886=CARTESIAN_POINT('Ctrl Pts',(0.084958462083537,1.,2.17063357870952));
#22887=CARTESIAN_POINT('Ctrl Pts',(0.087938129138692,-1.,2.16495552645014));
#22888=CARTESIAN_POINT('Ctrl Pts',(0.087938129138692,1.,2.16495552645014));
#22889=CARTESIAN_POINT('Ctrl Pts',(0.0908789888107263,-1.,2.15926961544516));
#22890=CARTESIAN_POINT('Ctrl Pts',(0.0908789888107263,1.,2.15926961544516));
#22891=CARTESIAN_POINT('Ctrl Pts',(0.0937807218867641,-1.,2.1535759397817));
#22892=CARTESIAN_POINT('Ctrl Pts',(0.0937807218867641,1.,2.1535759397817));
#22893=CARTESIAN_POINT('Ctrl Pts',(0.0966429852305456,-1.,2.14787463531795));
#22894=CARTESIAN_POINT('Ctrl Pts',(0.0966429852305456,1.,2.14787463531795));
#22895=CARTESIAN_POINT('Ctrl Pts',(0.0994654261990913,-1.,2.14216588396025));
#22896=CARTESIAN_POINT('Ctrl Pts',(0.0994654261990913,1.,2.14216588396025));
#22897=CARTESIAN_POINT('Ctrl Pts',(0.1022477005561,-1.,2.13644992667165));
#22898=CARTESIAN_POINT('Ctrl Pts',(0.1022477005561,1.,2.13644992667165));
#22899=CARTESIAN_POINT('Ctrl Pts',(0.104989479152739,-1.,2.13072704887293));
#22900=CARTESIAN_POINT('Ctrl Pts',(0.104989479152739,1.,2.13072704887293));
#22901=CARTESIAN_POINT('Ctrl Pts',(0.10769043523109,-1.,2.12499752307));
#22902=CARTESIAN_POINT('Ctrl Pts',(0.10769043523109,1.,2.12499752307));
#22903=CARTESIAN_POINT('Ctrl Pts',(0.110350236135025,-1.,2.11926155590865));
#22904=CARTESIAN_POINT('Ctrl Pts',(0.110350236135025,1.,2.11926155590865));
#22905=CARTESIAN_POINT('Ctrl Pts',(0.112968534419737,-1.,2.11351924490306));
#22906=CARTESIAN_POINT('Ctrl Pts',(0.112968534419737,1.,2.11351924490306));
#22907=CARTESIAN_POINT('Ctrl Pts',(0.115544957687926,-1.,2.10777050261309));
#22908=CARTESIAN_POINT('Ctrl Pts',(0.115544957687926,1.,2.10777050261309));
#22909=CARTESIAN_POINT('Ctrl Pts',(0.118079107988355,-1.,2.102015121329));
#22910=CARTESIAN_POINT('Ctrl Pts',(0.118079107988355,1.,2.102015121329));
#22911=CARTESIAN_POINT('Ctrl Pts',(0.120570567965122,-1.,2.0962529286773));
#22912=CARTESIAN_POINT('Ctrl Pts',(0.120570567965122,1.,2.0962529286773));
#22913=CARTESIAN_POINT('Ctrl Pts',(0.123018905621083,-1.,2.09048392424825));
#22914=CARTESIAN_POINT('Ctrl Pts',(0.123018905621083,1.,2.09048392424825));
#22915=CARTESIAN_POINT('Ctrl Pts',(0.125423679412061,-1.,2.08470840653643));
#22916=CARTESIAN_POINT('Ctrl Pts',(0.125423679412061,1.,2.08470840653643));
#22917=CARTESIAN_POINT('Ctrl Pts',(0.12778444527612,-1.,2.07892715110987));
#22918=CARTESIAN_POINT('Ctrl Pts',(0.12778444527612,1.,2.07892715110987));
#22919=CARTESIAN_POINT('Ctrl Pts',(0.130100748328403,-1.,2.07314114713063));
#22920=CARTESIAN_POINT('Ctrl Pts',(0.130100748328403,1.,2.07314114713063));
#22921=CARTESIAN_POINT('Ctrl Pts',(0.13237211154771,-1.,2.06735123910326));
#22922=CARTESIAN_POINT('Ctrl Pts',(0.13237211154771,1.,2.06735123910326));
#22923=CARTESIAN_POINT('Ctrl Pts',(0.134598026192106,-1.,2.06155781517842));
#22924=CARTESIAN_POINT('Ctrl Pts',(0.134598026192106,1.,2.06155781517842));
#22925=CARTESIAN_POINT('Ctrl Pts',(0.136777941218043,-1.,2.05576044414264));
#22926=CARTESIAN_POINT('Ctrl Pts',(0.136777941218043,1.,2.05576044414264));
#22927=CARTESIAN_POINT('Ctrl Pts',(0.138911255368966,-1.,2.04995762001328));
#22928=CARTESIAN_POINT('Ctrl Pts',(0.138911255368966,1.,2.04995762001328));
#22929=CARTESIAN_POINT('Ctrl Pts',(0.140997332152546,-1.,2.04414757947916));
#22930=CARTESIAN_POINT('Ctrl Pts',(0.140997332152546,1.,2.04414757947916));
#22931=CARTESIAN_POINT('Ctrl Pts',(0.143035515058208,-1.,2.03832911025912));
#22932=CARTESIAN_POINT('Ctrl Pts',(0.143035515058208,1.,2.03832911025912));
#22933=CARTESIAN_POINT('Ctrl Pts',(0.145025140186057,-1.,2.03250223739942));
#22934=CARTESIAN_POINT('Ctrl Pts',(0.145025140186057,1.,2.03250223739942));
#22935=CARTESIAN_POINT('Ctrl Pts',(0.146965557332583,-1.,2.02666926182017));
#22936=CARTESIAN_POINT('Ctrl Pts',(0.146965557332583,1.,2.02666926182017));
#22937=CARTESIAN_POINT('Ctrl Pts',(0.148856124775337,-1.,2.02083464969894));
#22938=CARTESIAN_POINT('Ctrl Pts',(0.148856124775337,1.,2.02083464969894));
#22939=CARTESIAN_POINT('Ctrl Pts',(0.150696157673078,-1.,2.01500291940238));
#22940=CARTESIAN_POINT('Ctrl Pts',(0.150696157673078,1.,2.01500291940238));
#22941=CARTESIAN_POINT('Ctrl Pts',(0.152484883621449,-1.,2.00917680318424));
#22942=CARTESIAN_POINT('Ctrl Pts',(0.152484883621449,1.,2.00917680318424));
#22943=CARTESIAN_POINT('Ctrl Pts',(0.154221403049722,-1.,2.00335565310543));
#22944=CARTESIAN_POINT('Ctrl Pts',(0.154221403049722,1.,2.00335565310543));
#22945=CARTESIAN_POINT('Ctrl Pts',(0.155904629548783,-1.,1.99753284771497));
#22946=CARTESIAN_POINT('Ctrl Pts',(0.155904629548783,1.,1.99753284771497));
#22947=CARTESIAN_POINT('Ctrl Pts',(0.157533331459227,-1.,1.99169810931908));
#22948=CARTESIAN_POINT('Ctrl Pts',(0.157533331459227,1.,1.99169810931908));
#22949=CARTESIAN_POINT('Ctrl Pts',(0.159106226437299,-1.,1.98584238283292));
#22950=CARTESIAN_POINT('Ctrl Pts',(0.159106226437299,1.,1.98584238283292));
#22951=CARTESIAN_POINT('Ctrl Pts',(0.160622060784611,-1.,1.97996195437559));
#22952=CARTESIAN_POINT('Ctrl Pts',(0.160622060784611,1.,1.97996195437559));
#22953=CARTESIAN_POINT('Ctrl Pts',(0.162079693556288,-1.,1.97406280235188));
#22954=CARTESIAN_POINT('Ctrl Pts',(0.162079693556288,1.,1.97406280235188));
#22955=CARTESIAN_POINT('Ctrl Pts',(0.163478185457734,-1.,1.96816512677967));
#22956=CARTESIAN_POINT('Ctrl Pts',(0.163478185457734,1.,1.96816512677967));
#22957=CARTESIAN_POINT('Ctrl Pts',(0.164816568920269,-1.,1.96229379940136));
#22958=CARTESIAN_POINT('Ctrl Pts',(0.164816568920269,1.,1.96229379940136));
#22959=CARTESIAN_POINT('Ctrl Pts',(0.166093592002812,-1.,1.9564675971873));
#22960=CARTESIAN_POINT('Ctrl Pts',(0.166093592002812,1.,1.9564675971873));
#22961=CARTESIAN_POINT('Ctrl Pts',(0.167307501784475,-1.,1.95069027794294));
#22962=CARTESIAN_POINT('Ctrl Pts',(0.167307501784475,1.,1.95069027794294));
#22963=CARTESIAN_POINT('Ctrl Pts',(0.168455741607556,-1.,1.94493757756931));
#22964=CARTESIAN_POINT('Ctrl Pts',(0.168455741607556,1.,1.94493757756931));
#22965=CARTESIAN_POINT('Ctrl Pts',(0.16953490481749,-1.,1.93915639211581));
#22966=CARTESIAN_POINT('Ctrl Pts',(0.16953490481749,1.,1.93915639211581));
#22967=CARTESIAN_POINT('Ctrl Pts',(0.170541253116201,-1.,1.93329183155539));
#22968=CARTESIAN_POINT('Ctrl Pts',(0.170541253116201,1.,1.93329183155539));
#22969=CARTESIAN_POINT('Ctrl Pts',(0.171471191532988,-1.,1.92731093582036));
#22970=CARTESIAN_POINT('Ctrl Pts',(0.171471191532988,1.,1.92731093582036));
#22971=CARTESIAN_POINT('Ctrl Pts',(0.172321621259513,-1.,1.9212233439798));
#22972=CARTESIAN_POINT('Ctrl Pts',(0.172321621259513,1.,1.9212233439798));
#22973=CARTESIAN_POINT('Ctrl Pts',(0.173090695383496,-1.,1.91511429159527));
#22974=CARTESIAN_POINT('Ctrl Pts',(0.173090695383496,1.,1.91511429159527));
#22975=CARTESIAN_POINT('Ctrl Pts',(0.173776635257816,-1.,1.90911693975267));
#22976=CARTESIAN_POINT('Ctrl Pts',(0.173776635257816,1.,1.90911693975267));
#22977=CARTESIAN_POINT('Ctrl Pts',(0.174375518661085,-1.,1.90335253862834));
#22978=CARTESIAN_POINT('Ctrl Pts',(0.174375518661085,1.,1.90335253862834));
#22979=CARTESIAN_POINT('Ctrl Pts',(0.174879405091263,-1.,1.89788101117132));
#22980=CARTESIAN_POINT('Ctrl Pts',(0.174879405091263,1.,1.89788101117132));
#22981=CARTESIAN_POINT('Ctrl Pts',(0.175274276190844,-1.,1.892646301985));
#22982=CARTESIAN_POINT('Ctrl Pts',(0.175274276190844,1.,1.892646301985));
#22983=CARTESIAN_POINT('Ctrl Pts',(0.175538155840648,-1.,1.88742606273259));
#22984=CARTESIAN_POINT('Ctrl Pts',(0.175538155840648,1.,1.88742606273259));
#22985=CARTESIAN_POINT('Ctrl Pts',(0.175644148889698,-1.,1.88188663145367));
#22986=CARTESIAN_POINT('Ctrl Pts',(0.175644148889698,1.,1.88188663145367));
#22987=CARTESIAN_POINT('Ctrl Pts',(0.175563480746485,-1.,1.87563767773588));
#22988=CARTESIAN_POINT('Ctrl Pts',(0.175563480746485,1.,1.87563767773588));
#22989=CARTESIAN_POINT('Ctrl Pts',(0.175268337590757,-1.,1.86828349694799));
#22990=CARTESIAN_POINT('Ctrl Pts',(0.175268337590757,1.,1.86828349694799));
#22991=CARTESIAN_POINT('Ctrl Pts',(0.17473525927603,-1.,1.85948367088837));
#22992=CARTESIAN_POINT('Ctrl Pts',(0.17473525927603,1.,1.85948367088837));
#22993=CARTESIAN_POINT('Ctrl Pts',(0.173946627587731,-1.,1.8489811319852));
#22994=CARTESIAN_POINT('Ctrl Pts',(0.173946627587731,1.,1.8489811319852));
#22995=CARTESIAN_POINT('Ctrl Pts',(0.1728894428919,-1.,1.83658380527692));
#22996=CARTESIAN_POINT('Ctrl Pts',(0.1728894428919,1.,1.83658380527692));
#22997=CARTESIAN_POINT('Ctrl Pts',(0.171554770204119,-1.,1.82215766811545));
#22998=CARTESIAN_POINT('Ctrl Pts',(0.171554770204119,1.,1.82215766811545));
#22999=CARTESIAN_POINT('Ctrl Pts',(0.169936923904608,-1.,1.80561530629706));
#23000=CARTESIAN_POINT('Ctrl Pts',(0.169936923904608,1.,1.80561530629706));
#23001=CARTESIAN_POINT('Ctrl Pts',(0.168032772805197,-1.,1.7869064998507));
#23002=CARTESIAN_POINT('Ctrl Pts',(0.168032772805197,1.,1.7869064998507));
#23003=CARTESIAN_POINT('Ctrl Pts',(0.1662793551464,-1.,1.77018771684844));
#23004=CARTESIAN_POINT('Ctrl Pts',(0.1662793551464,1.,1.77018771684844));
#23005=CARTESIAN_POINT('Ctrl Pts',(0.164834765707158,-1.,1.75666056638427));
#23006=CARTESIAN_POINT('Ctrl Pts',(0.164834765707158,1.,1.75666056638427));
#23007=CARTESIAN_POINT('Ctrl Pts',(0.163814161002002,-1.,1.7472034950333));
#23008=CARTESIAN_POINT('Ctrl Pts',(0.163814161002002,1.,1.7472034950333));
#23009=CARTESIAN_POINT('Ctrl Pts',(0.163289472382896,-1.,1.74236521665491));
#23010=CARTESIAN_POINT('Ctrl Pts',(0.163289472382896,1.,1.74236521665491));
#23011=CARTESIAN_POINT('',(0.0694764450219578,1.,2.19890268624765));
#23012=CARTESIAN_POINT('Ctrl Pts',(0.0694764450219578,1.,2.19890268624765));
#23013=CARTESIAN_POINT('Ctrl Pts',(0.0701143536325487,1.,2.19777582085423));
#23014=CARTESIAN_POINT('Ctrl Pts',(0.0713863779526151,1.,2.19552129484002));
#23015=CARTESIAN_POINT('Ctrl Pts',(0.0732830357306722,1.,2.19213712013662));
#23016=CARTESIAN_POINT('Ctrl Pts',(0.0757891465836145,1.,2.1876201139953));
#23017=CARTESIAN_POINT('Ctrl Pts',(0.078883772768524,1.,2.18196589448887));
#23018=CARTESIAN_POINT('Ctrl Pts',(0.0819402680872763,1.,2.176303712113));
#23019=CARTESIAN_POINT('Ctrl Pts',(0.084958462083537,1.,2.17063357870952));
#23020=CARTESIAN_POINT('Ctrl Pts',(0.087938129138692,1.,2.16495552645014));
#23021=CARTESIAN_POINT('Ctrl Pts',(0.0908789888107263,1.,2.15926961544516));
#23022=CARTESIAN_POINT('Ctrl Pts',(0.0937807218867641,1.,2.1535759397817));
#23023=CARTESIAN_POINT('Ctrl Pts',(0.0966429852305456,1.,2.14787463531795));
#23024=CARTESIAN_POINT('Ctrl Pts',(0.0994654261990913,1.,2.14216588396025));
#23025=CARTESIAN_POINT('Ctrl Pts',(0.1022477005561,1.,2.13644992667165));
#23026=CARTESIAN_POINT('Ctrl Pts',(0.104989479152739,1.,2.13072704887293));
#23027=CARTESIAN_POINT('Ctrl Pts',(0.10769043523109,1.,2.12499752307));
#23028=CARTESIAN_POINT('Ctrl Pts',(0.110350236135025,1.,2.11926155590865));
#23029=CARTESIAN_POINT('Ctrl Pts',(0.112968534419737,1.,2.11351924490306));
#23030=CARTESIAN_POINT('Ctrl Pts',(0.115544957687926,1.,2.10777050261309));
#23031=CARTESIAN_POINT('Ctrl Pts',(0.118079107988355,1.,2.102015121329));
#23032=CARTESIAN_POINT('Ctrl Pts',(0.120570567965122,1.,2.0962529286773));
#23033=CARTESIAN_POINT('Ctrl Pts',(0.123018905621083,1.,2.09048392424825));
#23034=CARTESIAN_POINT('Ctrl Pts',(0.125423679412061,1.,2.08470840653643));
#23035=CARTESIAN_POINT('Ctrl Pts',(0.12778444527612,1.,2.07892715110987));
#23036=CARTESIAN_POINT('Ctrl Pts',(0.130100748328403,1.,2.07314114713063));
#23037=CARTESIAN_POINT('Ctrl Pts',(0.13237211154771,1.,2.06735123910326));
#23038=CARTESIAN_POINT('Ctrl Pts',(0.134598026192106,1.,2.06155781517842));
#23039=CARTESIAN_POINT('Ctrl Pts',(0.136777941218043,1.,2.05576044414264));
#23040=CARTESIAN_POINT('Ctrl Pts',(0.138911255368966,1.,2.04995762001328));
#23041=CARTESIAN_POINT('Ctrl Pts',(0.140997332152546,1.,2.04414757947916));
#23042=CARTESIAN_POINT('Ctrl Pts',(0.143035515058208,1.,2.03832911025912));
#23043=CARTESIAN_POINT('Ctrl Pts',(0.145025140186057,1.,2.03250223739942));
#23044=CARTESIAN_POINT('Ctrl Pts',(0.146965557332583,1.,2.02666926182017));
#23045=CARTESIAN_POINT('Ctrl Pts',(0.148856124775337,1.,2.02083464969894));
#23046=CARTESIAN_POINT('Ctrl Pts',(0.150696157673078,1.,2.01500291940238));
#23047=CARTESIAN_POINT('Ctrl Pts',(0.152484883621449,1.,2.00917680318424));
#23048=CARTESIAN_POINT('Ctrl Pts',(0.154221403049722,1.,2.00335565310543));
#23049=CARTESIAN_POINT('Ctrl Pts',(0.155904629548783,1.,1.99753284771497));
#23050=CARTESIAN_POINT('Ctrl Pts',(0.157533331459227,1.,1.99169810931908));
#23051=CARTESIAN_POINT('Ctrl Pts',(0.159106226437299,1.,1.98584238283292));
#23052=CARTESIAN_POINT('Ctrl Pts',(0.160622060784611,1.,1.97996195437559));
#23053=CARTESIAN_POINT('Ctrl Pts',(0.162079693556288,1.,1.97406280235188));
#23054=CARTESIAN_POINT('Ctrl Pts',(0.163478185457734,1.,1.96816512677967));
#23055=CARTESIAN_POINT('Ctrl Pts',(0.164816568920269,1.,1.96229379940136));
#23056=CARTESIAN_POINT('Ctrl Pts',(0.166093592002812,1.,1.9564675971873));
#23057=CARTESIAN_POINT('Ctrl Pts',(0.167307501784475,1.,1.95069027794294));
#23058=CARTESIAN_POINT('Ctrl Pts',(0.168455741607556,1.,1.94493757756931));
#23059=CARTESIAN_POINT('Ctrl Pts',(0.16953490481749,1.,1.93915639211581));
#23060=CARTESIAN_POINT('Ctrl Pts',(0.170541253116201,1.,1.93329183155539));
#23061=CARTESIAN_POINT('Ctrl Pts',(0.171471191532988,1.,1.92731093582036));
#23062=CARTESIAN_POINT('Ctrl Pts',(0.172321621259513,1.,1.9212233439798));
#23063=CARTESIAN_POINT('Ctrl Pts',(0.173090695383496,1.,1.91511429159527));
#23064=CARTESIAN_POINT('Ctrl Pts',(0.173776635257816,1.,1.90911693975267));
#23065=CARTESIAN_POINT('Ctrl Pts',(0.174375518661085,1.,1.90335253862834));
#23066=CARTESIAN_POINT('Ctrl Pts',(0.174879405091263,1.,1.89788101117132));
#23067=CARTESIAN_POINT('Ctrl Pts',(0.175274276190844,1.,1.892646301985));
#23068=CARTESIAN_POINT('Ctrl Pts',(0.175538155840648,1.,1.88742606273259));
#23069=CARTESIAN_POINT('Ctrl Pts',(0.175644148889698,1.,1.88188663145367));
#23070=CARTESIAN_POINT('Ctrl Pts',(0.175563480746485,1.,1.87563767773588));
#23071=CARTESIAN_POINT('Ctrl Pts',(0.175268337590757,1.,1.86828349694799));
#23072=CARTESIAN_POINT('Ctrl Pts',(0.17473525927603,1.,1.85948367088837));
#23073=CARTESIAN_POINT('Ctrl Pts',(0.173946627587731,1.,1.8489811319852));
#23074=CARTESIAN_POINT('Ctrl Pts',(0.1728894428919,1.,1.83658380527692));
#23075=CARTESIAN_POINT('Ctrl Pts',(0.171554770204119,1.,1.82215766811545));
#23076=CARTESIAN_POINT('Ctrl Pts',(0.169936923904608,1.,1.80561530629706));
#23077=CARTESIAN_POINT('Ctrl Pts',(0.168032772805197,1.,1.7869064998507));
#23078=CARTESIAN_POINT('Ctrl Pts',(0.1662793551464,1.,1.77018771684844));
#23079=CARTESIAN_POINT('Ctrl Pts',(0.164834765707158,1.,1.75666056638427));
#23080=CARTESIAN_POINT('Ctrl Pts',(0.163814161002002,1.,1.7472034950333));
#23081=CARTESIAN_POINT('Ctrl Pts',(0.163289472382896,1.,1.74236521665491));
#23082=CARTESIAN_POINT('',(0.0694764450219578,0.,2.19890268624765));
#23083=CARTESIAN_POINT('Origin',(-0.0694764450219586,0.,2.19890268624765));
#23084=CARTESIAN_POINT('',(-0.0694764450219586,1.,2.19890268624765));
#23085=CARTESIAN_POINT('',(0.0694764450219578,1.,2.19890268624765));
#23086=CARTESIAN_POINT('',(-0.0694764450219586,0.,2.19890268624765));
#23087=CARTESIAN_POINT('Ctrl Pts',(-0.163289472382896,-1.,1.74236521665491));
#23088=CARTESIAN_POINT('Ctrl Pts',(-0.163289472382896,1.,1.74236521665491));
#23089=CARTESIAN_POINT('Ctrl Pts',(-0.163814161002474,-1.,1.74720349503904));
#23090=CARTESIAN_POINT('Ctrl Pts',(-0.163814161002474,1.,1.74720349503904));
#23091=CARTESIAN_POINT('Ctrl Pts',(-0.164834765708484,-1.,1.75666056640041));
#23092=CARTESIAN_POINT('Ctrl Pts',(-0.164834765708484,1.,1.75666056640041));
#23093=CARTESIAN_POINT('Ctrl Pts',(-0.166279355148738,-1.,1.77018771687692));
#23094=CARTESIAN_POINT('Ctrl Pts',(-0.166279355148738,1.,1.77018771687692));
#23095=CARTESIAN_POINT('Ctrl Pts',(-0.16803277280837,-1.,1.78690649988931));
#23096=CARTESIAN_POINT('Ctrl Pts',(-0.16803277280837,1.,1.78690649988931));
#23097=CARTESIAN_POINT('Ctrl Pts',(-0.169936923908078,-1.,1.80561530633924));
#23098=CARTESIAN_POINT('Ctrl Pts',(-0.169936923908078,1.,1.80561530633924));
#23099=CARTESIAN_POINT('Ctrl Pts',(-0.171554770207306,-1.,1.82215766815414));
#23100=CARTESIAN_POINT('Ctrl Pts',(-0.171554770207306,1.,1.82215766815414));
#23101=CARTESIAN_POINT('Ctrl Pts',(-0.17288944289442,-1.,1.83658380530747));
#23102=CARTESIAN_POINT('Ctrl Pts',(-0.17288944289442,1.,1.83658380530747));
#23103=CARTESIAN_POINT('Ctrl Pts',(-0.173946627589401,-1.,1.84898113200543));
#23104=CARTESIAN_POINT('Ctrl Pts',(-0.173946627589401,1.,1.84898113200543));
#23105=CARTESIAN_POINT('Ctrl Pts',(-0.174735259276856,-1.,1.85948367089838));
#23106=CARTESIAN_POINT('Ctrl Pts',(-0.174735259276856,1.,1.85948367089838));
#23107=CARTESIAN_POINT('Ctrl Pts',(-0.175268337590901,-1.,1.86828349694972));
#23108=CARTESIAN_POINT('Ctrl Pts',(-0.175268337590901,1.,1.86828349694972));
#23109=CARTESIAN_POINT('Ctrl Pts',(-0.175563480746206,-1.,1.87563767773249));
#23110=CARTESIAN_POINT('Ctrl Pts',(-0.175563480746206,1.,1.87563767773249));
#23111=CARTESIAN_POINT('Ctrl Pts',(-0.175644148889271,-1.,1.88188663144846));
#23112=CARTESIAN_POINT('Ctrl Pts',(-0.175644148889271,1.,1.88188663144846));
#23113=CARTESIAN_POINT('Ctrl Pts',(-0.175538155840286,-1.,1.88742606272818));
#23114=CARTESIAN_POINT('Ctrl Pts',(-0.175538155840286,1.,1.88742606272818));
#23115=CARTESIAN_POINT('Ctrl Pts',(-0.175274276190664,-1.,1.89264630198279));
#23116=CARTESIAN_POINT('Ctrl Pts',(-0.175274276190664,1.,1.89264630198279));
#23117=CARTESIAN_POINT('Ctrl Pts',(-0.174879405091277,-1.,1.89788101117148));
#23118=CARTESIAN_POINT('Ctrl Pts',(-0.174879405091277,1.,1.89788101117148));
#23119=CARTESIAN_POINT('Ctrl Pts',(-0.174375518661222,-1.,1.90335253863003));
#23120=CARTESIAN_POINT('Ctrl Pts',(-0.174375518661222,1.,1.90335253863003));
#23121=CARTESIAN_POINT('Ctrl Pts',(-0.173776635257984,-1.,1.90911693975475));
#23122=CARTESIAN_POINT('Ctrl Pts',(-0.173776635257984,1.,1.90911693975475));
#23123=CARTESIAN_POINT('Ctrl Pts',(-0.173090695383619,-1.,1.91511429159681));
#23124=CARTESIAN_POINT('Ctrl Pts',(-0.173090695383619,1.,1.91511429159681));
#23125=CARTESIAN_POINT('Ctrl Pts',(-0.172321621259557,-1.,1.92122334398034));
#23126=CARTESIAN_POINT('Ctrl Pts',(-0.172321621259557,1.,1.92122334398034));
#23127=CARTESIAN_POINT('Ctrl Pts',(-0.17147119153296,-1.,1.92731093582));
#23128=CARTESIAN_POINT('Ctrl Pts',(-0.17147119153296,1.,1.92731093582));
#23129=CARTESIAN_POINT('Ctrl Pts',(-0.170541253116136,-1.,1.93329183155455));
#23130=CARTESIAN_POINT('Ctrl Pts',(-0.170541253116136,1.,1.93329183155455));
#23131=CARTESIAN_POINT('Ctrl Pts',(-0.169534904817425,-1.,1.93915639211497));
#23132=CARTESIAN_POINT('Ctrl Pts',(-0.169534904817425,1.,1.93915639211497));
#23133=CARTESIAN_POINT('Ctrl Pts',(-0.168455741607516,-1.,1.94493757756879));
#23134=CARTESIAN_POINT('Ctrl Pts',(-0.168455741607516,1.,1.94493757756879));
#23135=CARTESIAN_POINT('Ctrl Pts',(-0.167307501784469,-1.,1.95069027794286));
#23136=CARTESIAN_POINT('Ctrl Pts',(-0.167307501784469,1.,1.95069027794286));
#23137=CARTESIAN_POINT('Ctrl Pts',(-0.166093592002833,-1.,1.95646759718755));
#23138=CARTESIAN_POINT('Ctrl Pts',(-0.166093592002833,1.,1.95646759718755));
#23139=CARTESIAN_POINT('Ctrl Pts',(-0.1648165689203,-1.,1.96229379940174));
#23140=CARTESIAN_POINT('Ctrl Pts',(-0.1648165689203,1.,1.96229379940174));
#23141=CARTESIAN_POINT('Ctrl Pts',(-0.16347818545776,-1.,1.96816512678));
#23142=CARTESIAN_POINT('Ctrl Pts',(-0.16347818545776,1.,1.96816512678));
#23143=CARTESIAN_POINT('Ctrl Pts',(-0.162079693556302,-1.,1.97406280235204));
#23144=CARTESIAN_POINT('Ctrl Pts',(-0.162079693556302,1.,1.97406280235204));
#23145=CARTESIAN_POINT('Ctrl Pts',(-0.16062206078461,-1.,1.97996195437557));
#23146=CARTESIAN_POINT('Ctrl Pts',(-0.16062206078461,1.,1.97996195437557));
#23147=CARTESIAN_POINT('Ctrl Pts',(-0.159106226437289,-1.,1.98584238283279));
#23148=CARTESIAN_POINT('Ctrl Pts',(-0.159106226437289,1.,1.98584238283279));
#23149=CARTESIAN_POINT('Ctrl Pts',(-0.157533331459215,-1.,1.99169810931893));
#23150=CARTESIAN_POINT('Ctrl Pts',(-0.157533331459215,1.,1.99169810931893));
#23151=CARTESIAN_POINT('Ctrl Pts',(-0.155904629548775,-1.,1.99753284771487));
#23152=CARTESIAN_POINT('Ctrl Pts',(-0.155904629548775,1.,1.99753284771487));
#23153=CARTESIAN_POINT('Ctrl Pts',(-0.154221403049719,-1.,2.00335565310539));
#23154=CARTESIAN_POINT('Ctrl Pts',(-0.154221403049719,1.,2.00335565310539));
#23155=CARTESIAN_POINT('Ctrl Pts',(-0.152484883621452,-1.,2.00917680318426));
#23156=CARTESIAN_POINT('Ctrl Pts',(-0.152484883621452,1.,2.00917680318426));
#23157=CARTESIAN_POINT('Ctrl Pts',(-0.150696157673084,-1.,2.01500291940243));
#23158=CARTESIAN_POINT('Ctrl Pts',(-0.150696157673084,1.,2.01500291940243));
#23159=CARTESIAN_POINT('Ctrl Pts',(-0.148856124775343,-1.,2.02083464969897));
#23160=CARTESIAN_POINT('Ctrl Pts',(-0.148856124775343,1.,2.02083464969897));
#23161=CARTESIAN_POINT('Ctrl Pts',(-0.146965557332586,-1.,2.02666926182017));
#23162=CARTESIAN_POINT('Ctrl Pts',(-0.146965557332586,1.,2.02666926182017));
#23163=CARTESIAN_POINT('Ctrl Pts',(-0.145025140186058,-1.,2.03250223739941));
#23164=CARTESIAN_POINT('Ctrl Pts',(-0.145025140186058,1.,2.03250223739941));
#23165=CARTESIAN_POINT('Ctrl Pts',(-0.143035515058208,-1.,2.03832911025913));
#23166=CARTESIAN_POINT('Ctrl Pts',(-0.143035515058208,1.,2.03832911025913));
#23167=CARTESIAN_POINT('Ctrl Pts',(-0.140997332152546,-1.,2.04414757947919));
#23168=CARTESIAN_POINT('Ctrl Pts',(-0.140997332152546,1.,2.04414757947919));
#23169=CARTESIAN_POINT('Ctrl Pts',(-0.138911255368966,-1.,2.04995762001333));
#23170=CARTESIAN_POINT('Ctrl Pts',(-0.138911255368966,1.,2.04995762001333));
#23171=CARTESIAN_POINT('Ctrl Pts',(-0.136777941218044,-1.,2.0557604441427));
#23172=CARTESIAN_POINT('Ctrl Pts',(-0.136777941218044,1.,2.0557604441427));
#23173=CARTESIAN_POINT('Ctrl Pts',(-0.134598026192107,-1.,2.06155781517844));
#23174=CARTESIAN_POINT('Ctrl Pts',(-0.134598026192107,1.,2.06155781517844));
#23175=CARTESIAN_POINT('Ctrl Pts',(-0.13237211154771,-1.,2.06735123910319));
#23176=CARTESIAN_POINT('Ctrl Pts',(-0.13237211154771,1.,2.06735123910319));
#23177=CARTESIAN_POINT('Ctrl Pts',(-0.130100748328401,-1.,2.07314114713047));
#23178=CARTESIAN_POINT('Ctrl Pts',(-0.130100748328401,1.,2.07314114713047));
#23179=CARTESIAN_POINT('Ctrl Pts',(-0.127784445276116,-1.,2.07892715110967));
#23180=CARTESIAN_POINT('Ctrl Pts',(-0.127784445276116,1.,2.07892715110967));
#23181=CARTESIAN_POINT('Ctrl Pts',(-0.125423679412058,-1.,2.08470840653628));
#23182=CARTESIAN_POINT('Ctrl Pts',(-0.125423679412058,1.,2.08470840653628));
#23183=CARTESIAN_POINT('Ctrl Pts',(-0.123018905621083,-1.,2.09048392424826));
#23184=CARTESIAN_POINT('Ctrl Pts',(-0.123018905621083,1.,2.09048392424826));
#23185=CARTESIAN_POINT('Ctrl Pts',(-0.120570567965129,-1.,2.09625292867756));
#23186=CARTESIAN_POINT('Ctrl Pts',(-0.120570567965129,1.,2.09625292867756));
#23187=CARTESIAN_POINT('Ctrl Pts',(-0.118079107988368,-1.,2.10201512132945));
#23188=CARTESIAN_POINT('Ctrl Pts',(-0.118079107988368,1.,2.10201512132945));
#23189=CARTESIAN_POINT('Ctrl Pts',(-0.115544957687941,-1.,2.10777050261359));
#23190=CARTESIAN_POINT('Ctrl Pts',(-0.115544957687941,1.,2.10777050261359));
#23191=CARTESIAN_POINT('Ctrl Pts',(-0.112968534419746,-1.,2.11351924490335));
#23192=CARTESIAN_POINT('Ctrl Pts',(-0.112968534419746,1.,2.11351924490335));
#23193=CARTESIAN_POINT('Ctrl Pts',(-0.11035023613502,-1.,2.11926155590849));
#23194=CARTESIAN_POINT('Ctrl Pts',(-0.11035023613502,1.,2.11926155590849));
#23195=CARTESIAN_POINT('Ctrl Pts',(-0.107690435231068,-1.,2.12499752306927));
#23196=CARTESIAN_POINT('Ctrl Pts',(-0.107690435231068,1.,2.12499752306927));
#23197=CARTESIAN_POINT('Ctrl Pts',(-0.104989479152703,-1.,2.1307270488718));
#23198=CARTESIAN_POINT('Ctrl Pts',(-0.104989479152703,1.,2.1307270488718));
#23199=CARTESIAN_POINT('Ctrl Pts',(-0.102247700556064,-1.,2.13644992667052));
#23200=CARTESIAN_POINT('Ctrl Pts',(-0.102247700556064,1.,2.13644992667052));
#23201=CARTESIAN_POINT('Ctrl Pts',(-0.0994654261990745,-1.,2.14216588395974));
#23202=CARTESIAN_POINT('Ctrl Pts',(-0.0994654261990745,1.,2.14216588395974));
#23203=CARTESIAN_POINT('Ctrl Pts',(-0.0966429852305691,-1.,2.14787463531864));
#23204=CARTESIAN_POINT('Ctrl Pts',(-0.0966429852305691,1.,2.14787463531864));
#23205=CARTESIAN_POINT('Ctrl Pts',(-0.0937807218868348,-1.,2.15357593978377));
#23206=CARTESIAN_POINT('Ctrl Pts',(-0.0937807218868348,1.,2.15357593978377));
#23207=CARTESIAN_POINT('Ctrl Pts',(-0.0908789888108269,-1.,2.15926961544808));
#23208=CARTESIAN_POINT('Ctrl Pts',(-0.0908789888108269,1.,2.15926961544808));
#23209=CARTESIAN_POINT('Ctrl Pts',(-0.0879381291387825,-1.,2.16495552645275));
#23210=CARTESIAN_POINT('Ctrl Pts',(-0.0879381291387825,1.,2.16495552645275));
#23211=CARTESIAN_POINT('Ctrl Pts',(-0.0849584620835646,-1.,2.17063357871031));
#23212=CARTESIAN_POINT('Ctrl Pts',(-0.0849584620835646,1.,2.17063357871031));
#23213=CARTESIAN_POINT('Ctrl Pts',(-0.0819402680871942,-1.,2.1763037121106));
#23214=CARTESIAN_POINT('Ctrl Pts',(-0.0819402680871942,1.,2.1763037121106));
#23215=CARTESIAN_POINT('Ctrl Pts',(-0.078883772768323,-1.,2.18196589448304));
#23216=CARTESIAN_POINT('Ctrl Pts',(-0.078883772768323,1.,2.18196589448304));
#23217=CARTESIAN_POINT('Ctrl Pts',(-0.0757891465833414,-1.,2.1876201139874));
#23218=CARTESIAN_POINT('Ctrl Pts',(-0.0757891465833414,1.,2.1876201139874));
#23219=CARTESIAN_POINT('Ctrl Pts',(-0.0732830357304279,-1.,2.19213712012956));
#23220=CARTESIAN_POINT('Ctrl Pts',(-0.0732830357304279,1.,2.19213712012956));
#23221=CARTESIAN_POINT('Ctrl Pts',(-0.071386377952463,-1.,2.19552129483562));
#23222=CARTESIAN_POINT('Ctrl Pts',(-0.071386377952463,1.,2.19552129483562));
#23223=CARTESIAN_POINT('Ctrl Pts',(-0.0701143536324929,-1.,2.19777582085261));
#23224=CARTESIAN_POINT('Ctrl Pts',(-0.0701143536324929,1.,2.19777582085261));
#23225=CARTESIAN_POINT('Ctrl Pts',(-0.0694764450219586,-1.,2.19890268624765));
#23226=CARTESIAN_POINT('Ctrl Pts',(-0.0694764450219586,1.,2.19890268624765));
#23227=CARTESIAN_POINT('',(-0.163289472382896,1.,1.74236521665491));
#23228=CARTESIAN_POINT('Ctrl Pts',(-0.163289472382896,1.,1.74236521665491));
#23229=CARTESIAN_POINT('Ctrl Pts',(-0.163814161002474,1.,1.74720349503904));
#23230=CARTESIAN_POINT('Ctrl Pts',(-0.164834765708484,1.,1.75666056640041));
#23231=CARTESIAN_POINT('Ctrl Pts',(-0.166279355148738,1.,1.77018771687692));
#23232=CARTESIAN_POINT('Ctrl Pts',(-0.16803277280837,1.,1.78690649988931));
#23233=CARTESIAN_POINT('Ctrl Pts',(-0.169936923908078,1.,1.80561530633924));
#23234=CARTESIAN_POINT('Ctrl Pts',(-0.171554770207306,1.,1.82215766815414));
#23235=CARTESIAN_POINT('Ctrl Pts',(-0.17288944289442,1.,1.83658380530747));
#23236=CARTESIAN_POINT('Ctrl Pts',(-0.173946627589401,1.,1.84898113200543));
#23237=CARTESIAN_POINT('Ctrl Pts',(-0.174735259276856,1.,1.85948367089838));
#23238=CARTESIAN_POINT('Ctrl Pts',(-0.175268337590901,1.,1.86828349694972));
#23239=CARTESIAN_POINT('Ctrl Pts',(-0.175563480746206,1.,1.87563767773249));
#23240=CARTESIAN_POINT('Ctrl Pts',(-0.175644148889271,1.,1.88188663144846));
#23241=CARTESIAN_POINT('Ctrl Pts',(-0.175538155840286,1.,1.88742606272818));
#23242=CARTESIAN_POINT('Ctrl Pts',(-0.175274276190664,1.,1.89264630198279));
#23243=CARTESIAN_POINT('Ctrl Pts',(-0.174879405091277,1.,1.89788101117148));
#23244=CARTESIAN_POINT('Ctrl Pts',(-0.174375518661222,1.,1.90335253863003));
#23245=CARTESIAN_POINT('Ctrl Pts',(-0.173776635257984,1.,1.90911693975475));
#23246=CARTESIAN_POINT('Ctrl Pts',(-0.173090695383619,1.,1.91511429159681));
#23247=CARTESIAN_POINT('Ctrl Pts',(-0.172321621259557,1.,1.92122334398034));
#23248=CARTESIAN_POINT('Ctrl Pts',(-0.17147119153296,1.,1.92731093582));
#23249=CARTESIAN_POINT('Ctrl Pts',(-0.170541253116136,1.,1.93329183155455));
#23250=CARTESIAN_POINT('Ctrl Pts',(-0.169534904817425,1.,1.93915639211497));
#23251=CARTESIAN_POINT('Ctrl Pts',(-0.168455741607516,1.,1.94493757756879));
#23252=CARTESIAN_POINT('Ctrl Pts',(-0.167307501784469,1.,1.95069027794286));
#23253=CARTESIAN_POINT('Ctrl Pts',(-0.166093592002833,1.,1.95646759718755));
#23254=CARTESIAN_POINT('Ctrl Pts',(-0.1648165689203,1.,1.96229379940174));
#23255=CARTESIAN_POINT('Ctrl Pts',(-0.16347818545776,1.,1.96816512678));
#23256=CARTESIAN_POINT('Ctrl Pts',(-0.162079693556302,1.,1.97406280235204));
#23257=CARTESIAN_POINT('Ctrl Pts',(-0.16062206078461,1.,1.97996195437557));
#23258=CARTESIAN_POINT('Ctrl Pts',(-0.159106226437289,1.,1.98584238283279));
#23259=CARTESIAN_POINT('Ctrl Pts',(-0.157533331459215,1.,1.99169810931893));
#23260=CARTESIAN_POINT('Ctrl Pts',(-0.155904629548775,1.,1.99753284771487));
#23261=CARTESIAN_POINT('Ctrl Pts',(-0.154221403049719,1.,2.00335565310539));
#23262=CARTESIAN_POINT('Ctrl Pts',(-0.152484883621452,1.,2.00917680318426));
#23263=CARTESIAN_POINT('Ctrl Pts',(-0.150696157673084,1.,2.01500291940243));
#23264=CARTESIAN_POINT('Ctrl Pts',(-0.148856124775343,1.,2.02083464969897));
#23265=CARTESIAN_POINT('Ctrl Pts',(-0.146965557332586,1.,2.02666926182017));
#23266=CARTESIAN_POINT('Ctrl Pts',(-0.145025140186058,1.,2.03250223739941));
#23267=CARTESIAN_POINT('Ctrl Pts',(-0.143035515058208,1.,2.03832911025913));
#23268=CARTESIAN_POINT('Ctrl Pts',(-0.140997332152546,1.,2.04414757947919));
#23269=CARTESIAN_POINT('Ctrl Pts',(-0.138911255368966,1.,2.04995762001333));
#23270=CARTESIAN_POINT('Ctrl Pts',(-0.136777941218044,1.,2.0557604441427));
#23271=CARTESIAN_POINT('Ctrl Pts',(-0.134598026192107,1.,2.06155781517844));
#23272=CARTESIAN_POINT('Ctrl Pts',(-0.13237211154771,1.,2.06735123910319));
#23273=CARTESIAN_POINT('Ctrl Pts',(-0.130100748328401,1.,2.07314114713047));
#23274=CARTESIAN_POINT('Ctrl Pts',(-0.127784445276116,1.,2.07892715110967));
#23275=CARTESIAN_POINT('Ctrl Pts',(-0.125423679412058,1.,2.08470840653628));
#23276=CARTESIAN_POINT('Ctrl Pts',(-0.123018905621083,1.,2.09048392424826));
#23277=CARTESIAN_POINT('Ctrl Pts',(-0.120570567965129,1.,2.09625292867756));
#23278=CARTESIAN_POINT('Ctrl Pts',(-0.118079107988368,1.,2.10201512132945));
#23279=CARTESIAN_POINT('Ctrl Pts',(-0.115544957687941,1.,2.10777050261359));
#23280=CARTESIAN_POINT('Ctrl Pts',(-0.112968534419746,1.,2.11351924490335));
#23281=CARTESIAN_POINT('Ctrl Pts',(-0.11035023613502,1.,2.11926155590849));
#23282=CARTESIAN_POINT('Ctrl Pts',(-0.107690435231068,1.,2.12499752306927));
#23283=CARTESIAN_POINT('Ctrl Pts',(-0.104989479152703,1.,2.1307270488718));
#23284=CARTESIAN_POINT('Ctrl Pts',(-0.102247700556064,1.,2.13644992667052));
#23285=CARTESIAN_POINT('Ctrl Pts',(-0.0994654261990745,1.,2.14216588395974));
#23286=CARTESIAN_POINT('Ctrl Pts',(-0.0966429852305691,1.,2.14787463531864));
#23287=CARTESIAN_POINT('Ctrl Pts',(-0.0937807218868348,1.,2.15357593978377));
#23288=CARTESIAN_POINT('Ctrl Pts',(-0.0908789888108269,1.,2.15926961544808));
#23289=CARTESIAN_POINT('Ctrl Pts',(-0.0879381291387825,1.,2.16495552645275));
#23290=CARTESIAN_POINT('Ctrl Pts',(-0.0849584620835646,1.,2.17063357871031));
#23291=CARTESIAN_POINT('Ctrl Pts',(-0.0819402680871942,1.,2.1763037121106));
#23292=CARTESIAN_POINT('Ctrl Pts',(-0.078883772768323,1.,2.18196589448304));
#23293=CARTESIAN_POINT('Ctrl Pts',(-0.0757891465833414,1.,2.1876201139874));
#23294=CARTESIAN_POINT('Ctrl Pts',(-0.0732830357304279,1.,2.19213712012956));
#23295=CARTESIAN_POINT('Ctrl Pts',(-0.071386377952463,1.,2.19552129483562));
#23296=CARTESIAN_POINT('Ctrl Pts',(-0.0701143536324929,1.,2.19777582085261));
#23297=CARTESIAN_POINT('Ctrl Pts',(-0.0694764450219586,1.,2.19890268624765));
#23298=CARTESIAN_POINT('',(-0.163289472382897,0.,1.74236521665491));
#23299=CARTESIAN_POINT('Origin',(0.,0.,0.));
#23300=CARTESIAN_POINT('',(-0.383122945602004,1.,1.7075470150345));
#23301=CARTESIAN_POINT('Origin',(0.,1.,0.));
#23302=CARTESIAN_POINT('',(-0.383122945602004,0.,1.7075470150345));
#23303=CARTESIAN_POINT('Ctrl Pts',(-0.61342227326009,-1.,2.11275013067528));
#23304=CARTESIAN_POINT('Ctrl Pts',(-0.61342227326009,1.,2.11275013067528));
#23305=CARTESIAN_POINT('Ctrl Pts',(-0.61246736556225,-1.,2.11187554260142));
#23306=CARTESIAN_POINT('Ctrl Pts',(-0.61246736556225,1.,2.11187554260142));
#23307=CARTESIAN_POINT('Ctrl Pts',(-0.610560911691113,-1.,2.11012443807661));
#23308=CARTESIAN_POINT('Ctrl Pts',(-0.610560911691113,1.,2.11012443807661));
#23309=CARTESIAN_POINT('Ctrl Pts',(-0.607711315456826,-1.,2.10749199615859));
#23310=CARTESIAN_POINT('Ctrl Pts',(-0.607711315456826,1.,2.10749199615859));
#23311=CARTESIAN_POINT('Ctrl Pts',(-0.603932030738212,-1.,2.10397049887709));
#23312=CARTESIAN_POINT('Ctrl Pts',(-0.603932030738212,1.,2.10397049887709));
#23313=CARTESIAN_POINT('Ctrl Pts',(-0.599241616422144,-1.,2.09954930865331));
#23314=CARTESIAN_POINT('Ctrl Pts',(-0.599241616422144,1.,2.09954930865331));
#23315=CARTESIAN_POINT('Ctrl Pts',(-0.594585006052824,-1.,2.09510876220501));
#23316=CARTESIAN_POINT('Ctrl Pts',(-0.594585006052824,1.,2.09510876220501));
#23317=CARTESIAN_POINT('Ctrl Pts',(-0.589962365403189,-1.,2.09064881812053));
#23318=CARTESIAN_POINT('Ctrl Pts',(-0.589962365403189,1.,2.09064881812053));
#23319=CARTESIAN_POINT('Ctrl Pts',(-0.585373918990895,-1.,2.086169437277));
#23320=CARTESIAN_POINT('Ctrl Pts',(-0.585373918990895,1.,2.086169437277));
#23321=CARTESIAN_POINT('Ctrl Pts',(-0.580819952107257,-1.,2.08167059018138));
#23322=CARTESIAN_POINT('Ctrl Pts',(-0.580819952107257,1.,2.08167059018138));
#23323=CARTESIAN_POINT('Ctrl Pts',(-0.576300797416275,-1.,2.07715226767361));
#23324=CARTESIAN_POINT('Ctrl Pts',(-0.576300797416275,1.,2.07715226767361));
#23325=CARTESIAN_POINT('Ctrl Pts',(-0.571816823242411,-1.,2.07261449292757));
#23326=CARTESIAN_POINT('Ctrl Pts',(-0.571816823242411,1.,2.07261449292757));
#23327=CARTESIAN_POINT('Ctrl Pts',(-0.567368421181229,-1.,2.06805732997383));
#23328=CARTESIAN_POINT('Ctrl Pts',(-0.567368421181229,1.,2.06805732997383));
#23329=CARTESIAN_POINT('Ctrl Pts',(-0.562955993082574,-1.,2.06348090160697));
#23330=CARTESIAN_POINT('Ctrl Pts',(-0.562955993082574,1.,2.06348090160697));
#23331=CARTESIAN_POINT('Ctrl Pts',(-0.558579940185467,-1.,2.05888537756571));
#23332=CARTESIAN_POINT('Ctrl Pts',(-0.558579940185467,1.,2.05888537756571));
#23333=CARTESIAN_POINT('Ctrl Pts',(-0.55424065746411,-1.,2.05427091604482));
#23334=CARTESIAN_POINT('Ctrl Pts',(-0.55424065746411,1.,2.05427091604482));
#23335=CARTESIAN_POINT('Ctrl Pts',(-0.549938525150342,-1.,2.04963761077974));
#23336=CARTESIAN_POINT('Ctrl Pts',(-0.549938525150342,1.,2.04963761077974));
#23337=CARTESIAN_POINT('Ctrl Pts',(-0.545673903817348,-1.,2.0449854471456));
#23338=CARTESIAN_POINT('Ctrl Pts',(-0.545673903817348,1.,2.0449854471456));
#23339=CARTESIAN_POINT('Ctrl Pts',(-0.54144712061552,-1.,2.0403142269048));
#23340=CARTESIAN_POINT('Ctrl Pts',(-0.54144712061552,1.,2.0403142269048));
#23341=CARTESIAN_POINT('Ctrl Pts',(-0.537258489833134,-1.,2.03562362953993));
#23342=CARTESIAN_POINT('Ctrl Pts',(-0.537258489833134,1.,2.03562362953993));
#23343=CARTESIAN_POINT('Ctrl Pts',(-0.533108355132905,-1.,2.03091336214401));
#23344=CARTESIAN_POINT('Ctrl Pts',(-0.533108355132905,1.,2.03091336214401));
#23345=CARTESIAN_POINT('Ctrl Pts',(-0.528997127241911,-1.,2.02618329083289));
#23346=CARTESIAN_POINT('Ctrl Pts',(-0.528997127241911,1.,2.02618329083289));
#23347=CARTESIAN_POINT('Ctrl Pts',(-0.524925318333518,-1.,2.02143356304712));
#23348=CARTESIAN_POINT('Ctrl Pts',(-0.524925318333518,1.,2.02143356304712));
#23349=CARTESIAN_POINT('Ctrl Pts',(-0.520893590399428,-1.,2.01666477917305));
#23350=CARTESIAN_POINT('Ctrl Pts',(-0.520893590399428,1.,2.01666477917305));
#23351=CARTESIAN_POINT('Ctrl Pts',(-0.516902681728733,-1.,2.01187773939257));
#23352=CARTESIAN_POINT('Ctrl Pts',(-0.516902681728733,1.,2.01187773939257));
#23353=CARTESIAN_POINT('Ctrl Pts',(-0.512953306961814,-1.,2.00707309946955));
#23354=CARTESIAN_POINT('Ctrl Pts',(-0.512953306961814,1.,2.00707309946955));
#23355=CARTESIAN_POINT('Ctrl Pts',(-0.509046069886152,-1.,2.00225107134733));
#23356=CARTESIAN_POINT('Ctrl Pts',(-0.509046069886152,1.,2.00225107134733));
#23357=CARTESIAN_POINT('Ctrl Pts',(-0.505181361323011,-1.,1.99741107463567));
#23358=CARTESIAN_POINT('Ctrl Pts',(-0.505181361323011,1.,1.99741107463567));
#23359=CARTESIAN_POINT('Ctrl Pts',(-0.501359287727129,-1.,1.9925514912615));
#23360=CARTESIAN_POINT('Ctrl Pts',(-0.501359287727129,1.,1.9925514912615));
#23361=CARTESIAN_POINT('Ctrl Pts',(-0.497579909545564,-1.,1.98767044752929));
#23362=CARTESIAN_POINT('Ctrl Pts',(-0.497579909545564,1.,1.98767044752929));
#23363=CARTESIAN_POINT('Ctrl Pts',(-0.493843476541492,-1.,1.9827665876182));
#23364=CARTESIAN_POINT('Ctrl Pts',(-0.493843476541492,1.,1.9827665876182));
#23365=CARTESIAN_POINT('Ctrl Pts',(-0.490150627860955,-1.,1.97783973019229));
#23366=CARTESIAN_POINT('Ctrl Pts',(-0.490150627860955,1.,1.97783973019229));
#23367=CARTESIAN_POINT('Ctrl Pts',(-0.486502692907661,-1.,1.97289186263272));
#23368=CARTESIAN_POINT('Ctrl Pts',(-0.486502692907661,1.,1.97289186263272));
#23369=CARTESIAN_POINT('Ctrl Pts',(-0.482901662120687,-1.,1.96792703422358));
#23370=CARTESIAN_POINT('Ctrl Pts',(-0.482901662120687,1.,1.96792703422358));
#23371=CARTESIAN_POINT('Ctrl Pts',(-0.479349583074846,-1.,1.96294933055938));
#23372=CARTESIAN_POINT('Ctrl Pts',(-0.479349583074846,1.,1.96294933055938));
#23373=CARTESIAN_POINT('Ctrl Pts',(-0.475848034683172,-1.,1.95796111148175));
#23374=CARTESIAN_POINT('Ctrl Pts',(-0.475848034683172,1.,1.95796111148175));
#23375=CARTESIAN_POINT('Ctrl Pts',(-0.47239767226408,-1.,1.95296148278136));
#23376=CARTESIAN_POINT('Ctrl Pts',(-0.47239767226408,1.,1.95296148278136));
#23377=CARTESIAN_POINT('Ctrl Pts',(-0.468997482913158,-1.,1.94794381136524));
#23378=CARTESIAN_POINT('Ctrl Pts',(-0.468997482913158,1.,1.94794381136524));
#23379=CARTESIAN_POINT('Ctrl Pts',(-0.465645462026065,-1.,1.94289794196205));
#23380=CARTESIAN_POINT('Ctrl Pts',(-0.465645462026065,1.,1.94289794196205));
#23381=CARTESIAN_POINT('Ctrl Pts',(-0.462340031009087,-1.,1.93781486640834));
#23382=CARTESIAN_POINT('Ctrl Pts',(-0.462340031009087,1.,1.93781486640834));
#23383=CARTESIAN_POINT('Ctrl Pts',(-0.459081234547931,-1.,1.93269066517936));
#23384=CARTESIAN_POINT('Ctrl Pts',(-0.459081234547931,1.,1.93269066517936));
#23385=CARTESIAN_POINT('Ctrl Pts',(-0.455872005174335,-1.,1.92753067150461));
#23386=CARTESIAN_POINT('Ctrl Pts',(-0.455872005174335,1.,1.92753067150461));
#23387=CARTESIAN_POINT('Ctrl Pts',(-0.452719478359356,-1.,1.9223538064847));
#23388=CARTESIAN_POINT('Ctrl Pts',(-0.452719478359356,1.,1.9223538064847));
#23389=CARTESIAN_POINT('Ctrl Pts',(-0.449632260106572,-1.,1.91718342555717));
#23390=CARTESIAN_POINT('Ctrl Pts',(-0.449632260106572,1.,1.91718342555717));
#23391=CARTESIAN_POINT('Ctrl Pts',(-0.446617343485651,-1.,1.91203699981095));
#23392=CARTESIAN_POINT('Ctrl Pts',(-0.446617343485651,1.,1.91203699981095));
#23393=CARTESIAN_POINT('Ctrl Pts',(-0.44367755684917,-1.,1.90691756144906));
#23394=CARTESIAN_POINT('Ctrl Pts',(-0.44367755684917,1.,1.90691756144906));
#23395=CARTESIAN_POINT('Ctrl Pts',(-0.440807833704161,-1.,1.90180124389137));
#23396=CARTESIAN_POINT('Ctrl Pts',(-0.440807833704161,1.,1.90180124389137));
#23397=CARTESIAN_POINT('Ctrl Pts',(-0.437995003948443,-1.,1.89663648956549));
#23398=CARTESIAN_POINT('Ctrl Pts',(-0.437995003948443,1.,1.89663648956549));
#23399=CARTESIAN_POINT('Ctrl Pts',(-0.43522566096358,-1.,1.89136993975585));
#23400=CARTESIAN_POINT('Ctrl Pts',(-0.43522566096358,1.,1.89136993975585));
#23401=CARTESIAN_POINT('Ctrl Pts',(-0.432493038548833,-1.,1.88596913666828));
#23402=CARTESIAN_POINT('Ctrl Pts',(-0.432493038548833,1.,1.88596913666828));
#23403=CARTESIAN_POINT('Ctrl Pts',(-0.429803062482217,-1.,1.88044229001778));
#23404=CARTESIAN_POINT('Ctrl Pts',(-0.429803062482217,1.,1.88044229001778));
#23405=CARTESIAN_POINT('Ctrl Pts',(-0.427183828518743,-1.,1.87486989291333));
#23406=CARTESIAN_POINT('Ctrl Pts',(-0.427183828518743,1.,1.87486989291333));
#23407=CARTESIAN_POINT('Ctrl Pts',(-0.424678177290876,-1.,1.8693780394412));
#23408=CARTESIAN_POINT('Ctrl Pts',(-0.424678177290876,1.,1.8693780394412));
#23409=CARTESIAN_POINT('Ctrl Pts',(-0.422327307417885,-1.,1.86408083333863));
#23410=CARTESIAN_POINT('Ctrl Pts',(-0.422327307417885,1.,1.86408083333863));
#23411=CARTESIAN_POINT('Ctrl Pts',(-0.420157287975583,-1.,1.8590328109667));
#23412=CARTESIAN_POINT('Ctrl Pts',(-0.420157287975583,1.,1.8590328109667));
#23413=CARTESIAN_POINT('Ctrl Pts',(-0.418164129144045,-1.,1.8541763285645));
#23414=CARTESIAN_POINT('Ctrl Pts',(-0.418164129144045,1.,1.8541763285645));
#23415=CARTESIAN_POINT('Ctrl Pts',(-0.416300022039885,-1.,1.84929312930314));
#23416=CARTESIAN_POINT('Ctrl Pts',(-0.416300022039885,1.,1.84929312930314));
#23417=CARTESIAN_POINT('Ctrl Pts',(-0.414487438255542,-1.,1.84405757074218));
#23418=CARTESIAN_POINT('Ctrl Pts',(-0.414487438255542,1.,1.84405757074218));
#23419=CARTESIAN_POINT('Ctrl Pts',(-0.412633125322945,-1.,1.8380895347617));
#23420=CARTESIAN_POINT('Ctrl Pts',(-0.412633125322945,1.,1.8380895347617));
#23421=CARTESIAN_POINT('Ctrl Pts',(-0.410641256301276,-1.,1.83100408895047));
#23422=CARTESIAN_POINT('Ctrl Pts',(-0.410641256301276,1.,1.83100408895047));
#23423=CARTESIAN_POINT('Ctrl Pts',(-0.408428948106227,-1.,1.82247022677562));
#23424=CARTESIAN_POINT('Ctrl Pts',(-0.408428948106227,1.,1.82247022677562));
#23425=CARTESIAN_POINT('Ctrl Pts',(-0.405933518407175,-1.,1.81223801812013));
#23426=CARTESIAN_POINT('Ctrl Pts',(-0.405933518407175,1.,1.81223801812013));
#23427=CARTESIAN_POINT('Ctrl Pts',(-0.403107976163396,-1.,1.80012077173238));
#23428=CARTESIAN_POINT('Ctrl Pts',(-0.403107976163396,1.,1.80012077173238));
#23429=CARTESIAN_POINT('Ctrl Pts',(-0.399919403774155,-1.,1.78598826343754));
#23430=CARTESIAN_POINT('Ctrl Pts',(-0.399919403774155,1.,1.78598826343754));
#23431=CARTESIAN_POINT('Ctrl Pts',(-0.396346196110688,-1.,1.76975560043442));
#23432=CARTESIAN_POINT('Ctrl Pts',(-0.396346196110688,1.,1.76975560043442));
#23433=CARTESIAN_POINT('Ctrl Pts',(-0.392375812285395,-1.,1.75137405310193));
#23434=CARTESIAN_POINT('Ctrl Pts',(-0.392375812285395,1.,1.75137405310193));
#23435=CARTESIAN_POINT('Ctrl Pts',(-0.388877023502615,-1.,1.73493170972829));
#23436=CARTESIAN_POINT('Ctrl Pts',(-0.388877023502615,1.,1.73493170972829));
#23437=CARTESIAN_POINT('Ctrl Pts',(-0.386070790323281,-1.,1.72162022244582));
#23438=CARTESIAN_POINT('Ctrl Pts',(-0.386070790323281,1.,1.72162022244582));
#23439=CARTESIAN_POINT('Ctrl Pts',(-0.384119047314215,-1.,1.71231062891398));
#23440=CARTESIAN_POINT('Ctrl Pts',(-0.384119047314215,1.,1.71231062891398));
#23441=CARTESIAN_POINT('Ctrl Pts',(-0.383122945602004,-1.,1.7075470150345));
#23442=CARTESIAN_POINT('Ctrl Pts',(-0.383122945602004,1.,1.7075470150345));
#23443=CARTESIAN_POINT('',(-0.61342227326009,1.,2.11275013067528));
#23444=CARTESIAN_POINT('Ctrl Pts',(-0.61342227326009,1.,2.11275013067528));
#23445=CARTESIAN_POINT('Ctrl Pts',(-0.61246736556225,1.,2.11187554260142));
#23446=CARTESIAN_POINT('Ctrl Pts',(-0.610560911691113,1.,2.11012443807661));
#23447=CARTESIAN_POINT('Ctrl Pts',(-0.607711315456826,1.,2.10749199615859));
#23448=CARTESIAN_POINT('Ctrl Pts',(-0.603932030738212,1.,2.10397049887709));
#23449=CARTESIAN_POINT('Ctrl Pts',(-0.599241616422144,1.,2.09954930865331));
#23450=CARTESIAN_POINT('Ctrl Pts',(-0.594585006052824,1.,2.09510876220501));
#23451=CARTESIAN_POINT('Ctrl Pts',(-0.589962365403189,1.,2.09064881812053));
#23452=CARTESIAN_POINT('Ctrl Pts',(-0.585373918990895,1.,2.086169437277));
#23453=CARTESIAN_POINT('Ctrl Pts',(-0.580819952107257,1.,2.08167059018138));
#23454=CARTESIAN_POINT('Ctrl Pts',(-0.576300797416275,1.,2.07715226767361));
#23455=CARTESIAN_POINT('Ctrl Pts',(-0.571816823242411,1.,2.07261449292757));
#23456=CARTESIAN_POINT('Ctrl Pts',(-0.567368421181229,1.,2.06805732997383));
#23457=CARTESIAN_POINT('Ctrl Pts',(-0.562955993082574,1.,2.06348090160697));
#23458=CARTESIAN_POINT('Ctrl Pts',(-0.558579940185467,1.,2.05888537756571));
#23459=CARTESIAN_POINT('Ctrl Pts',(-0.55424065746411,1.,2.05427091604482));
#23460=CARTESIAN_POINT('Ctrl Pts',(-0.549938525150342,1.,2.04963761077974));
#23461=CARTESIAN_POINT('Ctrl Pts',(-0.545673903817348,1.,2.0449854471456));
#23462=CARTESIAN_POINT('Ctrl Pts',(-0.54144712061552,1.,2.0403142269048));
#23463=CARTESIAN_POINT('Ctrl Pts',(-0.537258489833134,1.,2.03562362953993));
#23464=CARTESIAN_POINT('Ctrl Pts',(-0.533108355132905,1.,2.03091336214401));
#23465=CARTESIAN_POINT('Ctrl Pts',(-0.528997127241911,1.,2.02618329083289));
#23466=CARTESIAN_POINT('Ctrl Pts',(-0.524925318333518,1.,2.02143356304712));
#23467=CARTESIAN_POINT('Ctrl Pts',(-0.520893590399428,1.,2.01666477917305));
#23468=CARTESIAN_POINT('Ctrl Pts',(-0.516902681728733,1.,2.01187773939257));
#23469=CARTESIAN_POINT('Ctrl Pts',(-0.512953306961814,1.,2.00707309946955));
#23470=CARTESIAN_POINT('Ctrl Pts',(-0.509046069886152,1.,2.00225107134733));
#23471=CARTESIAN_POINT('Ctrl Pts',(-0.505181361323011,1.,1.99741107463567));
#23472=CARTESIAN_POINT('Ctrl Pts',(-0.501359287727129,1.,1.9925514912615));
#23473=CARTESIAN_POINT('Ctrl Pts',(-0.497579909545564,1.,1.98767044752929));
#23474=CARTESIAN_POINT('Ctrl Pts',(-0.493843476541492,1.,1.9827665876182));
#23475=CARTESIAN_POINT('Ctrl Pts',(-0.490150627860955,1.,1.97783973019229));
#23476=CARTESIAN_POINT('Ctrl Pts',(-0.486502692907661,1.,1.97289186263272));
#23477=CARTESIAN_POINT('Ctrl Pts',(-0.482901662120687,1.,1.96792703422358));
#23478=CARTESIAN_POINT('Ctrl Pts',(-0.479349583074846,1.,1.96294933055938));
#23479=CARTESIAN_POINT('Ctrl Pts',(-0.475848034683172,1.,1.95796111148175));
#23480=CARTESIAN_POINT('Ctrl Pts',(-0.47239767226408,1.,1.95296148278136));
#23481=CARTESIAN_POINT('Ctrl Pts',(-0.468997482913158,1.,1.94794381136524));
#23482=CARTESIAN_POINT('Ctrl Pts',(-0.465645462026065,1.,1.94289794196205));
#23483=CARTESIAN_POINT('Ctrl Pts',(-0.462340031009087,1.,1.93781486640834));
#23484=CARTESIAN_POINT('Ctrl Pts',(-0.459081234547931,1.,1.93269066517936));
#23485=CARTESIAN_POINT('Ctrl Pts',(-0.455872005174335,1.,1.92753067150461));
#23486=CARTESIAN_POINT('Ctrl Pts',(-0.452719478359356,1.,1.9223538064847));
#23487=CARTESIAN_POINT('Ctrl Pts',(-0.449632260106572,1.,1.91718342555717));
#23488=CARTESIAN_POINT('Ctrl Pts',(-0.446617343485651,1.,1.91203699981095));
#23489=CARTESIAN_POINT('Ctrl Pts',(-0.44367755684917,1.,1.90691756144906));
#23490=CARTESIAN_POINT('Ctrl Pts',(-0.440807833704161,1.,1.90180124389137));
#23491=CARTESIAN_POINT('Ctrl Pts',(-0.437995003948443,1.,1.89663648956549));
#23492=CARTESIAN_POINT('Ctrl Pts',(-0.43522566096358,1.,1.89136993975585));
#23493=CARTESIAN_POINT('Ctrl Pts',(-0.432493038548833,1.,1.88596913666828));
#23494=CARTESIAN_POINT('Ctrl Pts',(-0.429803062482217,1.,1.88044229001778));
#23495=CARTESIAN_POINT('Ctrl Pts',(-0.427183828518743,1.,1.87486989291333));
#23496=CARTESIAN_POINT('Ctrl Pts',(-0.424678177290876,1.,1.8693780394412));
#23497=CARTESIAN_POINT('Ctrl Pts',(-0.422327307417885,1.,1.86408083333863));
#23498=CARTESIAN_POINT('Ctrl Pts',(-0.420157287975583,1.,1.8590328109667));
#23499=CARTESIAN_POINT('Ctrl Pts',(-0.418164129144045,1.,1.8541763285645));
#23500=CARTESIAN_POINT('Ctrl Pts',(-0.416300022039885,1.,1.84929312930314));
#23501=CARTESIAN_POINT('Ctrl Pts',(-0.414487438255542,1.,1.84405757074218));
#23502=CARTESIAN_POINT('Ctrl Pts',(-0.412633125322945,1.,1.8380895347617));
#23503=CARTESIAN_POINT('Ctrl Pts',(-0.410641256301276,1.,1.83100408895047));
#23504=CARTESIAN_POINT('Ctrl Pts',(-0.408428948106227,1.,1.82247022677562));
#23505=CARTESIAN_POINT('Ctrl Pts',(-0.405933518407175,1.,1.81223801812013));
#23506=CARTESIAN_POINT('Ctrl Pts',(-0.403107976163396,1.,1.80012077173238));
#23507=CARTESIAN_POINT('Ctrl Pts',(-0.399919403774155,1.,1.78598826343754));
#23508=CARTESIAN_POINT('Ctrl Pts',(-0.396346196110688,1.,1.76975560043442));
#23509=CARTESIAN_POINT('Ctrl Pts',(-0.392375812285395,1.,1.75137405310193));
#23510=CARTESIAN_POINT('Ctrl Pts',(-0.388877023502615,1.,1.73493170972829));
#23511=CARTESIAN_POINT('Ctrl Pts',(-0.386070790323281,1.,1.72162022244582));
#23512=CARTESIAN_POINT('Ctrl Pts',(-0.384119047314215,1.,1.71231062891398));
#23513=CARTESIAN_POINT('Ctrl Pts',(-0.383122945602004,1.,1.7075470150345));
#23514=CARTESIAN_POINT('',(-0.61342227326009,0.,2.11275013067528));
#23515=CARTESIAN_POINT('Origin',(-0.745574324794401,0.,2.0698113262342));
#23516=CARTESIAN_POINT('',(-0.745574324794401,1.,2.0698113262342));
#23517=CARTESIAN_POINT('',(-0.61342227326009,1.,2.11275013067528));
#23518=CARTESIAN_POINT('',(-0.745574324794401,0.,2.0698113262342));
#23519=CARTESIAN_POINT('Ctrl Pts',(-0.693717979106306,-1.,1.60662857109684));
#23520=CARTESIAN_POINT('Ctrl Pts',(-0.693717979106306,1.,1.60662857109684));
#23521=CARTESIAN_POINT('Ctrl Pts',(-0.695712097881194,-1.,1.61106790958151));
#23522=CARTESIAN_POINT('Ctrl Pts',(-0.695712097881194,1.,1.61106790958151));
#23523=CARTESIAN_POINT('Ctrl Pts',(-0.699605146405088,-1.,1.61974673472612));
#23524=CARTESIAN_POINT('Ctrl Pts',(-0.699605146405088,1.,1.61974673472612));
#23525=CARTESIAN_POINT('Ctrl Pts',(-0.705159151988319,-1.,1.63216541664676));
#23526=CARTESIAN_POINT('Ctrl Pts',(-0.705159151988319,1.,1.63216541664676));
#23527=CARTESIAN_POINT('Ctrl Pts',(-0.711993139355394,-1.,1.64752408832016));
#23528=CARTESIAN_POINT('Ctrl Pts',(-0.711993139355394,1.,1.64752408832016));
#23529=CARTESIAN_POINT('Ctrl Pts',(-0.719585433804282,-1.,1.6647288055568));
#23530=CARTESIAN_POINT('Ctrl Pts',(-0.719585433804282,1.,1.6647288055568));
#23531=CARTESIAN_POINT('Ctrl Pts',(-0.726235967997433,-1.,1.67996158455503));
#23532=CARTESIAN_POINT('Ctrl Pts',(-0.726235967997433,1.,1.67996158455503));
#23533=CARTESIAN_POINT('Ctrl Pts',(-0.731963238697195,-1.,1.69326921975743));
#23534=CARTESIAN_POINT('Ctrl Pts',(-0.731963238697195,1.,1.69326921975743));
#23535=CARTESIAN_POINT('Ctrl Pts',(-0.736799665724771,-1.,1.70473309006121));
#23536=CARTESIAN_POINT('Ctrl Pts',(-0.736799665724771,1.,1.70473309006121));
#23537=CARTESIAN_POINT('Ctrl Pts',(-0.740795162032088,-1.,1.71447789751927));
#23538=CARTESIAN_POINT('Ctrl Pts',(-0.740795162032088,1.,1.71447789751927));
#23539=CARTESIAN_POINT('Ctrl Pts',(-0.744021445433764,-1.,1.7226822991693));
#23540=CARTESIAN_POINT('Ctrl Pts',(-0.744021445433764,1.,1.7226822991693));
#23541=CARTESIAN_POINT('Ctrl Pts',(-0.746574710096436,-1.,1.72958533647399));
#23542=CARTESIAN_POINT('Ctrl Pts',(-0.746574710096436,1.,1.72958533647399));
#23543=CARTESIAN_POINT('Ctrl Pts',(-0.748582462954855,-1.,1.73550351679848));
#23544=CARTESIAN_POINT('Ctrl Pts',(-0.748582462954855,1.,1.73550351679848));
#23545=CARTESIAN_POINT('Ctrl Pts',(-0.75019343597954,-1.,1.74080458266705));
#23546=CARTESIAN_POINT('Ctrl Pts',(-0.75019343597954,1.,1.74080458266705));
#23547=CARTESIAN_POINT('Ctrl Pts',(-0.751555614163629,-1.,1.74585086852298));
#23548=CARTESIAN_POINT('Ctrl Pts',(-0.751555614163629,1.,1.74585086852298));
#23549=CARTESIAN_POINT('Ctrl Pts',(-0.752797683531377,-1.,1.75095139468809));
#23550=CARTESIAN_POINT('Ctrl Pts',(-0.752797683531377,1.,1.75095139468809));
#23551=CARTESIAN_POINT('Ctrl Pts',(-0.75400925402848,-1.,1.75631083600175));
#23552=CARTESIAN_POINT('Ctrl Pts',(-0.75400925402848,1.,1.75631083600175));
#23553=CARTESIAN_POINT('Ctrl Pts',(-0.755220979975262,-1.,1.7619781724032));
#23554=CARTESIAN_POINT('Ctrl Pts',(-0.755220979975262,1.,1.7619781724032));
#23555=CARTESIAN_POINT('Ctrl Pts',(-0.756421896028403,-1.,1.76789396003141));
#23556=CARTESIAN_POINT('Ctrl Pts',(-0.756421896028403,1.,1.76789396003141));
#23557=CARTESIAN_POINT('Ctrl Pts',(-0.757578264077238,-1.,1.77394167108342));
#23558=CARTESIAN_POINT('Ctrl Pts',(-0.757578264077238,1.,1.77394167108342));
#23559=CARTESIAN_POINT('Ctrl Pts',(-0.75865062667738,-1.,1.77999411220912));
#23560=CARTESIAN_POINT('Ctrl Pts',(-0.75865062667738,1.,1.77999411220912));
#23561=CARTESIAN_POINT('Ctrl Pts',(-0.759614401109868,-1.,1.78596964884526));
#23562=CARTESIAN_POINT('Ctrl Pts',(-0.759614401109868,1.,1.78596964884526));
#23563=CARTESIAN_POINT('Ctrl Pts',(-0.760469555880425,-1.,1.79185815610802));
#23564=CARTESIAN_POINT('Ctrl Pts',(-0.760469555880425,1.,1.79185815610802));
#23565=CARTESIAN_POINT('Ctrl Pts',(-0.761229695230359,-1.,1.79768986997735));
#23566=CARTESIAN_POINT('Ctrl Pts',(-0.761229695230359,1.,1.79768986997735));
#23567=CARTESIAN_POINT('Ctrl Pts',(-0.761915336443516,-1.,1.80351583877334));
#23568=CARTESIAN_POINT('Ctrl Pts',(-0.761915336443516,1.,1.80351583877334));
#23569=CARTESIAN_POINT('Ctrl Pts',(-0.762546129464036,-1.,1.80938551463989));
#23570=CARTESIAN_POINT('Ctrl Pts',(-0.762546129464036,1.,1.80938551463989));
#23571=CARTESIAN_POINT('Ctrl Pts',(-0.763132003836783,-1.,1.81532118405566));
#23572=CARTESIAN_POINT('Ctrl Pts',(-0.763132003836783,1.,1.81532118405566));
#23573=CARTESIAN_POINT('Ctrl Pts',(-0.763673465462854,-1.,1.82131873145297));
#23574=CARTESIAN_POINT('Ctrl Pts',(-0.763673465462854,1.,1.82131873145297));
#23575=CARTESIAN_POINT('Ctrl Pts',(-0.764165902606055,-1.,1.8273599120008));
#23576=CARTESIAN_POINT('Ctrl Pts',(-0.764165902606055,1.,1.8273599120008));
#23577=CARTESIAN_POINT('Ctrl Pts',(-0.764602549687845,-1.,1.8334207722714));
#23578=CARTESIAN_POINT('Ctrl Pts',(-0.764602549687845,1.,1.8334207722714));
#23579=CARTESIAN_POINT('Ctrl Pts',(-0.764978057881687,-1.,1.83948181064823));
#23580=CARTESIAN_POINT('Ctrl Pts',(-0.764978057881687,1.,1.83948181064823));
#23581=CARTESIAN_POINT('Ctrl Pts',(-0.765291664861971,-1.,1.8455369887591));
#23582=CARTESIAN_POINT('Ctrl Pts',(-0.765291664861971,1.,1.8455369887591));
#23583=CARTESIAN_POINT('Ctrl Pts',(-0.765545710619023,-1.,1.85158945130054));
#23584=CARTESIAN_POINT('Ctrl Pts',(-0.765545710619023,1.,1.85158945130054));
#23585=CARTESIAN_POINT('Ctrl Pts',(-0.765744212909305,-1.,1.85764741390391));
#23586=CARTESIAN_POINT('Ctrl Pts',(-0.765744212909305,1.,1.85764741390391));
#23587=CARTESIAN_POINT('Ctrl Pts',(-0.765891519092557,-1.,1.86372027063314));
#23588=CARTESIAN_POINT('Ctrl Pts',(-0.765891519092557,1.,1.86372027063314));
#23589=CARTESIAN_POINT('Ctrl Pts',(-0.765990708546111,-1.,1.86981398314345));
#23590=CARTESIAN_POINT('Ctrl Pts',(-0.765990708546111,1.,1.86981398314345));
#23591=CARTESIAN_POINT('Ctrl Pts',(-0.766042837036759,-1.,1.87592888967886));
#23592=CARTESIAN_POINT('Ctrl Pts',(-0.766042837036759,1.,1.87592888967886));
#23593=CARTESIAN_POINT('Ctrl Pts',(-0.766047794851869,-1.,1.88206215302561));
#23594=CARTESIAN_POINT('Ctrl Pts',(-0.766047794851869,1.,1.88206215302561));
#23595=CARTESIAN_POINT('Ctrl Pts',(-0.76600483706209,-1.,1.88820926433409));
#23596=CARTESIAN_POINT('Ctrl Pts',(-0.76600483706209,1.,1.88820926433409));
#23597=CARTESIAN_POINT('Ctrl Pts',(-0.765913193856979,-1.,1.89436577771389));
#23598=CARTESIAN_POINT('Ctrl Pts',(-0.765913193856979,1.,1.89436577771389));
#23599=CARTESIAN_POINT('Ctrl Pts',(-0.765772772593395,-1.,1.90052930393599));
#23600=CARTESIAN_POINT('Ctrl Pts',(-0.765772772593395,1.,1.90052930393599));
#23601=CARTESIAN_POINT('Ctrl Pts',(-0.765584196937936,-1.,1.90669961402362));
#23602=CARTESIAN_POINT('Ctrl Pts',(-0.765584196937936,1.,1.90669961402362));
#23603=CARTESIAN_POINT('Ctrl Pts',(-0.765348465884739,-1.,1.91287765805174));
#23604=CARTESIAN_POINT('Ctrl Pts',(-0.765348465884739,1.,1.91287765805174));
#23605=CARTESIAN_POINT('Ctrl Pts',(-0.765066729667095,-1.,1.91906491634197));
#23606=CARTESIAN_POINT('Ctrl Pts',(-0.765066729667095,1.,1.91906491634197));
#23607=CARTESIAN_POINT('Ctrl Pts',(-0.764740025488189,-1.,1.92526263537041));
#23608=CARTESIAN_POINT('Ctrl Pts',(-0.764740025488189,1.,1.92526263537041));
#23609=CARTESIAN_POINT('Ctrl Pts',(-0.764369010673889,-1.,1.93147105496367));
#23610=CARTESIAN_POINT('Ctrl Pts',(-0.764369010673889,1.,1.93147105496367));
#23611=CARTESIAN_POINT('Ctrl Pts',(-0.763954049121393,-1.,1.93768964875867));
#23612=CARTESIAN_POINT('Ctrl Pts',(-0.763954049121393,1.,1.93768964875867));
#23613=CARTESIAN_POINT('Ctrl Pts',(-0.76349533353858,-1.,1.94391746617626));
#23614=CARTESIAN_POINT('Ctrl Pts',(-0.76349533353858,1.,1.94391746617626));
#23615=CARTESIAN_POINT('Ctrl Pts',(-0.762992990878774,-1.,1.95015342590025));
#23616=CARTESIAN_POINT('Ctrl Pts',(-0.762992990878774,1.,1.95015342590025));
#23617=CARTESIAN_POINT('Ctrl Pts',(-0.762447203806263,-1.,1.95639665309893));
#23618=CARTESIAN_POINT('Ctrl Pts',(-0.762447203806263,1.,1.95639665309893));
#23619=CARTESIAN_POINT('Ctrl Pts',(-0.761858300014575,-1.,1.96264672744229));
#23620=CARTESIAN_POINT('Ctrl Pts',(-0.761858300014575,1.,1.96264672744229));
#23621=CARTESIAN_POINT('Ctrl Pts',(-0.761226690483986,-1.,1.96890351582545));
#23622=CARTESIAN_POINT('Ctrl Pts',(-0.761226690483986,1.,1.96890351582545));
#23623=CARTESIAN_POINT('Ctrl Pts',(-0.760552825409855,-1.,1.97516705321521));
#23624=CARTESIAN_POINT('Ctrl Pts',(-0.760552825409855,1.,1.97516705321521));
#23625=CARTESIAN_POINT('Ctrl Pts',(-0.759837147452135,-1.,1.98143741418156));
#23626=CARTESIAN_POINT('Ctrl Pts',(-0.759837147452135,1.,1.98143741418156));
#23627=CARTESIAN_POINT('Ctrl Pts',(-0.759080037802243,-1.,1.98771456680806));
#23628=CARTESIAN_POINT('Ctrl Pts',(-0.759080037802243,1.,1.98771456680806));
#23629=CARTESIAN_POINT('Ctrl Pts',(-0.758281796766377,-1.,1.9939983109871));
#23630=CARTESIAN_POINT('Ctrl Pts',(-0.758281796766377,1.,1.9939983109871));
#23631=CARTESIAN_POINT('Ctrl Pts',(-0.757442676862341,-1.,2.00028834739072));
#23632=CARTESIAN_POINT('Ctrl Pts',(-0.757442676862341,1.,2.00028834739072));
#23633=CARTESIAN_POINT('Ctrl Pts',(-0.756562904646496,-1.,2.00658431587682));
#23634=CARTESIAN_POINT('Ctrl Pts',(-0.756562904646496,1.,2.00658431587682));
#23635=CARTESIAN_POINT('Ctrl Pts',(-0.7556427049581,-1.,2.01288584328149));
#23636=CARTESIAN_POINT('Ctrl Pts',(-0.7556427049581,1.,2.01288584328149));
#23637=CARTESIAN_POINT('Ctrl Pts',(-0.75468233072352,-1.,2.01919259406003));
#23638=CARTESIAN_POINT('Ctrl Pts',(-0.75468233072352,1.,2.01919259406003));
#23639=CARTESIAN_POINT('Ctrl Pts',(-0.753682061113766,-1.,2.02550428623587));
#23640=CARTESIAN_POINT('Ctrl Pts',(-0.753682061113766,1.,2.02550428623587));
#23641=CARTESIAN_POINT('Ctrl Pts',(-0.752642180488104,-1.,2.03182068456467));
#23642=CARTESIAN_POINT('Ctrl Pts',(-0.752642180488104,1.,2.03182068456467));
#23643=CARTESIAN_POINT('Ctrl Pts',(-0.751562963361384,-1.,2.03814160092173));
#23644=CARTESIAN_POINT('Ctrl Pts',(-0.751562963361384,1.,2.03814160092173));
#23645=CARTESIAN_POINT('Ctrl Pts',(-0.750444657874758,-1.,2.04446689147754));
#23646=CARTESIAN_POINT('Ctrl Pts',(-0.750444657874758,1.,2.04446689147754));
#23647=CARTESIAN_POINT('Ctrl Pts',(-0.749287468663053,-1.,2.05079645591606));
#23648=CARTESIAN_POINT('Ctrl Pts',(-0.749287468663053,1.,2.05079645591606));
#23649=CARTESIAN_POINT('Ctrl Pts',(-0.748091554181101,-1.,2.05713023030263));
#23650=CARTESIAN_POINT('Ctrl Pts',(-0.748091554181101,1.,2.05713023030263));
#23651=CARTESIAN_POINT('Ctrl Pts',(-0.747103932785504,-1.,2.06220058927162));
#23652=CARTESIAN_POINT('Ctrl Pts',(-0.747103932785504,1.,2.06220058927162));
#23653=CARTESIAN_POINT('Ctrl Pts',(-0.746345871542696,-1.,2.06600523016401));
#23654=CARTESIAN_POINT('Ctrl Pts',(-0.746345871542696,1.,2.06600523016401));
#23655=CARTESIAN_POINT('Ctrl Pts',(-0.74583279137781,-1.,2.06854248895575));
#23656=CARTESIAN_POINT('Ctrl Pts',(-0.74583279137781,1.,2.06854248895575));
#23657=CARTESIAN_POINT('Ctrl Pts',(-0.745574324794401,-1.,2.0698113262342));
#23658=CARTESIAN_POINT('Ctrl Pts',(-0.745574324794401,1.,2.0698113262342));
#23659=CARTESIAN_POINT('',(-0.693717979106306,1.,1.60662857109684));
#23660=CARTESIAN_POINT('Ctrl Pts',(-0.693717979106306,1.,1.60662857109684));
#23661=CARTESIAN_POINT('Ctrl Pts',(-0.695712097881194,1.,1.61106790958151));
#23662=CARTESIAN_POINT('Ctrl Pts',(-0.699605146405088,1.,1.61974673472612));
#23663=CARTESIAN_POINT('Ctrl Pts',(-0.705159151988319,1.,1.63216541664676));
#23664=CARTESIAN_POINT('Ctrl Pts',(-0.711993139355394,1.,1.64752408832016));
#23665=CARTESIAN_POINT('Ctrl Pts',(-0.719585433804282,1.,1.6647288055568));
#23666=CARTESIAN_POINT('Ctrl Pts',(-0.726235967997433,1.,1.67996158455503));
#23667=CARTESIAN_POINT('Ctrl Pts',(-0.731963238697195,1.,1.69326921975743));
#23668=CARTESIAN_POINT('Ctrl Pts',(-0.736799665724771,1.,1.70473309006121));
#23669=CARTESIAN_POINT('Ctrl Pts',(-0.740795162032088,1.,1.71447789751927));
#23670=CARTESIAN_POINT('Ctrl Pts',(-0.744021445433764,1.,1.7226822991693));
#23671=CARTESIAN_POINT('Ctrl Pts',(-0.746574710096436,1.,1.72958533647399));
#23672=CARTESIAN_POINT('Ctrl Pts',(-0.748582462954855,1.,1.73550351679848));
#23673=CARTESIAN_POINT('Ctrl Pts',(-0.75019343597954,1.,1.74080458266705));
#23674=CARTESIAN_POINT('Ctrl Pts',(-0.751555614163629,1.,1.74585086852298));
#23675=CARTESIAN_POINT('Ctrl Pts',(-0.752797683531377,1.,1.75095139468809));
#23676=CARTESIAN_POINT('Ctrl Pts',(-0.75400925402848,1.,1.75631083600175));
#23677=CARTESIAN_POINT('Ctrl Pts',(-0.755220979975262,1.,1.7619781724032));
#23678=CARTESIAN_POINT('Ctrl Pts',(-0.756421896028403,1.,1.76789396003141));
#23679=CARTESIAN_POINT('Ctrl Pts',(-0.757578264077238,1.,1.77394167108342));
#23680=CARTESIAN_POINT('Ctrl Pts',(-0.75865062667738,1.,1.77999411220912));
#23681=CARTESIAN_POINT('Ctrl Pts',(-0.759614401109868,1.,1.78596964884526));
#23682=CARTESIAN_POINT('Ctrl Pts',(-0.760469555880425,1.,1.79185815610802));
#23683=CARTESIAN_POINT('Ctrl Pts',(-0.761229695230359,1.,1.79768986997735));
#23684=CARTESIAN_POINT('Ctrl Pts',(-0.761915336443516,1.,1.80351583877334));
#23685=CARTESIAN_POINT('Ctrl Pts',(-0.762546129464036,1.,1.80938551463989));
#23686=CARTESIAN_POINT('Ctrl Pts',(-0.763132003836783,1.,1.81532118405566));
#23687=CARTESIAN_POINT('Ctrl Pts',(-0.763673465462854,1.,1.82131873145297));
#23688=CARTESIAN_POINT('Ctrl Pts',(-0.764165902606055,1.,1.8273599120008));
#23689=CARTESIAN_POINT('Ctrl Pts',(-0.764602549687845,1.,1.8334207722714));
#23690=CARTESIAN_POINT('Ctrl Pts',(-0.764978057881687,1.,1.83948181064823));
#23691=CARTESIAN_POINT('Ctrl Pts',(-0.765291664861971,1.,1.8455369887591));
#23692=CARTESIAN_POINT('Ctrl Pts',(-0.765545710619023,1.,1.85158945130054));
#23693=CARTESIAN_POINT('Ctrl Pts',(-0.765744212909305,1.,1.85764741390391));
#23694=CARTESIAN_POINT('Ctrl Pts',(-0.765891519092557,1.,1.86372027063314));
#23695=CARTESIAN_POINT('Ctrl Pts',(-0.765990708546111,1.,1.86981398314345));
#23696=CARTESIAN_POINT('Ctrl Pts',(-0.766042837036759,1.,1.87592888967886));
#23697=CARTESIAN_POINT('Ctrl Pts',(-0.766047794851869,1.,1.88206215302561));
#23698=CARTESIAN_POINT('Ctrl Pts',(-0.76600483706209,1.,1.88820926433409));
#23699=CARTESIAN_POINT('Ctrl Pts',(-0.765913193856979,1.,1.89436577771389));
#23700=CARTESIAN_POINT('Ctrl Pts',(-0.765772772593395,1.,1.90052930393599));
#23701=CARTESIAN_POINT('Ctrl Pts',(-0.765584196937936,1.,1.90669961402362));
#23702=CARTESIAN_POINT('Ctrl Pts',(-0.765348465884739,1.,1.91287765805174));
#23703=CARTESIAN_POINT('Ctrl Pts',(-0.765066729667095,1.,1.91906491634197));
#23704=CARTESIAN_POINT('Ctrl Pts',(-0.764740025488189,1.,1.92526263537041));
#23705=CARTESIAN_POINT('Ctrl Pts',(-0.764369010673889,1.,1.93147105496367));
#23706=CARTESIAN_POINT('Ctrl Pts',(-0.763954049121393,1.,1.93768964875867));
#23707=CARTESIAN_POINT('Ctrl Pts',(-0.76349533353858,1.,1.94391746617626));
#23708=CARTESIAN_POINT('Ctrl Pts',(-0.762992990878774,1.,1.95015342590025));
#23709=CARTESIAN_POINT('Ctrl Pts',(-0.762447203806263,1.,1.95639665309893));
#23710=CARTESIAN_POINT('Ctrl Pts',(-0.761858300014575,1.,1.96264672744229));
#23711=CARTESIAN_POINT('Ctrl Pts',(-0.761226690483986,1.,1.96890351582545));
#23712=CARTESIAN_POINT('Ctrl Pts',(-0.760552825409855,1.,1.97516705321521));
#23713=CARTESIAN_POINT('Ctrl Pts',(-0.759837147452135,1.,1.98143741418156));
#23714=CARTESIAN_POINT('Ctrl Pts',(-0.759080037802243,1.,1.98771456680806));
#23715=CARTESIAN_POINT('Ctrl Pts',(-0.758281796766377,1.,1.9939983109871));
#23716=CARTESIAN_POINT('Ctrl Pts',(-0.757442676862341,1.,2.00028834739072));
#23717=CARTESIAN_POINT('Ctrl Pts',(-0.756562904646496,1.,2.00658431587682));
#23718=CARTESIAN_POINT('Ctrl Pts',(-0.7556427049581,1.,2.01288584328149));
#23719=CARTESIAN_POINT('Ctrl Pts',(-0.75468233072352,1.,2.01919259406003));
#23720=CARTESIAN_POINT('Ctrl Pts',(-0.753682061113766,1.,2.02550428623587));
#23721=CARTESIAN_POINT('Ctrl Pts',(-0.752642180488104,1.,2.03182068456467));
#23722=CARTESIAN_POINT('Ctrl Pts',(-0.751562963361384,1.,2.03814160092173));
#23723=CARTESIAN_POINT('Ctrl Pts',(-0.750444657874758,1.,2.04446689147754));
#23724=CARTESIAN_POINT('Ctrl Pts',(-0.749287468663053,1.,2.05079645591606));
#23725=CARTESIAN_POINT('Ctrl Pts',(-0.748091554181101,1.,2.05713023030263));
#23726=CARTESIAN_POINT('Ctrl Pts',(-0.747103932785504,1.,2.06220058927162));
#23727=CARTESIAN_POINT('Ctrl Pts',(-0.746345871542696,1.,2.06600523016401));
#23728=CARTESIAN_POINT('Ctrl Pts',(-0.74583279137781,1.,2.06854248895575));
#23729=CARTESIAN_POINT('Ctrl Pts',(-0.745574324794401,1.,2.0698113262342));
#23730=CARTESIAN_POINT('',(-0.693717979106306,0.,1.60662857109684));
#23731=CARTESIAN_POINT('Origin',(0.,0.,0.));
#23732=CARTESIAN_POINT('',(-0.892032620296855,1.,1.5055822144029));
#23733=CARTESIAN_POINT('Origin',(0.,1.,0.));
#23734=CARTESIAN_POINT('',(-0.892032620296855,0.,1.5055822144029));
#23735=CARTESIAN_POINT('Ctrl Pts',(-1.23627494547115,-1.,1.81978687191668));
#23736=CARTESIAN_POINT('Ctrl Pts',(-1.23627494547115,1.,1.81978687191668));
#23737=CARTESIAN_POINT('Ctrl Pts',(-1.23509651170476,-1.,1.81925017193666));
#23738=CARTESIAN_POINT('Ctrl Pts',(-1.23509651170476,1.,1.81925017193666));
#23739=CARTESIAN_POINT('Ctrl Pts',(-1.2327422452705,-1.,1.81817389921279));
#23740=CARTESIAN_POINT('Ctrl Pts',(-1.2327422452705,1.,1.81817389921279));
#23741=CARTESIAN_POINT('Ctrl Pts',(-1.2292186489137,-1.,1.8165508718364));
#23742=CARTESIAN_POINT('Ctrl Pts',(-1.2292186489137,1.,1.8165508718364));
#23743=CARTESIAN_POINT('Ctrl Pts',(-1.2245361330495,-1.,1.81436959210434));
#23744=CARTESIAN_POINT('Ctrl Pts',(-1.2245361330495,1.,1.81436959210434));
#23745=CARTESIAN_POINT('Ctrl Pts',(-1.21870906103557,-1.,1.81161420806656));
#23746=CARTESIAN_POINT('Ctrl Pts',(-1.21870906103557,1.,1.81161420806656));
#23747=CARTESIAN_POINT('Ctrl Pts',(-1.21290815708314,-1.,1.80882996917129));
#23748=CARTESIAN_POINT('Ctrl Pts',(-1.21290815708314,1.,1.80882996917129));
#23749=CARTESIAN_POINT('Ctrl Pts',(-1.20713356605475,-1.,1.80601678480707));
#23750=CARTESIAN_POINT('Ctrl Pts',(-1.20713356605475,1.,1.80601678480707));
#23751=CARTESIAN_POINT('Ctrl Pts',(-1.20138548938974,-1.,1.80317454838603));
#23752=CARTESIAN_POINT('Ctrl Pts',(-1.20138548938974,1.,1.80317454838603));
#23753=CARTESIAN_POINT('Ctrl Pts',(-1.19566418930242,-1.,1.80030314369879));
#23754=CARTESIAN_POINT('Ctrl Pts',(-1.19566418930242,1.,1.80030314369879));
#23755=CARTESIAN_POINT('Ctrl Pts',(-1.18996997934445,-1.,1.79740245923478));
#23756=CARTESIAN_POINT('Ctrl Pts',(-1.18996997934445,1.,1.79740245923478));
#23757=CARTESIAN_POINT('Ctrl Pts',(-1.18430321697432,-1.,1.79447240321515));
#23758=CARTESIAN_POINT('Ctrl Pts',(-1.18430321697432,1.,1.79447240321515));
#23759=CARTESIAN_POINT('Ctrl Pts',(-1.17866429440809,-1.,1.79151291552689));
#23760=CARTESIAN_POINT('Ctrl Pts',(-1.17866429440809,1.,1.79151291552689));
#23761=CARTESIAN_POINT('Ctrl Pts',(-1.17305363177328,-1.,1.78852398877616));
#23762=CARTESIAN_POINT('Ctrl Pts',(-1.17305363177328,1.,1.78852398877616));
#23763=CARTESIAN_POINT('Ctrl Pts',(-1.16747166312303,-1.,1.78550566040443));
#23764=CARTESIAN_POINT('Ctrl Pts',(-1.16747166312303,1.,1.78550566040443));
#23765=CARTESIAN_POINT('Ctrl Pts',(-1.16191881298499,-1.,1.78245795881009));
#23766=CARTESIAN_POINT('Ctrl Pts',(-1.16191881298499,1.,1.78245795881009));
#23767=CARTESIAN_POINT('Ctrl Pts',(-1.15639547194698,-1.,1.77938085564275));
#23768=CARTESIAN_POINT('Ctrl Pts',(-1.15639547194698,1.,1.77938085564275));
#23769=CARTESIAN_POINT('Ctrl Pts',(-1.15090197841515,-1.,1.7762742255701));
#23770=CARTESIAN_POINT('Ctrl Pts',(-1.15090197841515,1.,1.7762742255701));
#23771=CARTESIAN_POINT('Ctrl Pts',(-1.1454385822692,-1.,1.77313777896194));
#23772=CARTESIAN_POINT('Ctrl Pts',(-1.1454385822692,1.,1.77313777896194));
#23773=CARTESIAN_POINT('Ctrl Pts',(-1.14000548336975,-1.,1.76997111386769));
#23774=CARTESIAN_POINT('Ctrl Pts',(-1.14000548336975,1.,1.76997111386769));
#23775=CARTESIAN_POINT('Ctrl Pts',(-1.1346029180462,-1.,1.76677384551862));
#23776=CARTESIAN_POINT('Ctrl Pts',(-1.1346029180462,1.,1.76677384551862));
#23777=CARTESIAN_POINT('Ctrl Pts',(-1.12923123555075,-1.,1.7635457196617));
#23778=CARTESIAN_POINT('Ctrl Pts',(-1.12923123555075,1.,1.7635457196617));
#23779=CARTESIAN_POINT('Ctrl Pts',(-1.12389096855086,-1.,1.76028671825096));
#23780=CARTESIAN_POINT('Ctrl Pts',(-1.12389096855086,1.,1.76028671825096));
#23781=CARTESIAN_POINT('Ctrl Pts',(-1.11858293216763,-1.,1.75699720772105));
#23782=CARTESIAN_POINT('Ctrl Pts',(-1.11858293216763,1.,1.75699720772105));
#23783=CARTESIAN_POINT('Ctrl Pts',(-1.11330807582551,-1.,1.7536777209463));
#23784=CARTESIAN_POINT('Ctrl Pts',(-1.11330807582551,1.,1.7536777209463));
#23785=CARTESIAN_POINT('Ctrl Pts',(-1.10806728183007,-1.,1.7503286607592));
#23786=CARTESIAN_POINT('Ctrl Pts',(-1.10806728183007,1.,1.7503286607592));
#23787=CARTESIAN_POINT('Ctrl Pts',(-1.10286118991143,-1.,1.74695004214923));
#23788=CARTESIAN_POINT('Ctrl Pts',(-1.10286118991143,1.,1.74695004214923));
#23789=CARTESIAN_POINT('Ctrl Pts',(-1.09768999241225,-1.,1.74354119236208));
#23790=CARTESIAN_POINT('Ctrl Pts',(-1.09768999241225,1.,1.74354119236208));
#23791=CARTESIAN_POINT('Ctrl Pts',(-1.09255329056493,-1.,1.74010053962247));
#23792=CARTESIAN_POINT('Ctrl Pts',(-1.09255329056493,1.,1.74010053962247));
#23793=CARTESIAN_POINT('Ctrl Pts',(-1.08745056285427,-1.,1.73662628326091));
#23794=CARTESIAN_POINT('Ctrl Pts',(-1.08745056285427,1.,1.73662628326091));
#23795=CARTESIAN_POINT('Ctrl Pts',(-1.08238162784749,-1.,1.73311705663407));
#23796=CARTESIAN_POINT('Ctrl Pts',(-1.08238162784749,1.,1.73311705663407));
#23797=CARTESIAN_POINT('Ctrl Pts',(-1.0773470373727,-1.,1.72957248977424));
#23798=CARTESIAN_POINT('Ctrl Pts',(-1.0773470373727,1.,1.72957248977424));
#23799=CARTESIAN_POINT('Ctrl Pts',(-1.07234866990252,-1.,1.72599406198488));
#23800=CARTESIAN_POINT('Ctrl Pts',(-1.07234866990252,1.,1.72599406198488));
#23801=CARTESIAN_POINT('Ctrl Pts',(-1.06738966975462,-1.,1.72238500928453));
#23802=CARTESIAN_POINT('Ctrl Pts',(-1.06738966975462,1.,1.72238500928453));
#23803=CARTESIAN_POINT('Ctrl Pts',(-1.06247324680647,-1.,1.71874858456904));
#23804=CARTESIAN_POINT('Ctrl Pts',(-1.06247324680647,1.,1.71874858456904));
#23805=CARTESIAN_POINT('Ctrl Pts',(-1.05760163192479,-1.,1.7150865442702));
#23806=CARTESIAN_POINT('Ctrl Pts',(-1.05760163192479,1.,1.7150865442702));
#23807=CARTESIAN_POINT('Ctrl Pts',(-1.05277517202855,-1.,1.71139783543989));
#23808=CARTESIAN_POINT('Ctrl Pts',(-1.05277517202855,1.,1.71139783543989));
#23809=CARTESIAN_POINT('Ctrl Pts',(-1.04799085404995,-1.,1.70767646263649));
#23810=CARTESIAN_POINT('Ctrl Pts',(-1.04799085404995,1.,1.70767646263649));
#23811=CARTESIAN_POINT('Ctrl Pts',(-1.04324363334554,-1.,1.70391338707982));
#23812=CARTESIAN_POINT('Ctrl Pts',(-1.04324363334554,1.,1.70391338707982));
#23813=CARTESIAN_POINT('Ctrl Pts',(-1.03852922490789,-1.,1.70010052930962));
#23814=CARTESIAN_POINT('Ctrl Pts',(-1.03852922490789,1.,1.70010052930962));
#23815=CARTESIAN_POINT('Ctrl Pts',(-1.03384646003588,-1.,1.69623414782771));
#23816=CARTESIAN_POINT('Ctrl Pts',(-1.03384646003588,1.,1.69623414782771));
#23817=CARTESIAN_POINT('Ctrl Pts',(-1.02919977579147,-1.,1.69231840863458));
#23818=CARTESIAN_POINT('Ctrl Pts',(-1.02919977579147,1.,1.69231840863458));
#23819=CARTESIAN_POINT('Ctrl Pts',(-1.02460180535255,-1.,1.68836910178447));
#23820=CARTESIAN_POINT('Ctrl Pts',(-1.02460180535255,1.,1.68836910178447));
#23821=CARTESIAN_POINT('Ctrl Pts',(-1.02006795074201,-1.,1.68440578021706));
#23822=CARTESIAN_POINT('Ctrl Pts',(-1.02006795074201,1.,1.68440578021706));
#23823=CARTESIAN_POINT('Ctrl Pts',(-1.01561026162773,-1.,1.68044289894798));
#23824=CARTESIAN_POINT('Ctrl Pts',(-1.01561026162773,1.,1.68044289894798));
#23825=CARTESIAN_POINT('Ctrl Pts',(-1.01123236493511,-1.,1.67648246776464));
#23826=CARTESIAN_POINT('Ctrl Pts',(-1.01123236493511,1.,1.67648246776464));
#23827=CARTESIAN_POINT('Ctrl Pts',(-1.00692206696414,-1.,1.67250335383293));
#23828=CARTESIAN_POINT('Ctrl Pts',(-1.00692206696414,1.,1.67250335383293));
#23829=CARTESIAN_POINT('Ctrl Pts',(-1.00265091003727,-1.,1.66846059277303));
#23830=CARTESIAN_POINT('Ctrl Pts',(-1.00265091003727,1.,1.66846059277303));
#23831=CARTESIAN_POINT('Ctrl Pts',(-0.998389654952758,-1.,1.66430758030376));
#23832=CARTESIAN_POINT('Ctrl Pts',(-0.998389654952758,1.,1.66430758030376));
#23833=CARTESIAN_POINT('Ctrl Pts',(-0.994121836661306,-1.,1.66001553809947));
#23834=CARTESIAN_POINT('Ctrl Pts',(-0.994121836661306,1.,1.66001553809947));
#23835=CARTESIAN_POINT('Ctrl Pts',(-0.989855627854165,-1.,1.65559044289699));
#23836=CARTESIAN_POINT('Ctrl Pts',(-0.989855627854165,1.,1.65559044289699));
#23837=CARTESIAN_POINT('Ctrl Pts',(-0.985642622920821,-1.,1.65110016612638));
#23838=CARTESIAN_POINT('Ctrl Pts',(-0.985642622920821,1.,1.65110016612638));
#23839=CARTESIAN_POINT('Ctrl Pts',(-0.981562530939489,-1.,1.64665139190656));
#23840=CARTESIAN_POINT('Ctrl Pts',(-0.981562530939489,1.,1.64665139190656));
#23841=CARTESIAN_POINT('Ctrl Pts',(-0.977689794119416,-1.,1.64233990826687));
#23842=CARTESIAN_POINT('Ctrl Pts',(-0.977689794119416,1.,1.64233990826687));
#23843=CARTESIAN_POINT('Ctrl Pts',(-0.974066058287418,-1.,1.63820952658144));
#23844=CARTESIAN_POINT('Ctrl Pts',(-0.974066058287418,1.,1.63820952658144));
#23845=CARTESIAN_POINT('Ctrl Pts',(-0.970669715997509,-1.,1.63420665729798));
#23846=CARTESIAN_POINT('Ctrl Pts',(-0.970669715997509,1.,1.63420665729798));
#23847=CARTESIAN_POINT('Ctrl Pts',(-0.967387853230345,-1.,1.63013849959461));
#23848=CARTESIAN_POINT('Ctrl Pts',(-0.967387853230345,1.,1.63013849959461));
#23849=CARTESIAN_POINT('Ctrl Pts',(-0.964046107040536,-1.,1.62571930670187));
#23850=CARTESIAN_POINT('Ctrl Pts',(-0.964046107040536,1.,1.62571930670187));
#23851=CARTESIAN_POINT('Ctrl Pts',(-0.960438326101729,-1.,1.62061638140221));
#23852=CARTESIAN_POINT('Ctrl Pts',(-0.960438326101729,1.,1.62061638140221));
#23853=CARTESIAN_POINT('Ctrl Pts',(-0.956354422920671,-1.,1.61449324337085));
#23854=CARTESIAN_POINT('Ctrl Pts',(-0.956354422920671,1.,1.61449324337085));
#23855=CARTESIAN_POINT('Ctrl Pts',(-0.951613284356035,-1.,1.60706069896936));
#23856=CARTESIAN_POINT('Ctrl Pts',(-0.951613284356035,1.,1.60706069896936));
#23857=CARTESIAN_POINT('Ctrl Pts',(-0.946078063315257,-1.,1.59810042043673));
#23858=CARTESIAN_POINT('Ctrl Pts',(-0.946078063315257,1.,1.59810042043673));
#23859=CARTESIAN_POINT('Ctrl Pts',(-0.939646377893399,-1.,1.58744937487176));
#23860=CARTESIAN_POINT('Ctrl Pts',(-0.939646377893399,1.,1.58744937487176));
#23861=CARTESIAN_POINT('Ctrl Pts',(-0.932246680108685,-1.,1.57499388382243));
#23862=CARTESIAN_POINT('Ctrl Pts',(-0.932246680108685,1.,1.57499388382243));
#23863=CARTESIAN_POINT('Ctrl Pts',(-0.923832188944341,-1.,1.56065988578893));
#23864=CARTESIAN_POINT('Ctrl Pts',(-0.923832188944341,1.,1.56065988578893));
#23865=CARTESIAN_POINT('Ctrl Pts',(-0.914375919026456,-1.,1.54440491149498));
#23866=CARTESIAN_POINT('Ctrl Pts',(-0.914375919026456,1.,1.54440491149498));
#23867=CARTESIAN_POINT('Ctrl Pts',(-0.905967409625651,-1.,1.52984849887993));
#23868=CARTESIAN_POINT('Ctrl Pts',(-0.905967409625651,1.,1.52984849887993));
#23869=CARTESIAN_POINT('Ctrl Pts',(-0.899185047483511,-1.,1.51805569590094));
#23870=CARTESIAN_POINT('Ctrl Pts',(-0.899185047483511,1.,1.51805569590094));
#23871=CARTESIAN_POINT('Ctrl Pts',(-0.894452006964543,-1.,1.50980486806688));
#23872=CARTESIAN_POINT('Ctrl Pts',(-0.894452006964543,1.,1.50980486806688));
#23873=CARTESIAN_POINT('Ctrl Pts',(-0.892032620296855,-1.,1.5055822144029));
#23874=CARTESIAN_POINT('Ctrl Pts',(-0.892032620296855,1.,1.5055822144029));
#23875=CARTESIAN_POINT('',(-1.23627494547115,1.,1.81978687191668));
#23876=CARTESIAN_POINT('Ctrl Pts',(-1.23627494547115,1.,1.81978687191668));
#23877=CARTESIAN_POINT('Ctrl Pts',(-1.23509651170476,1.,1.81925017193666));
#23878=CARTESIAN_POINT('Ctrl Pts',(-1.2327422452705,1.,1.81817389921279));
#23879=CARTESIAN_POINT('Ctrl Pts',(-1.2292186489137,1.,1.8165508718364));
#23880=CARTESIAN_POINT('Ctrl Pts',(-1.2245361330495,1.,1.81436959210434));
#23881=CARTESIAN_POINT('Ctrl Pts',(-1.21870906103557,1.,1.81161420806656));
#23882=CARTESIAN_POINT('Ctrl Pts',(-1.21290815708314,1.,1.80882996917129));
#23883=CARTESIAN_POINT('Ctrl Pts',(-1.20713356605475,1.,1.80601678480707));
#23884=CARTESIAN_POINT('Ctrl Pts',(-1.20138548938974,1.,1.80317454838603));
#23885=CARTESIAN_POINT('Ctrl Pts',(-1.19566418930242,1.,1.80030314369879));
#23886=CARTESIAN_POINT('Ctrl Pts',(-1.18996997934445,1.,1.79740245923478));
#23887=CARTESIAN_POINT('Ctrl Pts',(-1.18430321697432,1.,1.79447240321515));
#23888=CARTESIAN_POINT('Ctrl Pts',(-1.17866429440809,1.,1.79151291552689));
#23889=CARTESIAN_POINT('Ctrl Pts',(-1.17305363177328,1.,1.78852398877616));
#23890=CARTESIAN_POINT('Ctrl Pts',(-1.16747166312303,1.,1.78550566040443));
#23891=CARTESIAN_POINT('Ctrl Pts',(-1.16191881298499,1.,1.78245795881009));
#23892=CARTESIAN_POINT('Ctrl Pts',(-1.15639547194698,1.,1.77938085564275));
#23893=CARTESIAN_POINT('Ctrl Pts',(-1.15090197841515,1.,1.7762742255701));
#23894=CARTESIAN_POINT('Ctrl Pts',(-1.1454385822692,1.,1.77313777896194));
#23895=CARTESIAN_POINT('Ctrl Pts',(-1.14000548336975,1.,1.76997111386769));
#23896=CARTESIAN_POINT('Ctrl Pts',(-1.1346029180462,1.,1.76677384551862));
#23897=CARTESIAN_POINT('Ctrl Pts',(-1.12923123555075,1.,1.7635457196617));
#23898=CARTESIAN_POINT('Ctrl Pts',(-1.12389096855086,1.,1.76028671825096));
#23899=CARTESIAN_POINT('Ctrl Pts',(-1.11858293216763,1.,1.75699720772105));
#23900=CARTESIAN_POINT('Ctrl Pts',(-1.11330807582551,1.,1.7536777209463));
#23901=CARTESIAN_POINT('Ctrl Pts',(-1.10806728183007,1.,1.7503286607592));
#23902=CARTESIAN_POINT('Ctrl Pts',(-1.10286118991143,1.,1.74695004214923));
#23903=CARTESIAN_POINT('Ctrl Pts',(-1.09768999241225,1.,1.74354119236208));
#23904=CARTESIAN_POINT('Ctrl Pts',(-1.09255329056493,1.,1.74010053962247));
#23905=CARTESIAN_POINT('Ctrl Pts',(-1.08745056285427,1.,1.73662628326091));
#23906=CARTESIAN_POINT('Ctrl Pts',(-1.08238162784749,1.,1.73311705663407));
#23907=CARTESIAN_POINT('Ctrl Pts',(-1.0773470373727,1.,1.72957248977424));
#23908=CARTESIAN_POINT('Ctrl Pts',(-1.07234866990252,1.,1.72599406198488));
#23909=CARTESIAN_POINT('Ctrl Pts',(-1.06738966975462,1.,1.72238500928453));
#23910=CARTESIAN_POINT('Ctrl Pts',(-1.06247324680647,1.,1.71874858456904));
#23911=CARTESIAN_POINT('Ctrl Pts',(-1.05760163192479,1.,1.7150865442702));
#23912=CARTESIAN_POINT('Ctrl Pts',(-1.05277517202855,1.,1.71139783543989));
#23913=CARTESIAN_POINT('Ctrl Pts',(-1.04799085404995,1.,1.70767646263649));
#23914=CARTESIAN_POINT('Ctrl Pts',(-1.04324363334554,1.,1.70391338707982));
#23915=CARTESIAN_POINT('Ctrl Pts',(-1.03852922490789,1.,1.70010052930962));
#23916=CARTESIAN_POINT('Ctrl Pts',(-1.03384646003588,1.,1.69623414782771));
#23917=CARTESIAN_POINT('Ctrl Pts',(-1.02919977579147,1.,1.69231840863458));
#23918=CARTESIAN_POINT('Ctrl Pts',(-1.02460180535255,1.,1.68836910178447));
#23919=CARTESIAN_POINT('Ctrl Pts',(-1.02006795074201,1.,1.68440578021706));
#23920=CARTESIAN_POINT('Ctrl Pts',(-1.01561026162773,1.,1.68044289894798));
#23921=CARTESIAN_POINT('Ctrl Pts',(-1.01123236493511,1.,1.67648246776464));
#23922=CARTESIAN_POINT('Ctrl Pts',(-1.00692206696414,1.,1.67250335383293));
#23923=CARTESIAN_POINT('Ctrl Pts',(-1.00265091003727,1.,1.66846059277303));
#23924=CARTESIAN_POINT('Ctrl Pts',(-0.998389654952758,1.,1.66430758030376));
#23925=CARTESIAN_POINT('Ctrl Pts',(-0.994121836661306,1.,1.66001553809947));
#23926=CARTESIAN_POINT('Ctrl Pts',(-0.989855627854165,1.,1.65559044289699));
#23927=CARTESIAN_POINT('Ctrl Pts',(-0.985642622920821,1.,1.65110016612638));
#23928=CARTESIAN_POINT('Ctrl Pts',(-0.981562530939489,1.,1.64665139190656));
#23929=CARTESIAN_POINT('Ctrl Pts',(-0.977689794119416,1.,1.64233990826687));
#23930=CARTESIAN_POINT('Ctrl Pts',(-0.974066058287418,1.,1.63820952658144));
#23931=CARTESIAN_POINT('Ctrl Pts',(-0.970669715997509,1.,1.63420665729798));
#23932=CARTESIAN_POINT('Ctrl Pts',(-0.967387853230345,1.,1.63013849959461));
#23933=CARTESIAN_POINT('Ctrl Pts',(-0.964046107040536,1.,1.62571930670187));
#23934=CARTESIAN_POINT('Ctrl Pts',(-0.960438326101729,1.,1.62061638140221));
#23935=CARTESIAN_POINT('Ctrl Pts',(-0.956354422920671,1.,1.61449324337085));
#23936=CARTESIAN_POINT('Ctrl Pts',(-0.951613284356035,1.,1.60706069896936));
#23937=CARTESIAN_POINT('Ctrl Pts',(-0.946078063315257,1.,1.59810042043673));
#23938=CARTESIAN_POINT('Ctrl Pts',(-0.939646377893399,1.,1.58744937487176));
#23939=CARTESIAN_POINT('Ctrl Pts',(-0.932246680108685,1.,1.57499388382243));
#23940=CARTESIAN_POINT('Ctrl Pts',(-0.923832188944341,1.,1.56065988578893));
#23941=CARTESIAN_POINT('Ctrl Pts',(-0.914375919026456,1.,1.54440491149498));
#23942=CARTESIAN_POINT('Ctrl Pts',(-0.905967409625651,1.,1.52984849887993));
#23943=CARTESIAN_POINT('Ctrl Pts',(-0.899185047483511,1.,1.51805569590094));
#23944=CARTESIAN_POINT('Ctrl Pts',(-0.894452006964543,1.,1.50980486806688));
#23945=CARTESIAN_POINT('Ctrl Pts',(-0.892032620296855,1.,1.5055822144029));
#23946=CARTESIAN_POINT('',(-1.23627494547115,0.,1.81978687191668));
#23947=CARTESIAN_POINT('Origin',(-1.34869019493419,0.,1.73811241238545));
#23948=CARTESIAN_POINT('',(-1.34869019493419,1.,1.73811241238545));
#23949=CARTESIAN_POINT('',(-1.23627494547115,1.,1.81978687191668));
#23950=CARTESIAN_POINT('',(-1.34869019493419,0.,1.73811241238545));
#23951=CARTESIAN_POINT('Ctrl Pts',(-1.15624053661742,-1.,1.31362392696032));
#23952=CARTESIAN_POINT('Ctrl Pts',(-1.15624053661742,1.,1.31362392696032));
#23953=CARTESIAN_POINT('Ctrl Pts',(-1.15950888730809,-1.,1.31722977216397));
#23954=CARTESIAN_POINT('Ctrl Pts',(-1.15950888730809,1.,1.31722977216397));
#23955=CARTESIAN_POINT('Ctrl Pts',(-1.16589330093588,-1.,1.32428080721772));
#23956=CARTESIAN_POINT('Ctrl Pts',(-1.16589330093588,1.,1.32428080721772));
#23957=CARTESIAN_POINT('Ctrl Pts',(-1.17501305789857,-1.,1.33437539347008));
#23958=CARTESIAN_POINT('Ctrl Pts',(-1.17501305789857,1.,1.33437539347008));
#23959=CARTESIAN_POINT('Ctrl Pts',(-1.18625865667441,-1.,1.34687054001093));
#23960=CARTESIAN_POINT('Ctrl Pts',(-1.18625865667441,1.,1.34687054001093));
#23961=CARTESIAN_POINT('Ctrl Pts',(-1.1987959077932,-1.,1.36088705043885));
#23962=CARTESIAN_POINT('Ctrl Pts',(-1.1987959077932,1.,1.36088705043885));
#23963=CARTESIAN_POINT('Ctrl Pts',(-1.20982812925645,-1.,1.37331915607905));
#23964=CARTESIAN_POINT('Ctrl Pts',(-1.20982812925645,1.,1.37331915607905));
#23965=CARTESIAN_POINT('Ctrl Pts',(-1.21938737280852,-1.,1.38420564527715));
#23966=CARTESIAN_POINT('Ctrl Pts',(-1.21938737280852,1.,1.38420564527715));
#23967=CARTESIAN_POINT('Ctrl Pts',(-1.22752961899387,-1.,1.39361389568796));
#23968=CARTESIAN_POINT('Ctrl Pts',(-1.22752961899387,1.,1.39361389568796));
#23969=CARTESIAN_POINT('Ctrl Pts',(-1.23434087290423,-1.,1.40164708206106));
#23970=CARTESIAN_POINT('Ctrl Pts',(-1.23434087290423,1.,1.40164708206106));
#23971=CARTESIAN_POINT('Ctrl Pts',(-1.23994455029534,-1.,1.40845295531283));
#23972=CARTESIAN_POINT('Ctrl Pts',(-1.23994455029534,1.,1.40845295531283));
#23973=CARTESIAN_POINT('Ctrl Pts',(-1.24450600513056,-1.,1.41422913175179));
#23974=CARTESIAN_POINT('Ctrl Pts',(-1.24450600513056,1.,1.41422913175179));
#23975=CARTESIAN_POINT('Ctrl Pts',(-1.24824430986571,-1.,1.41923722596025));
#23976=CARTESIAN_POINT('Ctrl Pts',(-1.24824430986571,1.,1.41923722596025));
#23977=CARTESIAN_POINT('Ctrl Pts',(-1.2514145557001,-1.,1.42378102115575));
#23978=CARTESIAN_POINT('Ctrl Pts',(-1.2514145557001,1.,1.42378102115575));
#23979=CARTESIAN_POINT('Ctrl Pts',(-1.25426945222639,-1.,1.42815938799387));
#23980=CARTESIAN_POINT('Ctrl Pts',(-1.25426945222639,1.,1.42815938799387));
#23981=CARTESIAN_POINT('Ctrl Pts',(-1.25702687965755,-1.,1.43262645609691));
#23982=CARTESIAN_POINT('Ctrl Pts',(-1.25702687965755,1.,1.43262645609691));
#23983=CARTESIAN_POINT('Ctrl Pts',(-1.25983531012005,-1.,1.43734919180848));
#23984=CARTESIAN_POINT('Ctrl Pts',(-1.25983531012005,1.,1.43734919180848));
#23985=CARTESIAN_POINT('Ctrl Pts',(-1.26273903323859,-1.,1.44236470511303));
#23986=CARTESIAN_POINT('Ctrl Pts',(-1.26273903323859,1.,1.44236470511303));
#23987=CARTESIAN_POINT('Ctrl Pts',(-1.26570925118868,-1.,1.44761985001662));
#23988=CARTESIAN_POINT('Ctrl Pts',(-1.26570925118868,1.,1.44761985001662));
#23989=CARTESIAN_POINT('Ctrl Pts',(-1.2686778680489,-1.,1.45301422764247));
#23990=CARTESIAN_POINT('Ctrl Pts',(-1.2686778680489,1.,1.45301422764247));
#23991=CARTESIAN_POINT('Ctrl Pts',(-1.27156805265289,-1.,1.45843906294697));
#23992=CARTESIAN_POINT('Ctrl Pts',(-1.27156805265289,1.,1.45843906294697));
#23993=CARTESIAN_POINT('Ctrl Pts',(-1.27433119897822,-1.,1.46382431332476));
#23994=CARTESIAN_POINT('Ctrl Pts',(-1.27433119897822,1.,1.46382431332476));
#23995=CARTESIAN_POINT('Ctrl Pts',(-1.27696414831089,-1.,1.46916035917133));
#23996=CARTESIAN_POINT('Ctrl Pts',(-1.27696414831089,1.,1.46916035917133));
#23997=CARTESIAN_POINT('Ctrl Pts',(-1.2794891824849,-1.,1.4744717526707));
#23998=CARTESIAN_POINT('Ctrl Pts',(-1.2794891824849,1.,1.4744717526707));
#23999=CARTESIAN_POINT('Ctrl Pts',(-1.28194158939517,-1.,1.47980070347095));
#24000=CARTESIAN_POINT('Ctrl Pts',(-1.28194158939517,1.,1.47980070347095));
#24001=CARTESIAN_POINT('Ctrl Pts',(-1.28435533880201,-1.,1.4851881711891));
#24002=CARTESIAN_POINT('Ctrl Pts',(-1.28435533880201,1.,1.4851881711891));
#24003=CARTESIAN_POINT('Ctrl Pts',(-1.2867467611644,-1.,1.4906522831278));
#24004=CARTESIAN_POINT('Ctrl Pts',(-1.2867467611644,1.,1.4906522831278));
#24005=CARTESIAN_POINT('Ctrl Pts',(-1.28911506584254,-1.,1.49618896881754));
#24006=CARTESIAN_POINT('Ctrl Pts',(-1.28911506584254,1.,1.49618896881754));
#24007=CARTESIAN_POINT('Ctrl Pts',(-1.29145022885181,-1.,1.50178230149776));
#24008=CARTESIAN_POINT('Ctrl Pts',(-1.29145022885181,1.,1.50178230149776));
#24009=CARTESIAN_POINT('Ctrl Pts',(-1.29373841372842,-1.,1.50741159078365));
#24010=CARTESIAN_POINT('Ctrl Pts',(-1.29373841372842,1.,1.50741159078365));
#24011=CARTESIAN_POINT('Ctrl Pts',(-1.29596850710509,-1.,1.51305994241402));
#24012=CARTESIAN_POINT('Ctrl Pts',(-1.29596850710509,1.,1.51305994241402));
#24013=CARTESIAN_POINT('Ctrl Pts',(-1.29813791800747,-1.,1.51872184912724));
#24014=CARTESIAN_POINT('Ctrl Pts',(-1.29813791800747,1.,1.51872184912724));
#24015=CARTESIAN_POINT('Ctrl Pts',(-1.30024984366328,-1.,1.52439957861062));
#24016=CARTESIAN_POINT('Ctrl Pts',(-1.30024984366328,1.,1.52439957861062));
#24017=CARTESIAN_POINT('Ctrl Pts',(-1.30231064395568,-1.,1.53009970283891));
#24018=CARTESIAN_POINT('Ctrl Pts',(-1.30231064395568,1.,1.53009970283891));
#24019=CARTESIAN_POINT('Ctrl Pts',(-1.30432735639489,-1.,1.53582981268977));
#24020=CARTESIAN_POINT('Ctrl Pts',(-1.30432735639489,1.,1.53582981268977));
#24021=CARTESIAN_POINT('Ctrl Pts',(-1.30630475189556,-1.,1.54159462645432));
#24022=CARTESIAN_POINT('Ctrl Pts',(-1.30630475189556,1.,1.54159462645432));
#24023=CARTESIAN_POINT('Ctrl Pts',(-1.30824393907473,-1.,1.54739413957185));
#24024=CARTESIAN_POINT('Ctrl Pts',(-1.30824393907473,1.,1.54739413957185));
#24025=CARTESIAN_POINT('Ctrl Pts',(-1.31014393684222,-1.,1.55322568759481));
#24026=CARTESIAN_POINT('Ctrl Pts',(-1.31014393684222,1.,1.55322568759481));
#24027=CARTESIAN_POINT('Ctrl Pts',(-1.31200264341696,-1.,1.55908521254821));
#24028=CARTESIAN_POINT('Ctrl Pts',(-1.31200264341696,1.,1.55908521254821));
#24029=CARTESIAN_POINT('Ctrl Pts',(-1.31381795281002,-1.,1.56496872402353));
#24030=CARTESIAN_POINT('Ctrl Pts',(-1.31381795281002,1.,1.56496872402353));
#24031=CARTESIAN_POINT('Ctrl Pts',(-1.31558903860016,-1.,1.57087397835723));
#24032=CARTESIAN_POINT('Ctrl Pts',(-1.31558903860016,1.,1.57087397835723));
#24033=CARTESIAN_POINT('Ctrl Pts',(-1.31731642317187,-1.,1.5768005650559));
#24034=CARTESIAN_POINT('Ctrl Pts',(-1.31731642317187,1.,1.5768005650559));
#24035=CARTESIAN_POINT('Ctrl Pts',(-1.31900135021432,-1.,1.58274907898834));
#24036=CARTESIAN_POINT('Ctrl Pts',(-1.31900135021432,1.,1.58274907898834));
#24037=CARTESIAN_POINT('Ctrl Pts',(-1.32064537110892,-1.,1.58872057258245));
#24038=CARTESIAN_POINT('Ctrl Pts',(-1.32064537110892,1.,1.58872057258245));
#24039=CARTESIAN_POINT('Ctrl Pts',(-1.32224985747682,-1.,1.59471591079403));
#24040=CARTESIAN_POINT('Ctrl Pts',(-1.32224985747682,1.,1.59471591079403));
#24041=CARTESIAN_POINT('Ctrl Pts',(-1.32381550858256,-1.,1.60073511858687));
#24042=CARTESIAN_POINT('Ctrl Pts',(-1.32381550858256,1.,1.60073511858687));
#24043=CARTESIAN_POINT('Ctrl Pts',(-1.32534250785782,-1.,1.60677758290954));
#24044=CARTESIAN_POINT('Ctrl Pts',(-1.32534250785782,1.,1.60677758290954));
#24045=CARTESIAN_POINT('Ctrl Pts',(-1.32683074483356,-1.,1.6128423401575));
#24046=CARTESIAN_POINT('Ctrl Pts',(-1.32683074483356,1.,1.6128423401575));
#24047=CARTESIAN_POINT('Ctrl Pts',(-1.32828000610449,-1.,1.61892832270724));
#24048=CARTESIAN_POINT('Ctrl Pts',(-1.32828000610449,1.,1.61892832270724));
#24049=CARTESIAN_POINT('Ctrl Pts',(-1.3296901950568,-1.,1.62503464209797));
#24050=CARTESIAN_POINT('Ctrl Pts',(-1.3296901950568,1.,1.62503464209797));
#24051=CARTESIAN_POINT('Ctrl Pts',(-1.33106149345645,-1.,1.63116079730923));
#24052=CARTESIAN_POINT('Ctrl Pts',(-1.33106149345645,1.,1.63116079730923));
#24053=CARTESIAN_POINT('Ctrl Pts',(-1.33239425103724,-1.,1.63730653475089));
#24054=CARTESIAN_POINT('Ctrl Pts',(-1.33239425103724,1.,1.63730653475089));
#24055=CARTESIAN_POINT('Ctrl Pts',(-1.33368890676572,-1.,1.6434717485603));
#24056=CARTESIAN_POINT('Ctrl Pts',(-1.33368890676572,1.,1.6434717485603));
#24057=CARTESIAN_POINT('Ctrl Pts',(-1.33494590467993,-1.,1.6496563728683));
#24058=CARTESIAN_POINT('Ctrl Pts',(-1.33494590467993,1.,1.6496563728683));
#24059=CARTESIAN_POINT('Ctrl Pts',(-1.33616559745172,-1.,1.65586025952593));
#24060=CARTESIAN_POINT('Ctrl Pts',(-1.33616559745172,1.,1.65586025952593));
#24061=CARTESIAN_POINT('Ctrl Pts',(-1.33734820885262,-1.,1.66208312541983));
#24062=CARTESIAN_POINT('Ctrl Pts',(-1.33734820885262,1.,1.66208312541983));
#24063=CARTESIAN_POINT('Ctrl Pts',(-1.33849388654388,-1.,1.66832460783989));
#24064=CARTESIAN_POINT('Ctrl Pts',(-1.33849388654388,1.,1.66832460783989));
#24065=CARTESIAN_POINT('Ctrl Pts',(-1.3396027347034,-1.,1.67458429426086));
#24066=CARTESIAN_POINT('Ctrl Pts',(-1.3396027347034,1.,1.67458429426086));
#24067=CARTESIAN_POINT('Ctrl Pts',(-1.34067485185203,-1.,1.68086176030362));
#24068=CARTESIAN_POINT('Ctrl Pts',(-1.34067485185203,1.,1.68086176030362));
#24069=CARTESIAN_POINT('Ctrl Pts',(-1.341710374848,-1.,1.68715660868764));
#24070=CARTESIAN_POINT('Ctrl Pts',(-1.341710374848,1.,1.68715660868764));
#24071=CARTESIAN_POINT('Ctrl Pts',(-1.34270948206319,-1.,1.6934684849687));
#24072=CARTESIAN_POINT('Ctrl Pts',(-1.34270948206319,1.,1.6934684849687));
#24073=CARTESIAN_POINT('Ctrl Pts',(-1.34367237124483,-1.,1.69979707754427));
#24074=CARTESIAN_POINT('Ctrl Pts',(-1.34367237124483,1.,1.69979707754427));
#24075=CARTESIAN_POINT('Ctrl Pts',(-1.34459924533831,-1.,1.70614212266738));
#24076=CARTESIAN_POINT('Ctrl Pts',(-1.34459924533831,1.,1.70614212266738));
#24077=CARTESIAN_POINT('Ctrl Pts',(-1.34549029589416,-1.,1.71250340686822));
#24078=CARTESIAN_POINT('Ctrl Pts',(-1.34549029589416,1.,1.71250340686822));
#24079=CARTESIAN_POINT('Ctrl Pts',(-1.34634568653227,-1.,1.7188807715049));
#24080=CARTESIAN_POINT('Ctrl Pts',(-1.34634568653227,1.,1.7188807715049));
#24081=CARTESIAN_POINT('Ctrl Pts',(-1.34716554819527,-1.,1.72527410680674));
#24082=CARTESIAN_POINT('Ctrl Pts',(-1.34716554819527,1.,1.72527410680674));
#24083=CARTESIAN_POINT('Ctrl Pts',(-1.34779309152035,-1.,1.7304014965394));
#24084=CARTESIAN_POINT('Ctrl Pts',(-1.34779309152035,1.,1.7304014965394));
#24085=CARTESIAN_POINT('Ctrl Pts',(-1.34824783112887,-1.,1.73425417885907));
#24086=CARTESIAN_POINT('Ctrl Pts',(-1.34824783112887,1.,1.73425417885907));
#24087=CARTESIAN_POINT('Ctrl Pts',(-1.34854391898045,-1.,1.73682580585691));
#24088=CARTESIAN_POINT('Ctrl Pts',(-1.34854391898045,1.,1.73682580585691));
#24089=CARTESIAN_POINT('Ctrl Pts',(-1.34869019493419,-1.,1.73811241238545));
#24090=CARTESIAN_POINT('Ctrl Pts',(-1.34869019493419,1.,1.73811241238545));
#24091=CARTESIAN_POINT('',(-1.15624053661742,1.,1.31362392696032));
#24092=CARTESIAN_POINT('Ctrl Pts',(-1.15624053661742,1.,1.31362392696032));
#24093=CARTESIAN_POINT('Ctrl Pts',(-1.15950888730809,1.,1.31722977216397));
#24094=CARTESIAN_POINT('Ctrl Pts',(-1.16589330093588,1.,1.32428080721772));
#24095=CARTESIAN_POINT('Ctrl Pts',(-1.17501305789857,1.,1.33437539347008));
#24096=CARTESIAN_POINT('Ctrl Pts',(-1.18625865667441,1.,1.34687054001093));
#24097=CARTESIAN_POINT('Ctrl Pts',(-1.1987959077932,1.,1.36088705043885));
#24098=CARTESIAN_POINT('Ctrl Pts',(-1.20982812925645,1.,1.37331915607905));
#24099=CARTESIAN_POINT('Ctrl Pts',(-1.21938737280852,1.,1.38420564527715));
#24100=CARTESIAN_POINT('Ctrl Pts',(-1.22752961899387,1.,1.39361389568796));
#24101=CARTESIAN_POINT('Ctrl Pts',(-1.23434087290423,1.,1.40164708206106));
#24102=CARTESIAN_POINT('Ctrl Pts',(-1.23994455029534,1.,1.40845295531283));
#24103=CARTESIAN_POINT('Ctrl Pts',(-1.24450600513056,1.,1.41422913175179));
#24104=CARTESIAN_POINT('Ctrl Pts',(-1.24824430986571,1.,1.41923722596025));
#24105=CARTESIAN_POINT('Ctrl Pts',(-1.2514145557001,1.,1.42378102115575));
#24106=CARTESIAN_POINT('Ctrl Pts',(-1.25426945222639,1.,1.42815938799387));
#24107=CARTESIAN_POINT('Ctrl Pts',(-1.25702687965755,1.,1.43262645609691));
#24108=CARTESIAN_POINT('Ctrl Pts',(-1.25983531012005,1.,1.43734919180848));
#24109=CARTESIAN_POINT('Ctrl Pts',(-1.26273903323859,1.,1.44236470511303));
#24110=CARTESIAN_POINT('Ctrl Pts',(-1.26570925118868,1.,1.44761985001662));
#24111=CARTESIAN_POINT('Ctrl Pts',(-1.2686778680489,1.,1.45301422764247));
#24112=CARTESIAN_POINT('Ctrl Pts',(-1.27156805265289,1.,1.45843906294697));
#24113=CARTESIAN_POINT('Ctrl Pts',(-1.27433119897822,1.,1.46382431332476));
#24114=CARTESIAN_POINT('Ctrl Pts',(-1.27696414831089,1.,1.46916035917133));
#24115=CARTESIAN_POINT('Ctrl Pts',(-1.2794891824849,1.,1.4744717526707));
#24116=CARTESIAN_POINT('Ctrl Pts',(-1.28194158939517,1.,1.47980070347095));
#24117=CARTESIAN_POINT('Ctrl Pts',(-1.28435533880201,1.,1.4851881711891));
#24118=CARTESIAN_POINT('Ctrl Pts',(-1.2867467611644,1.,1.4906522831278));
#24119=CARTESIAN_POINT('Ctrl Pts',(-1.28911506584254,1.,1.49618896881754));
#24120=CARTESIAN_POINT('Ctrl Pts',(-1.29145022885181,1.,1.50178230149776));
#24121=CARTESIAN_POINT('Ctrl Pts',(-1.29373841372842,1.,1.50741159078365));
#24122=CARTESIAN_POINT('Ctrl Pts',(-1.29596850710509,1.,1.51305994241402));
#24123=CARTESIAN_POINT('Ctrl Pts',(-1.29813791800747,1.,1.51872184912724));
#24124=CARTESIAN_POINT('Ctrl Pts',(-1.30024984366328,1.,1.52439957861062));
#24125=CARTESIAN_POINT('Ctrl Pts',(-1.30231064395568,1.,1.53009970283891));
#24126=CARTESIAN_POINT('Ctrl Pts',(-1.30432735639489,1.,1.53582981268977));
#24127=CARTESIAN_POINT('Ctrl Pts',(-1.30630475189556,1.,1.54159462645432));
#24128=CARTESIAN_POINT('Ctrl Pts',(-1.30824393907473,1.,1.54739413957185));
#24129=CARTESIAN_POINT('Ctrl Pts',(-1.31014393684222,1.,1.55322568759481));
#24130=CARTESIAN_POINT('Ctrl Pts',(-1.31200264341696,1.,1.55908521254821));
#24131=CARTESIAN_POINT('Ctrl Pts',(-1.31381795281002,1.,1.56496872402353));
#24132=CARTESIAN_POINT('Ctrl Pts',(-1.31558903860016,1.,1.57087397835723));
#24133=CARTESIAN_POINT('Ctrl Pts',(-1.31731642317187,1.,1.5768005650559));
#24134=CARTESIAN_POINT('Ctrl Pts',(-1.31900135021432,1.,1.58274907898834));
#24135=CARTESIAN_POINT('Ctrl Pts',(-1.32064537110892,1.,1.58872057258245));
#24136=CARTESIAN_POINT('Ctrl Pts',(-1.32224985747682,1.,1.59471591079403));
#24137=CARTESIAN_POINT('Ctrl Pts',(-1.32381550858256,1.,1.60073511858687));
#24138=CARTESIAN_POINT('Ctrl Pts',(-1.32534250785782,1.,1.60677758290954));
#24139=CARTESIAN_POINT('Ctrl Pts',(-1.32683074483356,1.,1.6128423401575));
#24140=CARTESIAN_POINT('Ctrl Pts',(-1.32828000610449,1.,1.61892832270724));
#24141=CARTESIAN_POINT('Ctrl Pts',(-1.3296901950568,1.,1.62503464209797));
#24142=CARTESIAN_POINT('Ctrl Pts',(-1.33106149345645,1.,1.63116079730923));
#24143=CARTESIAN_POINT('Ctrl Pts',(-1.33239425103724,1.,1.63730653475089));
#24144=CARTESIAN_POINT('Ctrl Pts',(-1.33368890676572,1.,1.6434717485603));
#24145=CARTESIAN_POINT('Ctrl Pts',(-1.33494590467993,1.,1.6496563728683));
#24146=CARTESIAN_POINT('Ctrl Pts',(-1.33616559745172,1.,1.65586025952593));
#24147=CARTESIAN_POINT('Ctrl Pts',(-1.33734820885262,1.,1.66208312541983));
#24148=CARTESIAN_POINT('Ctrl Pts',(-1.33849388654388,1.,1.66832460783989));
#24149=CARTESIAN_POINT('Ctrl Pts',(-1.3396027347034,1.,1.67458429426086));
#24150=CARTESIAN_POINT('Ctrl Pts',(-1.34067485185203,1.,1.68086176030362));
#24151=CARTESIAN_POINT('Ctrl Pts',(-1.341710374848,1.,1.68715660868764));
#24152=CARTESIAN_POINT('Ctrl Pts',(-1.34270948206319,1.,1.6934684849687));
#24153=CARTESIAN_POINT('Ctrl Pts',(-1.34367237124483,1.,1.69979707754427));
#24154=CARTESIAN_POINT('Ctrl Pts',(-1.34459924533831,1.,1.70614212266738));
#24155=CARTESIAN_POINT('Ctrl Pts',(-1.34549029589416,1.,1.71250340686822));
#24156=CARTESIAN_POINT('Ctrl Pts',(-1.34634568653227,1.,1.7188807715049));
#24157=CARTESIAN_POINT('Ctrl Pts',(-1.34716554819527,1.,1.72527410680674));
#24158=CARTESIAN_POINT('Ctrl Pts',(-1.34779309152035,1.,1.7304014965394));
#24159=CARTESIAN_POINT('Ctrl Pts',(-1.34824783112887,1.,1.73425417885907));
#24160=CARTESIAN_POINT('Ctrl Pts',(-1.34854391898045,1.,1.73682580585691));
#24161=CARTESIAN_POINT('Ctrl Pts',(-1.34869019493419,1.,1.73811241238545));
#24162=CARTESIAN_POINT('',(-1.15624053661742,0.,1.31362392696032));
#24163=CARTESIAN_POINT('Origin',(0.,0.,0.));
#24164=CARTESIAN_POINT('',(-1.31362392696033,1.,1.15624053661742));
#24165=CARTESIAN_POINT('Origin',(0.,1.,0.));
#24166=CARTESIAN_POINT('',(-1.31362392696033,0.,1.15624053661742));
#24167=CARTESIAN_POINT('Ctrl Pts',(-1.73811241238545,-1.,1.34869019493419));
#24168=CARTESIAN_POINT('Ctrl Pts',(-1.73811241238545,1.,1.34869019493419));
#24169=CARTESIAN_POINT('Ctrl Pts',(-1.73682580585819,-1.,1.34854391898145));
#24170=CARTESIAN_POINT('Ctrl Pts',(-1.73682580585819,1.,1.34854391898145));
#24171=CARTESIAN_POINT('Ctrl Pts',(-1.73425417886255,-1.,1.34824783113158));
#24172=CARTESIAN_POINT('Ctrl Pts',(-1.73425417886255,1.,1.34824783113158));
#24173=CARTESIAN_POINT('Ctrl Pts',(-1.73040149654497,-1.,1.3477930915247));
#24174=CARTESIAN_POINT('Ctrl Pts',(-1.73040149654497,1.,1.3477930915247));
#24175=CARTESIAN_POINT('Ctrl Pts',(-1.72527410681298,-1.,1.34716554820013));
#24176=CARTESIAN_POINT('Ctrl Pts',(-1.72527410681298,1.,1.34716554820013));
#24177=CARTESIAN_POINT('Ctrl Pts',(-1.7188807715095,-1.,1.34634568653586));
#24178=CARTESIAN_POINT('Ctrl Pts',(-1.7188807715095,1.,1.34634568653586));
#24179=CARTESIAN_POINT('Ctrl Pts',(-1.71250340687011,-1.,1.34549029589563));
#24180=CARTESIAN_POINT('Ctrl Pts',(-1.71250340687011,1.,1.34549029589563));
#24181=CARTESIAN_POINT('Ctrl Pts',(-1.70614212266676,-1.,1.34459924533783));
#24182=CARTESIAN_POINT('Ctrl Pts',(-1.70614212266676,1.,1.34459924533783));
#24183=CARTESIAN_POINT('Ctrl Pts',(-1.69979707754221,-1.,1.34367237124322));
#24184=CARTESIAN_POINT('Ctrl Pts',(-1.69979707754221,1.,1.34367237124322));
#24185=CARTESIAN_POINT('Ctrl Pts',(-1.6934684849664,-1.,1.34270948206139));
#24186=CARTESIAN_POINT('Ctrl Pts',(-1.6934684849664,1.,1.34270948206139));
#24187=CARTESIAN_POINT('Ctrl Pts',(-1.68715660868602,-1.,1.34171037484673));
#24188=CARTESIAN_POINT('Ctrl Pts',(-1.68715660868602,1.,1.34171037484673));
#24189=CARTESIAN_POINT('Ctrl Pts',(-1.68086176030308,-1.,1.3406748518516));
#24190=CARTESIAN_POINT('Ctrl Pts',(-1.68086176030308,1.,1.3406748518516));
#24191=CARTESIAN_POINT('Ctrl Pts',(-1.67458429426126,-1.,1.33960273470372));
#24192=CARTESIAN_POINT('Ctrl Pts',(-1.67458429426126,1.,1.33960273470372));
#24193=CARTESIAN_POINT('Ctrl Pts',(-1.66832460784078,-1.,1.33849388654458));
#24194=CARTESIAN_POINT('Ctrl Pts',(-1.66832460784078,1.,1.33849388654458));
#24195=CARTESIAN_POINT('Ctrl Pts',(-1.66208312542073,-1.,1.33734820885331));
#24196=CARTESIAN_POINT('Ctrl Pts',(-1.66208312542073,1.,1.33734820885331));
#24197=CARTESIAN_POINT('Ctrl Pts',(-1.65586025952651,-1.,1.33616559745217));
#24198=CARTESIAN_POINT('Ctrl Pts',(-1.65586025952651,1.,1.33616559745217));
#24199=CARTESIAN_POINT('Ctrl Pts',(-1.64965637286843,-1.,1.33494590468003));
#24200=CARTESIAN_POINT('Ctrl Pts',(-1.64965637286843,1.,1.33494590468003));
#24201=CARTESIAN_POINT('Ctrl Pts',(-1.64347174856007,-1.,1.33368890676554));
#24202=CARTESIAN_POINT('Ctrl Pts',(-1.64347174856007,1.,1.33368890676554));
#24203=CARTESIAN_POINT('Ctrl Pts',(-1.6373065347505,-1.,1.33239425103694));
#24204=CARTESIAN_POINT('Ctrl Pts',(-1.6373065347505,1.,1.33239425103694));
#24205=CARTESIAN_POINT('Ctrl Pts',(-1.63116079730887,-1.,1.33106149345618));
#24206=CARTESIAN_POINT('Ctrl Pts',(-1.63116079730887,1.,1.33106149345618));
#24207=CARTESIAN_POINT('Ctrl Pts',(-1.62503464209777,-1.,1.32969019505665));
#24208=CARTESIAN_POINT('Ctrl Pts',(-1.62503464209777,1.,1.32969019505665));
#24209=CARTESIAN_POINT('Ctrl Pts',(-1.61892832270723,-1.,1.32828000610448));
#24210=CARTESIAN_POINT('Ctrl Pts',(-1.61892832270723,1.,1.32828000610448));
#24211=CARTESIAN_POINT('Ctrl Pts',(-1.61284234015762,-1.,1.32683074483365));
#24212=CARTESIAN_POINT('Ctrl Pts',(-1.61284234015762,1.,1.32683074483365));
#24213=CARTESIAN_POINT('Ctrl Pts',(-1.6067775829097,-1.,1.32534250785794));
#24214=CARTESIAN_POINT('Ctrl Pts',(-1.6067775829097,1.,1.32534250785794));
#24215=CARTESIAN_POINT('Ctrl Pts',(-1.600735118587,-1.,1.32381550858266));
#24216=CARTESIAN_POINT('Ctrl Pts',(-1.600735118587,1.,1.32381550858266));
#24217=CARTESIAN_POINT('Ctrl Pts',(-1.59471591079408,-1.,1.32224985747686));
#24218=CARTESIAN_POINT('Ctrl Pts',(-1.59471591079408,1.,1.32224985747686));
#24219=CARTESIAN_POINT('Ctrl Pts',(-1.58872057258244,-1.,1.32064537110891));
#24220=CARTESIAN_POINT('Ctrl Pts',(-1.58872057258244,1.,1.32064537110891));
#24221=CARTESIAN_POINT('Ctrl Pts',(-1.58274907898829,-1.,1.31900135021428));
#24222=CARTESIAN_POINT('Ctrl Pts',(-1.58274907898829,1.,1.31900135021428));
#24223=CARTESIAN_POINT('Ctrl Pts',(-1.57680056505585,-1.,1.31731642317183));
#24224=CARTESIAN_POINT('Ctrl Pts',(-1.57680056505585,1.,1.31731642317183));
#24225=CARTESIAN_POINT('Ctrl Pts',(-1.57087397835721,-1.,1.31558903860015));
#24226=CARTESIAN_POINT('Ctrl Pts',(-1.57087397835721,1.,1.31558903860015));
#24227=CARTESIAN_POINT('Ctrl Pts',(-1.56496872402352,-1.,1.31381795281002));
#24228=CARTESIAN_POINT('Ctrl Pts',(-1.56496872402352,1.,1.31381795281002));
#24229=CARTESIAN_POINT('Ctrl Pts',(-1.55908521254822,-1.,1.31200264341696));
#24230=CARTESIAN_POINT('Ctrl Pts',(-1.55908521254822,1.,1.31200264341696));
#24231=CARTESIAN_POINT('Ctrl Pts',(-1.55322568759481,-1.,1.31014393684221));
#24232=CARTESIAN_POINT('Ctrl Pts',(-1.55322568759481,1.,1.31014393684221));
#24233=CARTESIAN_POINT('Ctrl Pts',(-1.54739413957183,-1.,1.30824393907471));
#24234=CARTESIAN_POINT('Ctrl Pts',(-1.54739413957183,1.,1.30824393907471));
#24235=CARTESIAN_POINT('Ctrl Pts',(-1.54159462645428,-1.,1.30630475189553));
#24236=CARTESIAN_POINT('Ctrl Pts',(-1.54159462645428,1.,1.30630475189553));
#24237=CARTESIAN_POINT('Ctrl Pts',(-1.53582981268976,-1.,1.30432735639487));
#24238=CARTESIAN_POINT('Ctrl Pts',(-1.53582981268976,1.,1.30432735639487));
#24239=CARTESIAN_POINT('Ctrl Pts',(-1.53009970283893,-1.,1.3023106439557));
#24240=CARTESIAN_POINT('Ctrl Pts',(-1.53009970283893,1.,1.3023106439557));
#24241=CARTESIAN_POINT('Ctrl Pts',(-1.5243995786107,-1.,1.30024984366334));
#24242=CARTESIAN_POINT('Ctrl Pts',(-1.5243995786107,1.,1.30024984366334));
#24243=CARTESIAN_POINT('Ctrl Pts',(-1.51872184912735,-1.,1.29813791800757));
#24244=CARTESIAN_POINT('Ctrl Pts',(-1.51872184912735,1.,1.29813791800757));
#24245=CARTESIAN_POINT('Ctrl Pts',(-1.51305994241412,-1.,1.29596850710518));
#24246=CARTESIAN_POINT('Ctrl Pts',(-1.51305994241412,1.,1.29596850710518));
#24247=CARTESIAN_POINT('Ctrl Pts',(-1.50741159078367,-1.,1.29373841372843));
#24248=CARTESIAN_POINT('Ctrl Pts',(-1.50741159078367,1.,1.29373841372843));
#24249=CARTESIAN_POINT('Ctrl Pts',(-1.50178230149764,-1.,1.29145022885171));
#24250=CARTESIAN_POINT('Ctrl Pts',(-1.50178230149764,1.,1.29145022885171));
#24251=CARTESIAN_POINT('Ctrl Pts',(-1.49618896881729,-1.,1.28911506584232));
#24252=CARTESIAN_POINT('Ctrl Pts',(-1.49618896881729,1.,1.28911506584232));
#24253=CARTESIAN_POINT('Ctrl Pts',(-1.4906522831275,-1.,1.28674676116415));
#24254=CARTESIAN_POINT('Ctrl Pts',(-1.4906522831275,1.,1.28674676116415));
#24255=CARTESIAN_POINT('Ctrl Pts',(-1.48518817118891,-1.,1.28435533880184));
#24256=CARTESIAN_POINT('Ctrl Pts',(-1.48518817118891,1.,1.28435533880184));
#24257=CARTESIAN_POINT('Ctrl Pts',(-1.47980070347102,-1.,1.28194158939522));
#24258=CARTESIAN_POINT('Ctrl Pts',(-1.47980070347102,1.,1.28194158939522));
#24259=CARTESIAN_POINT('Ctrl Pts',(-1.4744717526711,-1.,1.27948918248524));
#24260=CARTESIAN_POINT('Ctrl Pts',(-1.4744717526711,1.,1.27948918248524));
#24261=CARTESIAN_POINT('Ctrl Pts',(-1.46916035917197,-1.,1.27696414831144));
#24262=CARTESIAN_POINT('Ctrl Pts',(-1.46916035917197,1.,1.27696414831144));
#24263=CARTESIAN_POINT('Ctrl Pts',(-1.4638243133254,-1.,1.27433119897877));
#24264=CARTESIAN_POINT('Ctrl Pts',(-1.4638243133254,1.,1.27433119897877));
#24265=CARTESIAN_POINT('Ctrl Pts',(-1.45843906294725,-1.,1.27156805265312));
#24266=CARTESIAN_POINT('Ctrl Pts',(-1.45843906294725,1.,1.27156805265312));
#24267=CARTESIAN_POINT('Ctrl Pts',(-1.45301422764205,-1.,1.26867786804854));
#24268=CARTESIAN_POINT('Ctrl Pts',(-1.45301422764205,1.,1.26867786804854));
#24269=CARTESIAN_POINT('Ctrl Pts',(-1.44761985001544,-1.,1.26570925118767));
#24270=CARTESIAN_POINT('Ctrl Pts',(-1.44761985001544,1.,1.26570925118767));
#24271=CARTESIAN_POINT('Ctrl Pts',(-1.44236470511145,-1.,1.26273903323723));
#24272=CARTESIAN_POINT('Ctrl Pts',(-1.44236470511145,1.,1.26273903323723));
#24273=CARTESIAN_POINT('Ctrl Pts',(-1.43734919180719,-1.,1.25983531011894));
#24274=CARTESIAN_POINT('Ctrl Pts',(-1.43734919180719,1.,1.25983531011894));
#24275=CARTESIAN_POINT('Ctrl Pts',(-1.43262645609679,-1.,1.25702687965744));
#24276=CARTESIAN_POINT('Ctrl Pts',(-1.43262645609679,1.,1.25702687965744));
#24277=CARTESIAN_POINT('Ctrl Pts',(-1.42815938799555,-1.,1.25426945222783));
#24278=CARTESIAN_POINT('Ctrl Pts',(-1.42815938799555,1.,1.25426945222783));
#24279=CARTESIAN_POINT('Ctrl Pts',(-1.42378102115911,-1.,1.25141455570299));
#24280=CARTESIAN_POINT('Ctrl Pts',(-1.42378102115911,1.,1.25141455570299));
#24281=CARTESIAN_POINT('Ctrl Pts',(-1.41923722596421,-1.,1.24824430986911));
#24282=CARTESIAN_POINT('Ctrl Pts',(-1.41923722596421,1.,1.24824430986911));
#24283=CARTESIAN_POINT('Ctrl Pts',(-1.41422913175437,-1.,1.24450600513278));
#24284=CARTESIAN_POINT('Ctrl Pts',(-1.41422913175437,1.,1.24450600513278));
#24285=CARTESIAN_POINT('Ctrl Pts',(-1.40845295531151,-1.,1.23994455029421));
#24286=CARTESIAN_POINT('Ctrl Pts',(-1.40845295531151,1.,1.23994455029421));
#24287=CARTESIAN_POINT('Ctrl Pts',(-1.40164708205345,-1.,1.23434087289768));
#24288=CARTESIAN_POINT('Ctrl Pts',(-1.40164708205345,1.,1.23434087289768));
#24289=CARTESIAN_POINT('Ctrl Pts',(-1.39361389567257,-1.,1.22752961898063));
#24290=CARTESIAN_POINT('Ctrl Pts',(-1.39361389567257,1.,1.22752961898063));
#24291=CARTESIAN_POINT('Ctrl Pts',(-1.38420564525391,-1.,1.21938737278853));
#24292=CARTESIAN_POINT('Ctrl Pts',(-1.38420564525391,1.,1.21938737278853));
#24293=CARTESIAN_POINT('Ctrl Pts',(-1.37331915604962,-1.,1.20982812923113));
#24294=CARTESIAN_POINT('Ctrl Pts',(-1.37331915604962,1.,1.20982812923113));
#24295=CARTESIAN_POINT('Ctrl Pts',(-1.36088705040677,-1.,1.1987959077656));
#24296=CARTESIAN_POINT('Ctrl Pts',(-1.36088705040677,1.,1.1987959077656));
#24297=CARTESIAN_POINT('Ctrl Pts',(-1.34687053998157,-1.,1.18625865664915));
#24298=CARTESIAN_POINT('Ctrl Pts',(-1.34687053998157,1.,1.18625865664915));
#24299=CARTESIAN_POINT('Ctrl Pts',(-1.33437539344842,-1.,1.17501305787994));
#24300=CARTESIAN_POINT('Ctrl Pts',(-1.33437539344842,1.,1.17501305787994));
#24301=CARTESIAN_POINT('Ctrl Pts',(-1.32428080720544,-1.,1.16589330092532));
#24302=CARTESIAN_POINT('Ctrl Pts',(-1.32428080720544,1.,1.16589330092532));
#24303=CARTESIAN_POINT('Ctrl Pts',(-1.3172297721596,-1.,1.15950888730433));
#24304=CARTESIAN_POINT('Ctrl Pts',(-1.3172297721596,1.,1.15950888730433));
#24305=CARTESIAN_POINT('Ctrl Pts',(-1.31362392696033,-1.,1.15624053661742));
#24306=CARTESIAN_POINT('Ctrl Pts',(-1.31362392696033,1.,1.15624053661742));
#24307=CARTESIAN_POINT('',(-1.73811241238545,1.,1.34869019493419));
#24308=CARTESIAN_POINT('Ctrl Pts',(-1.73811241238545,1.,1.34869019493419));
#24309=CARTESIAN_POINT('Ctrl Pts',(-1.73682580585819,1.,1.34854391898145));
#24310=CARTESIAN_POINT('Ctrl Pts',(-1.73425417886255,1.,1.34824783113158));
#24311=CARTESIAN_POINT('Ctrl Pts',(-1.73040149654497,1.,1.3477930915247));
#24312=CARTESIAN_POINT('Ctrl Pts',(-1.72527410681298,1.,1.34716554820013));
#24313=CARTESIAN_POINT('Ctrl Pts',(-1.7188807715095,1.,1.34634568653586));
#24314=CARTESIAN_POINT('Ctrl Pts',(-1.71250340687011,1.,1.34549029589563));
#24315=CARTESIAN_POINT('Ctrl Pts',(-1.70614212266676,1.,1.34459924533783));
#24316=CARTESIAN_POINT('Ctrl Pts',(-1.69979707754221,1.,1.34367237124322));
#24317=CARTESIAN_POINT('Ctrl Pts',(-1.6934684849664,1.,1.34270948206139));
#24318=CARTESIAN_POINT('Ctrl Pts',(-1.68715660868602,1.,1.34171037484673));
#24319=CARTESIAN_POINT('Ctrl Pts',(-1.68086176030308,1.,1.3406748518516));
#24320=CARTESIAN_POINT('Ctrl Pts',(-1.67458429426126,1.,1.33960273470372));
#24321=CARTESIAN_POINT('Ctrl Pts',(-1.66832460784078,1.,1.33849388654458));
#24322=CARTESIAN_POINT('Ctrl Pts',(-1.66208312542073,1.,1.33734820885331));
#24323=CARTESIAN_POINT('Ctrl Pts',(-1.65586025952651,1.,1.33616559745217));
#24324=CARTESIAN_POINT('Ctrl Pts',(-1.64965637286843,1.,1.33494590468003));
#24325=CARTESIAN_POINT('Ctrl Pts',(-1.64347174856007,1.,1.33368890676554));
#24326=CARTESIAN_POINT('Ctrl Pts',(-1.6373065347505,1.,1.33239425103694));
#24327=CARTESIAN_POINT('Ctrl Pts',(-1.63116079730887,1.,1.33106149345618));
#24328=CARTESIAN_POINT('Ctrl Pts',(-1.62503464209777,1.,1.32969019505665));
#24329=CARTESIAN_POINT('Ctrl Pts',(-1.61892832270723,1.,1.32828000610448));
#24330=CARTESIAN_POINT('Ctrl Pts',(-1.61284234015762,1.,1.32683074483365));
#24331=CARTESIAN_POINT('Ctrl Pts',(-1.6067775829097,1.,1.32534250785794));
#24332=CARTESIAN_POINT('Ctrl Pts',(-1.600735118587,1.,1.32381550858266));
#24333=CARTESIAN_POINT('Ctrl Pts',(-1.59471591079408,1.,1.32224985747686));
#24334=CARTESIAN_POINT('Ctrl Pts',(-1.58872057258244,1.,1.32064537110891));
#24335=CARTESIAN_POINT('Ctrl Pts',(-1.58274907898829,1.,1.31900135021428));
#24336=CARTESIAN_POINT('Ctrl Pts',(-1.57680056505585,1.,1.31731642317183));
#24337=CARTESIAN_POINT('Ctrl Pts',(-1.57087397835721,1.,1.31558903860015));
#24338=CARTESIAN_POINT('Ctrl Pts',(-1.56496872402352,1.,1.31381795281002));
#24339=CARTESIAN_POINT('Ctrl Pts',(-1.55908521254822,1.,1.31200264341696));
#24340=CARTESIAN_POINT('Ctrl Pts',(-1.55322568759481,1.,1.31014393684221));
#24341=CARTESIAN_POINT('Ctrl Pts',(-1.54739413957183,1.,1.30824393907471));
#24342=CARTESIAN_POINT('Ctrl Pts',(-1.54159462645428,1.,1.30630475189553));
#24343=CARTESIAN_POINT('Ctrl Pts',(-1.53582981268976,1.,1.30432735639487));
#24344=CARTESIAN_POINT('Ctrl Pts',(-1.53009970283893,1.,1.3023106439557));
#24345=CARTESIAN_POINT('Ctrl Pts',(-1.5243995786107,1.,1.30024984366334));
#24346=CARTESIAN_POINT('Ctrl Pts',(-1.51872184912735,1.,1.29813791800757));
#24347=CARTESIAN_POINT('Ctrl Pts',(-1.51305994241412,1.,1.29596850710518));
#24348=CARTESIAN_POINT('Ctrl Pts',(-1.50741159078367,1.,1.29373841372843));
#24349=CARTESIAN_POINT('Ctrl Pts',(-1.50178230149764,1.,1.29145022885171));
#24350=CARTESIAN_POINT('Ctrl Pts',(-1.49618896881729,1.,1.28911506584232));
#24351=CARTESIAN_POINT('Ctrl Pts',(-1.4906522831275,1.,1.28674676116415));
#24352=CARTESIAN_POINT('Ctrl Pts',(-1.48518817118891,1.,1.28435533880184));
#24353=CARTESIAN_POINT('Ctrl Pts',(-1.47980070347102,1.,1.28194158939522));
#24354=CARTESIAN_POINT('Ctrl Pts',(-1.4744717526711,1.,1.27948918248524));
#24355=CARTESIAN_POINT('Ctrl Pts',(-1.46916035917197,1.,1.27696414831144));
#24356=CARTESIAN_POINT('Ctrl Pts',(-1.4638243133254,1.,1.27433119897877));
#24357=CARTESIAN_POINT('Ctrl Pts',(-1.45843906294725,1.,1.27156805265312));
#24358=CARTESIAN_POINT('Ctrl Pts',(-1.45301422764205,1.,1.26867786804854));
#24359=CARTESIAN_POINT('Ctrl Pts',(-1.44761985001544,1.,1.26570925118767));
#24360=CARTESIAN_POINT('Ctrl Pts',(-1.44236470511145,1.,1.26273903323723));
#24361=CARTESIAN_POINT('Ctrl Pts',(-1.43734919180719,1.,1.25983531011894));
#24362=CARTESIAN_POINT('Ctrl Pts',(-1.43262645609679,1.,1.25702687965744));
#24363=CARTESIAN_POINT('Ctrl Pts',(-1.42815938799555,1.,1.25426945222783));
#24364=CARTESIAN_POINT('Ctrl Pts',(-1.42378102115911,1.,1.25141455570299));
#24365=CARTESIAN_POINT('Ctrl Pts',(-1.41923722596421,1.,1.24824430986911));
#24366=CARTESIAN_POINT('Ctrl Pts',(-1.41422913175437,1.,1.24450600513278));
#24367=CARTESIAN_POINT('Ctrl Pts',(-1.40845295531151,1.,1.23994455029421));
#24368=CARTESIAN_POINT('Ctrl Pts',(-1.40164708205345,1.,1.23434087289768));
#24369=CARTESIAN_POINT('Ctrl Pts',(-1.39361389567257,1.,1.22752961898063));
#24370=CARTESIAN_POINT('Ctrl Pts',(-1.38420564525391,1.,1.21938737278853));
#24371=CARTESIAN_POINT('Ctrl Pts',(-1.37331915604962,1.,1.20982812923113));
#24372=CARTESIAN_POINT('Ctrl Pts',(-1.36088705040677,1.,1.1987959077656));
#24373=CARTESIAN_POINT('Ctrl Pts',(-1.34687053998157,1.,1.18625865664915));
#24374=CARTESIAN_POINT('Ctrl Pts',(-1.33437539344842,1.,1.17501305787994));
#24375=CARTESIAN_POINT('Ctrl Pts',(-1.32428080720544,1.,1.16589330092532));
#24376=CARTESIAN_POINT('Ctrl Pts',(-1.3172297721596,1.,1.15950888730433));
#24377=CARTESIAN_POINT('Ctrl Pts',(-1.31362392696033,1.,1.15624053661742));
#24378=CARTESIAN_POINT('',(-1.73811241238545,0.,1.34869019493419));
#24379=CARTESIAN_POINT('Origin',(-1.81978687191668,0.,1.23627494547115));
#24380=CARTESIAN_POINT('',(-1.81978687191668,1.,1.23627494547115));
#24381=CARTESIAN_POINT('',(-1.73811241238545,1.,1.34869019493419));
#24382=CARTESIAN_POINT('',(-1.81978687191668,0.,1.23627494547115));
#24383=CARTESIAN_POINT('Ctrl Pts',(-1.5055822144029,-1.,0.892032620296855));
#24384=CARTESIAN_POINT('Ctrl Pts',(-1.5055822144029,1.,0.892032620296855));
#24385=CARTESIAN_POINT('Ctrl Pts',(-1.50980486807181,-1.,0.894452006967538));
#24386=CARTESIAN_POINT('Ctrl Pts',(-1.50980486807181,1.,0.894452006967538));
#24387=CARTESIAN_POINT('Ctrl Pts',(-1.51805569591479,-1.,0.89918504749193));
#24388=CARTESIAN_POINT('Ctrl Pts',(-1.51805569591479,1.,0.89918504749193));
#24389=CARTESIAN_POINT('Ctrl Pts',(-1.52984849890434,-1.,0.905967409640499));
#24390=CARTESIAN_POINT('Ctrl Pts',(-1.52984849890434,1.,0.905967409640499));
#24391=CARTESIAN_POINT('Ctrl Pts',(-1.54440491152808,-1.,0.91437591904658));
#24392=CARTESIAN_POINT('Ctrl Pts',(-1.54440491152808,1.,0.91437591904658));
#24393=CARTESIAN_POINT('Ctrl Pts',(-1.56065988582509,-1.,0.923832188966322));
#24394=CARTESIAN_POINT('Ctrl Pts',(-1.56065988582509,1.,0.923832188966322));
#24395=CARTESIAN_POINT('Ctrl Pts',(-1.57499388385561,-1.,0.932246680128849));
#24396=CARTESIAN_POINT('Ctrl Pts',(-1.57499388385561,1.,0.932246680128849));
#24397=CARTESIAN_POINT('Ctrl Pts',(-1.58744937489796,-1.,0.939646377909319));
#24398=CARTESIAN_POINT('Ctrl Pts',(-1.58744937489796,1.,0.939646377909319));
#24399=CARTESIAN_POINT('Ctrl Pts',(-1.59810042045408,-1.,0.946078063325796));
#24400=CARTESIAN_POINT('Ctrl Pts',(-1.59810042045408,1.,0.946078063325796));
#24401=CARTESIAN_POINT('Ctrl Pts',(-1.60706069897794,-1.,0.951613284361248));
#24402=CARTESIAN_POINT('Ctrl Pts',(-1.60706069897794,1.,0.951613284361248));
#24403=CARTESIAN_POINT('Ctrl Pts',(-1.61449324337233,-1.,0.956354422921573));
#24404=CARTESIAN_POINT('Ctrl Pts',(-1.61449324337233,1.,0.956354422921573));
#24405=CARTESIAN_POINT('Ctrl Pts',(-1.62061638139929,-1.,0.960438326099958));
#24406=CARTESIAN_POINT('Ctrl Pts',(-1.62061638139929,1.,0.960438326099958));
#24407=CARTESIAN_POINT('Ctrl Pts',(-1.6257193066974,-1.,0.964046107037821));
#24408=CARTESIAN_POINT('Ctrl Pts',(-1.6257193066974,1.,0.964046107037821));
#24409=CARTESIAN_POINT('Ctrl Pts',(-1.63013849959083,-1.,0.967387853228041));
#24410=CARTESIAN_POINT('Ctrl Pts',(-1.63013849959083,1.,0.967387853228041));
#24411=CARTESIAN_POINT('Ctrl Pts',(-1.63420665729609,-1.,0.970669715996356));
#24412=CARTESIAN_POINT('Ctrl Pts',(-1.63420665729609,1.,0.970669715996356));
#24413=CARTESIAN_POINT('Ctrl Pts',(-1.63820952658157,-1.,0.974066058287501));
#24414=CARTESIAN_POINT('Ctrl Pts',(-1.63820952658157,1.,0.974066058287501));
#24415=CARTESIAN_POINT('Ctrl Pts',(-1.64233990826831,-1.,0.977689794120297));
#24416=CARTESIAN_POINT('Ctrl Pts',(-1.64233990826831,1.,0.977689794120297));
#24417=CARTESIAN_POINT('Ctrl Pts',(-1.64665139190834,-1.,0.981562530940574));
#24418=CARTESIAN_POINT('Ctrl Pts',(-1.64665139190834,1.,0.981562530940574));
#24419=CARTESIAN_POINT('Ctrl Pts',(-1.6511001661277,-1.,0.985642622921626));
#24420=CARTESIAN_POINT('Ctrl Pts',(-1.6511001661277,1.,0.985642622921626));
#24421=CARTESIAN_POINT('Ctrl Pts',(-1.65559044289746,-1.,0.98985562785445));
#24422=CARTESIAN_POINT('Ctrl Pts',(-1.65559044289746,1.,0.98985562785445));
#24423=CARTESIAN_POINT('Ctrl Pts',(-1.66001553809916,-1.,0.994121836661116));
#24424=CARTESIAN_POINT('Ctrl Pts',(-1.66001553809916,1.,0.994121836661116));
#24425=CARTESIAN_POINT('Ctrl Pts',(-1.66430758030304,-1.,0.998389654952317));
#24426=CARTESIAN_POINT('Ctrl Pts',(-1.66430758030304,1.,0.998389654952317));
#24427=CARTESIAN_POINT('Ctrl Pts',(-1.66846059277231,-1.,1.00265091003682));
#24428=CARTESIAN_POINT('Ctrl Pts',(-1.66846059277231,1.,1.00265091003682));
#24429=CARTESIAN_POINT('Ctrl Pts',(-1.67250335383248,-1.,1.00692206696387));
#24430=CARTESIAN_POINT('Ctrl Pts',(-1.67250335383248,1.,1.00692206696387));
#24431=CARTESIAN_POINT('Ctrl Pts',(-1.67648246776457,-1.,1.01123236493507));
#24432=CARTESIAN_POINT('Ctrl Pts',(-1.67648246776457,1.,1.01123236493507));
#24433=CARTESIAN_POINT('Ctrl Pts',(-1.6804428989482,-1.,1.01561026162787));
#24434=CARTESIAN_POINT('Ctrl Pts',(-1.6804428989482,1.,1.01561026162787));
#24435=CARTESIAN_POINT('Ctrl Pts',(-1.68440578021739,-1.,1.02006795074222));
#24436=CARTESIAN_POINT('Ctrl Pts',(-1.68440578021739,1.,1.02006795074222));
#24437=CARTESIAN_POINT('Ctrl Pts',(-1.68836910178475,-1.,1.02460180535272));
#24438=CARTESIAN_POINT('Ctrl Pts',(-1.68836910178475,1.,1.02460180535272));
#24439=CARTESIAN_POINT('Ctrl Pts',(-1.69231840863471,-1.,1.02919977579155));
#24440=CARTESIAN_POINT('Ctrl Pts',(-1.69231840863471,1.,1.02919977579155));
#24441=CARTESIAN_POINT('Ctrl Pts',(-1.69623414782769,-1.,1.03384646003587));
#24442=CARTESIAN_POINT('Ctrl Pts',(-1.69623414782769,1.,1.03384646003587));
#24443=CARTESIAN_POINT('Ctrl Pts',(-1.70010052930951,-1.,1.03852922490782));
#24444=CARTESIAN_POINT('Ctrl Pts',(-1.70010052930951,1.,1.03852922490782));
#24445=CARTESIAN_POINT('Ctrl Pts',(-1.70391338707969,-1.,1.04324363334546));
#24446=CARTESIAN_POINT('Ctrl Pts',(-1.70391338707969,1.,1.04324363334546));
#24447=CARTESIAN_POINT('Ctrl Pts',(-1.70767646263641,-1.,1.0479908540499));
#24448=CARTESIAN_POINT('Ctrl Pts',(-1.70767646263641,1.,1.0479908540499));
#24449=CARTESIAN_POINT('Ctrl Pts',(-1.71139783543986,-1.,1.05277517202854));
#24450=CARTESIAN_POINT('Ctrl Pts',(-1.71139783543986,1.,1.05277517202854));
#24451=CARTESIAN_POINT('Ctrl Pts',(-1.71508654427022,-1.,1.05760163192481));
#24452=CARTESIAN_POINT('Ctrl Pts',(-1.71508654427022,1.,1.05760163192481));
#24453=CARTESIAN_POINT('Ctrl Pts',(-1.71874858456908,-1.,1.0624732468065));
#24454=CARTESIAN_POINT('Ctrl Pts',(-1.71874858456908,1.,1.0624732468065));
#24455=CARTESIAN_POINT('Ctrl Pts',(-1.72238500928456,-1.,1.06738966975463));
#24456=CARTESIAN_POINT('Ctrl Pts',(-1.72238500928456,1.,1.06738966975463));
#24457=CARTESIAN_POINT('Ctrl Pts',(-1.72599406198489,-1.,1.07234866990252));
#24458=CARTESIAN_POINT('Ctrl Pts',(-1.72599406198489,1.,1.07234866990252));
#24459=CARTESIAN_POINT('Ctrl Pts',(-1.72957248977424,-1.,1.0773470373727));
#24460=CARTESIAN_POINT('Ctrl Pts',(-1.72957248977424,1.,1.0773470373727));
#24461=CARTESIAN_POINT('Ctrl Pts',(-1.73311705663407,-1.,1.08238162784749));
#24462=CARTESIAN_POINT('Ctrl Pts',(-1.73311705663407,1.,1.08238162784749));
#24463=CARTESIAN_POINT('Ctrl Pts',(-1.73662628326093,-1.,1.08745056285429));
#24464=CARTESIAN_POINT('Ctrl Pts',(-1.73662628326093,1.,1.08745056285429));
#24465=CARTESIAN_POINT('Ctrl Pts',(-1.74010053962252,-1.,1.09255329056496));
#24466=CARTESIAN_POINT('Ctrl Pts',(-1.74010053962252,1.,1.09255329056496));
#24467=CARTESIAN_POINT('Ctrl Pts',(-1.74354119236212,-1.,1.09768999241229));
#24468=CARTESIAN_POINT('Ctrl Pts',(-1.74354119236212,1.,1.09768999241229));
#24469=CARTESIAN_POINT('Ctrl Pts',(-1.74695004214924,-1.,1.10286118991144));
#24470=CARTESIAN_POINT('Ctrl Pts',(-1.74695004214924,1.,1.10286118991144));
#24471=CARTESIAN_POINT('Ctrl Pts',(-1.75032866075914,-1.,1.10806728183003));
#24472=CARTESIAN_POINT('Ctrl Pts',(-1.75032866075914,1.,1.10806728183003));
#24473=CARTESIAN_POINT('Ctrl Pts',(-1.75367772094617,-1.,1.11330807582542));
#24474=CARTESIAN_POINT('Ctrl Pts',(-1.75367772094617,1.,1.11330807582542));
#24475=CARTESIAN_POINT('Ctrl Pts',(-1.75699720772089,-1.,1.11858293216752));
#24476=CARTESIAN_POINT('Ctrl Pts',(-1.75699720772089,1.,1.11858293216752));
#24477=CARTESIAN_POINT('Ctrl Pts',(-1.76028671825084,-1.,1.12389096855078));
#24478=CARTESIAN_POINT('Ctrl Pts',(-1.76028671825084,1.,1.12389096855078));
#24479=CARTESIAN_POINT('Ctrl Pts',(-1.76354571966171,-1.,1.12923123555076));
#24480=CARTESIAN_POINT('Ctrl Pts',(-1.76354571966171,1.,1.12923123555076));
#24481=CARTESIAN_POINT('Ctrl Pts',(-1.76677384551883,-1.,1.13460291804635));
#24482=CARTESIAN_POINT('Ctrl Pts',(-1.76677384551883,1.,1.13460291804635));
#24483=CARTESIAN_POINT('Ctrl Pts',(-1.76997111386806,-1.,1.14000548337));
#24484=CARTESIAN_POINT('Ctrl Pts',(-1.76997111386806,1.,1.14000548337));
#24485=CARTESIAN_POINT('Ctrl Pts',(-1.77313777896234,-1.,1.14543858226948));
#24486=CARTESIAN_POINT('Ctrl Pts',(-1.77313777896234,1.,1.14543858226948));
#24487=CARTESIAN_POINT('Ctrl Pts',(-1.77627422557034,-1.,1.15090197841531));
#24488=CARTESIAN_POINT('Ctrl Pts',(-1.77627422557034,1.,1.15090197841531));
#24489=CARTESIAN_POINT('Ctrl Pts',(-1.77938085564261,-1.,1.15639547194689));
#24490=CARTESIAN_POINT('Ctrl Pts',(-1.77938085564261,1.,1.15639547194689));
#24491=CARTESIAN_POINT('Ctrl Pts',(-1.78245795880949,-1.,1.16191881298458));
#24492=CARTESIAN_POINT('Ctrl Pts',(-1.78245795880949,1.,1.16191881298458));
#24493=CARTESIAN_POINT('Ctrl Pts',(-1.78550566040349,-1.,1.16747166312239));
#24494=CARTESIAN_POINT('Ctrl Pts',(-1.78550566040349,1.,1.16747166312239));
#24495=CARTESIAN_POINT('Ctrl Pts',(-1.78852398877523,-1.,1.17305363177265));
#24496=CARTESIAN_POINT('Ctrl Pts',(-1.78852398877523,1.,1.17305363177265));
#24497=CARTESIAN_POINT('Ctrl Pts',(-1.79151291552646,-1.,1.17866429440781));
#24498=CARTESIAN_POINT('Ctrl Pts',(-1.79151291552646,1.,1.17866429440781));
#24499=CARTESIAN_POINT('Ctrl Pts',(-1.79447240321572,-1.,1.18430321697471));
#24500=CARTESIAN_POINT('Ctrl Pts',(-1.79447240321572,1.,1.18430321697471));
#24501=CARTESIAN_POINT('Ctrl Pts',(-1.79740245923649,-1.,1.1899699793456));
#24502=CARTESIAN_POINT('Ctrl Pts',(-1.79740245923649,1.,1.1899699793456));
#24503=CARTESIAN_POINT('Ctrl Pts',(-1.80030314370121,-1.,1.19566418930405));
#24504=CARTESIAN_POINT('Ctrl Pts',(-1.80030314370121,1.,1.19566418930405));
#24505=CARTESIAN_POINT('Ctrl Pts',(-1.8031745483882,-1.,1.2013854893912));
#24506=CARTESIAN_POINT('Ctrl Pts',(-1.8031745483882,1.,1.2013854893912));
#24507=CARTESIAN_POINT('Ctrl Pts',(-1.80601678480772,-1.,1.20713356605519));
#24508=CARTESIAN_POINT('Ctrl Pts',(-1.80601678480772,1.,1.20713356605519));
#24509=CARTESIAN_POINT('Ctrl Pts',(-1.80882996916931,-1.,1.2129081570818));
#24510=CARTESIAN_POINT('Ctrl Pts',(-1.80882996916931,1.,1.2129081570818));
#24511=CARTESIAN_POINT('Ctrl Pts',(-1.81161420806172,-1.,1.2187090610323));
#24512=CARTESIAN_POINT('Ctrl Pts',(-1.81161420806172,1.,1.2187090610323));
#24513=CARTESIAN_POINT('Ctrl Pts',(-1.81436959209778,-1.,1.22453613304507));
#24514=CARTESIAN_POINT('Ctrl Pts',(-1.81436959209778,1.,1.22453613304507));
#24515=CARTESIAN_POINT('Ctrl Pts',(-1.81655087183054,-1.,1.22921864890975));
#24516=CARTESIAN_POINT('Ctrl Pts',(-1.81655087183054,1.,1.22921864890975));
#24517=CARTESIAN_POINT('Ctrl Pts',(-1.81817389920914,-1.,1.23274224526804));
#24518=CARTESIAN_POINT('Ctrl Pts',(-1.81817389920914,1.,1.23274224526804));
#24519=CARTESIAN_POINT('Ctrl Pts',(-1.81925017193531,-1.,1.23509651170384));
#24520=CARTESIAN_POINT('Ctrl Pts',(-1.81925017193531,1.,1.23509651170384));
#24521=CARTESIAN_POINT('Ctrl Pts',(-1.81978687191668,-1.,1.23627494547115));
#24522=CARTESIAN_POINT('Ctrl Pts',(-1.81978687191668,1.,1.23627494547115));
#24523=CARTESIAN_POINT('',(-1.5055822144029,1.,0.892032620296855));
#24524=CARTESIAN_POINT('Ctrl Pts',(-1.5055822144029,1.,0.892032620296855));
#24525=CARTESIAN_POINT('Ctrl Pts',(-1.50980486807181,1.,0.894452006967538));
#24526=CARTESIAN_POINT('Ctrl Pts',(-1.51805569591479,1.,0.89918504749193));
#24527=CARTESIAN_POINT('Ctrl Pts',(-1.52984849890434,1.,0.905967409640499));
#24528=CARTESIAN_POINT('Ctrl Pts',(-1.54440491152808,1.,0.91437591904658));
#24529=CARTESIAN_POINT('Ctrl Pts',(-1.56065988582509,1.,0.923832188966322));
#24530=CARTESIAN_POINT('Ctrl Pts',(-1.57499388385561,1.,0.932246680128849));
#24531=CARTESIAN_POINT('Ctrl Pts',(-1.58744937489796,1.,0.939646377909319));
#24532=CARTESIAN_POINT('Ctrl Pts',(-1.59810042045408,1.,0.946078063325796));
#24533=CARTESIAN_POINT('Ctrl Pts',(-1.60706069897794,1.,0.951613284361248));
#24534=CARTESIAN_POINT('Ctrl Pts',(-1.61449324337233,1.,0.956354422921573));
#24535=CARTESIAN_POINT('Ctrl Pts',(-1.62061638139929,1.,0.960438326099958));
#24536=CARTESIAN_POINT('Ctrl Pts',(-1.6257193066974,1.,0.964046107037821));
#24537=CARTESIAN_POINT('Ctrl Pts',(-1.63013849959083,1.,0.967387853228041));
#24538=CARTESIAN_POINT('Ctrl Pts',(-1.63420665729609,1.,0.970669715996356));
#24539=CARTESIAN_POINT('Ctrl Pts',(-1.63820952658157,1.,0.974066058287501));
#24540=CARTESIAN_POINT('Ctrl Pts',(-1.64233990826831,1.,0.977689794120297));
#24541=CARTESIAN_POINT('Ctrl Pts',(-1.64665139190834,1.,0.981562530940574));
#24542=CARTESIAN_POINT('Ctrl Pts',(-1.6511001661277,1.,0.985642622921626));
#24543=CARTESIAN_POINT('Ctrl Pts',(-1.65559044289746,1.,0.98985562785445));
#24544=CARTESIAN_POINT('Ctrl Pts',(-1.66001553809916,1.,0.994121836661116));
#24545=CARTESIAN_POINT('Ctrl Pts',(-1.66430758030304,1.,0.998389654952317));
#24546=CARTESIAN_POINT('Ctrl Pts',(-1.66846059277231,1.,1.00265091003682));
#24547=CARTESIAN_POINT('Ctrl Pts',(-1.67250335383248,1.,1.00692206696387));
#24548=CARTESIAN_POINT('Ctrl Pts',(-1.67648246776457,1.,1.01123236493507));
#24549=CARTESIAN_POINT('Ctrl Pts',(-1.6804428989482,1.,1.01561026162787));
#24550=CARTESIAN_POINT('Ctrl Pts',(-1.68440578021739,1.,1.02006795074222));
#24551=CARTESIAN_POINT('Ctrl Pts',(-1.68836910178475,1.,1.02460180535272));
#24552=CARTESIAN_POINT('Ctrl Pts',(-1.69231840863471,1.,1.02919977579155));
#24553=CARTESIAN_POINT('Ctrl Pts',(-1.69623414782769,1.,1.03384646003587));
#24554=CARTESIAN_POINT('Ctrl Pts',(-1.70010052930951,1.,1.03852922490782));
#24555=CARTESIAN_POINT('Ctrl Pts',(-1.70391338707969,1.,1.04324363334546));
#24556=CARTESIAN_POINT('Ctrl Pts',(-1.70767646263641,1.,1.0479908540499));
#24557=CARTESIAN_POINT('Ctrl Pts',(-1.71139783543986,1.,1.05277517202854));
#24558=CARTESIAN_POINT('Ctrl Pts',(-1.71508654427022,1.,1.05760163192481));
#24559=CARTESIAN_POINT('Ctrl Pts',(-1.71874858456908,1.,1.0624732468065));
#24560=CARTESIAN_POINT('Ctrl Pts',(-1.72238500928456,1.,1.06738966975463));
#24561=CARTESIAN_POINT('Ctrl Pts',(-1.72599406198489,1.,1.07234866990252));
#24562=CARTESIAN_POINT('Ctrl Pts',(-1.72957248977424,1.,1.0773470373727));
#24563=CARTESIAN_POINT('Ctrl Pts',(-1.73311705663407,1.,1.08238162784749));
#24564=CARTESIAN_POINT('Ctrl Pts',(-1.73662628326093,1.,1.08745056285429));
#24565=CARTESIAN_POINT('Ctrl Pts',(-1.74010053962252,1.,1.09255329056496));
#24566=CARTESIAN_POINT('Ctrl Pts',(-1.74354119236212,1.,1.09768999241229));
#24567=CARTESIAN_POINT('Ctrl Pts',(-1.74695004214924,1.,1.10286118991144));
#24568=CARTESIAN_POINT('Ctrl Pts',(-1.75032866075914,1.,1.10806728183003));
#24569=CARTESIAN_POINT('Ctrl Pts',(-1.75367772094617,1.,1.11330807582542));
#24570=CARTESIAN_POINT('Ctrl Pts',(-1.75699720772089,1.,1.11858293216752));
#24571=CARTESIAN_POINT('Ctrl Pts',(-1.76028671825084,1.,1.12389096855078));
#24572=CARTESIAN_POINT('Ctrl Pts',(-1.76354571966171,1.,1.12923123555076));
#24573=CARTESIAN_POINT('Ctrl Pts',(-1.76677384551883,1.,1.13460291804635));
#24574=CARTESIAN_POINT('Ctrl Pts',(-1.76997111386806,1.,1.14000548337));
#24575=CARTESIAN_POINT('Ctrl Pts',(-1.77313777896234,1.,1.14543858226948));
#24576=CARTESIAN_POINT('Ctrl Pts',(-1.77627422557034,1.,1.15090197841531));
#24577=CARTESIAN_POINT('Ctrl Pts',(-1.77938085564261,1.,1.15639547194689));
#24578=CARTESIAN_POINT('Ctrl Pts',(-1.78245795880949,1.,1.16191881298458));
#24579=CARTESIAN_POINT('Ctrl Pts',(-1.78550566040349,1.,1.16747166312239));
#24580=CARTESIAN_POINT('Ctrl Pts',(-1.78852398877523,1.,1.17305363177265));
#24581=CARTESIAN_POINT('Ctrl Pts',(-1.79151291552646,1.,1.17866429440781));
#24582=CARTESIAN_POINT('Ctrl Pts',(-1.79447240321572,1.,1.18430321697471));
#24583=CARTESIAN_POINT('Ctrl Pts',(-1.79740245923649,1.,1.1899699793456));
#24584=CARTESIAN_POINT('Ctrl Pts',(-1.80030314370121,1.,1.19566418930405));
#24585=CARTESIAN_POINT('Ctrl Pts',(-1.8031745483882,1.,1.2013854893912));
#24586=CARTESIAN_POINT('Ctrl Pts',(-1.80601678480772,1.,1.20713356605519));
#24587=CARTESIAN_POINT('Ctrl Pts',(-1.80882996916931,1.,1.2129081570818));
#24588=CARTESIAN_POINT('Ctrl Pts',(-1.81161420806172,1.,1.2187090610323));
#24589=CARTESIAN_POINT('Ctrl Pts',(-1.81436959209778,1.,1.22453613304507));
#24590=CARTESIAN_POINT('Ctrl Pts',(-1.81655087183054,1.,1.22921864890975));
#24591=CARTESIAN_POINT('Ctrl Pts',(-1.81817389920914,1.,1.23274224526804));
#24592=CARTESIAN_POINT('Ctrl Pts',(-1.81925017193531,1.,1.23509651170384));
#24593=CARTESIAN_POINT('Ctrl Pts',(-1.81978687191668,1.,1.23627494547115));
#24594=CARTESIAN_POINT('',(-1.5055822144029,0.,0.892032620296856));
#24595=CARTESIAN_POINT('Origin',(0.,0.,0.));
#24596=CARTESIAN_POINT('',(-1.60662857109684,1.,0.693717979106305));
#24597=CARTESIAN_POINT('Origin',(0.,1.,0.));
#24598=CARTESIAN_POINT('',(-1.60662857109684,0.,0.693717979106306));
#24599=CARTESIAN_POINT('Ctrl Pts',(-2.0698113262342,-1.,0.7455743247944));
#24600=CARTESIAN_POINT('Ctrl Pts',(-2.0698113262342,1.,0.7455743247944));
#24601=CARTESIAN_POINT('Ctrl Pts',(-2.06854248895728,-1.,0.745832791378367));
#24602=CARTESIAN_POINT('Ctrl Pts',(-2.06854248895728,1.,0.745832791378367));
#24603=CARTESIAN_POINT('Ctrl Pts',(-2.06600523016815,-1.,0.7463458715442));
#24604=CARTESIAN_POINT('Ctrl Pts',(-2.06600523016815,1.,0.7463458715442));
#24605=CARTESIAN_POINT('Ctrl Pts',(-2.06220058927826,-1.,0.747103932787919));
#24606=CARTESIAN_POINT('Ctrl Pts',(-2.06220058927826,1.,0.747103932787919));
#24607=CARTESIAN_POINT('Ctrl Pts',(-2.05713023031006,-1.,0.748091554183802));
#24608=CARTESIAN_POINT('Ctrl Pts',(-2.05713023031006,1.,0.748091554183802));
#24609=CARTESIAN_POINT('Ctrl Pts',(-2.05079645592154,-1.,0.749287468665046));
#24610=CARTESIAN_POINT('Ctrl Pts',(-2.05079645592154,1.,0.749287468665046));
#24611=CARTESIAN_POINT('Ctrl Pts',(-2.04446689147979,-1.,0.750444657875576));
#24612=CARTESIAN_POINT('Ctrl Pts',(-2.04446689147979,1.,0.750444657875576));
#24613=CARTESIAN_POINT('Ctrl Pts',(-2.03814160092099,-1.,0.751562963361115));
#24614=CARTESIAN_POINT('Ctrl Pts',(-2.03814160092099,1.,0.751562963361115));
#24615=CARTESIAN_POINT('Ctrl Pts',(-2.03182068456221,-1.,0.752642180487211));
#24616=CARTESIAN_POINT('Ctrl Pts',(-2.03182068456221,1.,0.752642180487211));
#24617=CARTESIAN_POINT('Ctrl Pts',(-2.02550428623313,-1.,0.753682061112768));
#24618=CARTESIAN_POINT('Ctrl Pts',(-2.02550428623313,1.,0.753682061112768));
#24619=CARTESIAN_POINT('Ctrl Pts',(-2.01919259405809,-1.,0.754682330722816));
#24620=CARTESIAN_POINT('Ctrl Pts',(-2.01919259405809,1.,0.754682330722816));
#24621=CARTESIAN_POINT('Ctrl Pts',(-2.01288584328084,-1.,0.755642704957865));
#24622=CARTESIAN_POINT('Ctrl Pts',(-2.01288584328084,1.,0.755642704957865));
#24623=CARTESIAN_POINT('Ctrl Pts',(-2.0065843158773,-1.,0.75656290464667));
#24624=CARTESIAN_POINT('Ctrl Pts',(-2.0065843158773,1.,0.75656290464667));
#24625=CARTESIAN_POINT('Ctrl Pts',(-2.00028834739178,-1.,0.757442676862724));
#24626=CARTESIAN_POINT('Ctrl Pts',(-2.00028834739178,1.,0.757442676862724));
#24627=CARTESIAN_POINT('Ctrl Pts',(-1.99399831098817,-1.,0.758281796766761));
#24628=CARTESIAN_POINT('Ctrl Pts',(-1.99399831098817,1.,0.758281796766761));
#24629=CARTESIAN_POINT('Ctrl Pts',(-1.98771456680874,-1.,0.759080037802488));
#24630=CARTESIAN_POINT('Ctrl Pts',(-1.98771456680874,1.,0.759080037802488));
#24631=CARTESIAN_POINT('Ctrl Pts',(-1.98143741418172,-1.,0.75983714745219));
#24632=CARTESIAN_POINT('Ctrl Pts',(-1.98143741418172,1.,0.75983714745219));
#24633=CARTESIAN_POINT('Ctrl Pts',(-1.97516705321494,-1.,0.760552825409757));
#24634=CARTESIAN_POINT('Ctrl Pts',(-1.97516705321494,1.,0.760552825409757));
#24635=CARTESIAN_POINT('Ctrl Pts',(-1.96890351582499,-1.,0.76122669048382));
#24636=CARTESIAN_POINT('Ctrl Pts',(-1.96890351582499,1.,0.76122669048382));
#24637=CARTESIAN_POINT('Ctrl Pts',(-1.96264672744186,-1.,0.761858300014423));
#24638=CARTESIAN_POINT('Ctrl Pts',(-1.96264672744186,1.,0.761858300014423));
#24639=CARTESIAN_POINT('Ctrl Pts',(-1.95639665309869,-1.,0.762447203806179));
#24640=CARTESIAN_POINT('Ctrl Pts',(-1.95639665309869,1.,0.762447203806179));
#24641=CARTESIAN_POINT('Ctrl Pts',(-1.95015342590024,-1.,0.762992990878769));
#24642=CARTESIAN_POINT('Ctrl Pts',(-1.95015342590024,1.,0.762992990878769));
#24643=CARTESIAN_POINT('Ctrl Pts',(-1.9439174661764,-1.,0.763495333538629));
#24644=CARTESIAN_POINT('Ctrl Pts',(-1.9439174661764,1.,0.763495333538629));
#24645=CARTESIAN_POINT('Ctrl Pts',(-1.93768964875886,-1.,0.763954049121458));
#24646=CARTESIAN_POINT('Ctrl Pts',(-1.93768964875886,1.,0.763954049121458));
#24647=CARTESIAN_POINT('Ctrl Pts',(-1.93147105496382,-1.,0.76436901067394));
#24648=CARTESIAN_POINT('Ctrl Pts',(-1.93147105496382,1.,0.76436901067394));
#24649=CARTESIAN_POINT('Ctrl Pts',(-1.92526263537048,-1.,0.764740025488211));
#24650=CARTESIAN_POINT('Ctrl Pts',(-1.92526263537048,1.,0.764740025488211));
#24651=CARTESIAN_POINT('Ctrl Pts',(-1.91906491634196,-1.,0.765066729667088));
#24652=CARTESIAN_POINT('Ctrl Pts',(-1.91906491634196,1.,0.765066729667088));
#24653=CARTESIAN_POINT('Ctrl Pts',(-1.91287765805169,-1.,0.765348465884722));
#24654=CARTESIAN_POINT('Ctrl Pts',(-1.91287765805169,1.,0.765348465884722));
#24655=CARTESIAN_POINT('Ctrl Pts',(-1.90669961402356,-1.,0.765584196937919));
#24656=CARTESIAN_POINT('Ctrl Pts',(-1.90669961402356,1.,0.765584196937919));
#24657=CARTESIAN_POINT('Ctrl Pts',(-1.90052930393596,-1.,0.765772772593386));
#24658=CARTESIAN_POINT('Ctrl Pts',(-1.90052930393596,1.,0.765772772593386));
#24659=CARTESIAN_POINT('Ctrl Pts',(-1.89436577771388,-1.,0.765913193856978));
#24660=CARTESIAN_POINT('Ctrl Pts',(-1.89436577771388,1.,0.765913193856978));
#24661=CARTESIAN_POINT('Ctrl Pts',(-1.88820926433409,-1.,0.766004837062091));
#24662=CARTESIAN_POINT('Ctrl Pts',(-1.88820926433409,1.,0.766004837062091));
#24663=CARTESIAN_POINT('Ctrl Pts',(-1.88206215302561,-1.,0.766047794851864));
#24664=CARTESIAN_POINT('Ctrl Pts',(-1.88206215302561,1.,0.766047794851864));
#24665=CARTESIAN_POINT('Ctrl Pts',(-1.87592888967883,-1.,0.766042837036744));
#24666=CARTESIAN_POINT('Ctrl Pts',(-1.87592888967883,1.,0.766042837036744));
#24667=CARTESIAN_POINT('Ctrl Pts',(-1.86981398314341,-1.,0.765990708546091));
#24668=CARTESIAN_POINT('Ctrl Pts',(-1.86981398314341,1.,0.765990708546091));
#24669=CARTESIAN_POINT('Ctrl Pts',(-1.86372027063312,-1.,0.765891519092547));
#24670=CARTESIAN_POINT('Ctrl Pts',(-1.86372027063312,1.,0.765891519092547));
#24671=CARTESIAN_POINT('Ctrl Pts',(-1.85764741390394,-1.,0.765744212909318));
#24672=CARTESIAN_POINT('Ctrl Pts',(-1.85764741390394,1.,0.765744212909318));
#24673=CARTESIAN_POINT('Ctrl Pts',(-1.85158945130063,-1.,0.765545710619062));
#24674=CARTESIAN_POINT('Ctrl Pts',(-1.85158945130063,1.,0.765545710619062));
#24675=CARTESIAN_POINT('Ctrl Pts',(-1.84553698875924,-1.,0.765291664862029));
#24676=CARTESIAN_POINT('Ctrl Pts',(-1.84553698875924,1.,0.765291664862029));
#24677=CARTESIAN_POINT('Ctrl Pts',(-1.83948181064835,-1.,0.764978057881737));
#24678=CARTESIAN_POINT('Ctrl Pts',(-1.83948181064835,1.,0.764978057881737));
#24679=CARTESIAN_POINT('Ctrl Pts',(-1.83342077227142,-1.,0.764602549687853));
#24680=CARTESIAN_POINT('Ctrl Pts',(-1.83342077227142,1.,0.764602549687853));
#24681=CARTESIAN_POINT('Ctrl Pts',(-1.82735991200065,-1.,0.764165902605995));
#24682=CARTESIAN_POINT('Ctrl Pts',(-1.82735991200065,1.,0.764165902605995));
#24683=CARTESIAN_POINT('Ctrl Pts',(-1.82131873145266,-1.,0.763673465462726));
#24684=CARTESIAN_POINT('Ctrl Pts',(-1.82131873145266,1.,0.763673465462726));
#24685=CARTESIAN_POINT('Ctrl Pts',(-1.8153211840553,-1.,0.763132003836634));
#24686=CARTESIAN_POINT('Ctrl Pts',(-1.8153211840553,1.,0.763132003836634));
#24687=CARTESIAN_POINT('Ctrl Pts',(-1.80938551463965,-1.,0.762546129463938));
#24688=CARTESIAN_POINT('Ctrl Pts',(-1.80938551463965,1.,0.762546129463938));
#24689=CARTESIAN_POINT('Ctrl Pts',(-1.80351583877342,-1.,0.761915336443547));
#24690=CARTESIAN_POINT('Ctrl Pts',(-1.80351583877342,1.,0.761915336443547));
#24691=CARTESIAN_POINT('Ctrl Pts',(-1.79768986997783,-1.,0.761229695230558));
#24692=CARTESIAN_POINT('Ctrl Pts',(-1.79768986997783,1.,0.761229695230558));
#24693=CARTESIAN_POINT('Ctrl Pts',(-1.7918581561088,-1.,0.760469555880749));
#24694=CARTESIAN_POINT('Ctrl Pts',(-1.7918581561088,1.,0.760469555880749));
#24695=CARTESIAN_POINT('Ctrl Pts',(-1.78596964884604,-1.,0.759614401110189));
#24696=CARTESIAN_POINT('Ctrl Pts',(-1.78596964884604,1.,0.759614401110189));
#24697=CARTESIAN_POINT('Ctrl Pts',(-1.77999411220945,-1.,0.758650626677518));
#24698=CARTESIAN_POINT('Ctrl Pts',(-1.77999411220945,1.,0.758650626677518));
#24699=CARTESIAN_POINT('Ctrl Pts',(-1.77394167108292,-1.,0.757578264077029));
#24700=CARTESIAN_POINT('Ctrl Pts',(-1.77394167108292,1.,0.757578264077029));
#24701=CARTESIAN_POINT('Ctrl Pts',(-1.76789396002998,-1.,0.75642189602781));
#24702=CARTESIAN_POINT('Ctrl Pts',(-1.76789396002998,1.,0.75642189602781));
#24703=CARTESIAN_POINT('Ctrl Pts',(-1.76197817240128,-1.,0.755220979974461));
#24704=CARTESIAN_POINT('Ctrl Pts',(-1.76197817240128,1.,0.755220979974461));
#24705=CARTESIAN_POINT('Ctrl Pts',(-1.75631083600019,-1.,0.754009254027829));
#24706=CARTESIAN_POINT('Ctrl Pts',(-1.75631083600019,1.,0.754009254027829));
#24707=CARTESIAN_POINT('Ctrl Pts',(-1.75095139468794,-1.,0.752797683531314));
#24708=CARTESIAN_POINT('Ctrl Pts',(-1.75095139468794,1.,0.752797683531314));
#24709=CARTESIAN_POINT('Ctrl Pts',(-1.74585086852502,-1.,0.751555614164482));
#24710=CARTESIAN_POINT('Ctrl Pts',(-1.74585086852502,1.,0.751555614164482));
#24711=CARTESIAN_POINT('Ctrl Pts',(-1.74080458267114,-1.,0.750193435981249));
#24712=CARTESIAN_POINT('Ctrl Pts',(-1.74080458267114,1.,0.750193435981249));
#24713=CARTESIAN_POINT('Ctrl Pts',(-1.7355035168033,-1.,0.74858246295687));
#24714=CARTESIAN_POINT('Ctrl Pts',(-1.7355035168033,1.,0.74858246295687));
#24715=CARTESIAN_POINT('Ctrl Pts',(-1.72958533647714,-1.,0.746574710097752));
#24716=CARTESIAN_POINT('Ctrl Pts',(-1.72958533647714,1.,0.746574710097752));
#24717=CARTESIAN_POINT('Ctrl Pts',(-1.72268229916769,-1.,0.744021445433093));
#24718=CARTESIAN_POINT('Ctrl Pts',(-1.72268229916769,1.,0.744021445433093));
#24719=CARTESIAN_POINT('Ctrl Pts',(-1.71447789751001,-1.,0.74079516202821));
#24720=CARTESIAN_POINT('Ctrl Pts',(-1.71447789751001,1.,0.74079516202821));
#24721=CARTESIAN_POINT('Ctrl Pts',(-1.70473309004249,-1.,0.736799665716932));
#24722=CARTESIAN_POINT('Ctrl Pts',(-1.70473309004249,1.,0.736799665716932));
#24723=CARTESIAN_POINT('Ctrl Pts',(-1.69326921972915,-1.,0.731963238685357));
#24724=CARTESIAN_POINT('Ctrl Pts',(-1.69326921972915,1.,0.731963238685357));
#24725=CARTESIAN_POINT('Ctrl Pts',(-1.67996158451922,-1.,0.726235967982445));
#24726=CARTESIAN_POINT('Ctrl Pts',(-1.67996158451922,1.,0.726235967982445));
#24727=CARTESIAN_POINT('Ctrl Pts',(-1.66472880551777,-1.,0.71958543378795));
#24728=CARTESIAN_POINT('Ctrl Pts',(-1.66472880551777,1.,0.71958543378795));
#24729=CARTESIAN_POINT('Ctrl Pts',(-1.64752408828442,-1.,0.711993139340447));
#24730=CARTESIAN_POINT('Ctrl Pts',(-1.64752408828442,1.,0.711993139340447));
#24731=CARTESIAN_POINT('Ctrl Pts',(-1.6321654166204,-1.,0.705159151977294));
#24732=CARTESIAN_POINT('Ctrl Pts',(-1.6321654166204,1.,0.705159151977294));
#24733=CARTESIAN_POINT('Ctrl Pts',(-1.61974673471117,-1.,0.699605146398837));
#24734=CARTESIAN_POINT('Ctrl Pts',(-1.61974673471117,1.,0.699605146398837));
#24735=CARTESIAN_POINT('Ctrl Pts',(-1.61106790957619,-1.,0.69571209787897));
#24736=CARTESIAN_POINT('Ctrl Pts',(-1.61106790957619,1.,0.69571209787897));
#24737=CARTESIAN_POINT('Ctrl Pts',(-1.60662857109684,-1.,0.693717979106305));
#24738=CARTESIAN_POINT('Ctrl Pts',(-1.60662857109684,1.,0.693717979106305));
#24739=CARTESIAN_POINT('',(-2.0698113262342,1.,0.7455743247944));
#24740=CARTESIAN_POINT('Ctrl Pts',(-2.0698113262342,1.,0.7455743247944));
#24741=CARTESIAN_POINT('Ctrl Pts',(-2.06854248895728,1.,0.745832791378367));
#24742=CARTESIAN_POINT('Ctrl Pts',(-2.06600523016815,1.,0.7463458715442));
#24743=CARTESIAN_POINT('Ctrl Pts',(-2.06220058927826,1.,0.747103932787919));
#24744=CARTESIAN_POINT('Ctrl Pts',(-2.05713023031006,1.,0.748091554183802));
#24745=CARTESIAN_POINT('Ctrl Pts',(-2.05079645592154,1.,0.749287468665046));
#24746=CARTESIAN_POINT('Ctrl Pts',(-2.04446689147979,1.,0.750444657875576));
#24747=CARTESIAN_POINT('Ctrl Pts',(-2.03814160092099,1.,0.751562963361115));
#24748=CARTESIAN_POINT('Ctrl Pts',(-2.03182068456221,1.,0.752642180487211));
#24749=CARTESIAN_POINT('Ctrl Pts',(-2.02550428623313,1.,0.753682061112768));
#24750=CARTESIAN_POINT('Ctrl Pts',(-2.01919259405809,1.,0.754682330722816));
#24751=CARTESIAN_POINT('Ctrl Pts',(-2.01288584328084,1.,0.755642704957865));
#24752=CARTESIAN_POINT('Ctrl Pts',(-2.0065843158773,1.,0.75656290464667));
#24753=CARTESIAN_POINT('Ctrl Pts',(-2.00028834739178,1.,0.757442676862724));
#24754=CARTESIAN_POINT('Ctrl Pts',(-1.99399831098817,1.,0.758281796766761));
#24755=CARTESIAN_POINT('Ctrl Pts',(-1.98771456680874,1.,0.759080037802488));
#24756=CARTESIAN_POINT('Ctrl Pts',(-1.98143741418172,1.,0.75983714745219));
#24757=CARTESIAN_POINT('Ctrl Pts',(-1.97516705321494,1.,0.760552825409757));
#24758=CARTESIAN_POINT('Ctrl Pts',(-1.96890351582499,1.,0.76122669048382));
#24759=CARTESIAN_POINT('Ctrl Pts',(-1.96264672744186,1.,0.761858300014423));
#24760=CARTESIAN_POINT('Ctrl Pts',(-1.95639665309869,1.,0.762447203806179));
#24761=CARTESIAN_POINT('Ctrl Pts',(-1.95015342590024,1.,0.762992990878769));
#24762=CARTESIAN_POINT('Ctrl Pts',(-1.9439174661764,1.,0.763495333538629));
#24763=CARTESIAN_POINT('Ctrl Pts',(-1.93768964875886,1.,0.763954049121458));
#24764=CARTESIAN_POINT('Ctrl Pts',(-1.93147105496382,1.,0.76436901067394));
#24765=CARTESIAN_POINT('Ctrl Pts',(-1.92526263537048,1.,0.764740025488211));
#24766=CARTESIAN_POINT('Ctrl Pts',(-1.91906491634196,1.,0.765066729667088));
#24767=CARTESIAN_POINT('Ctrl Pts',(-1.91287765805169,1.,0.765348465884722));
#24768=CARTESIAN_POINT('Ctrl Pts',(-1.90669961402356,1.,0.765584196937919));
#24769=CARTESIAN_POINT('Ctrl Pts',(-1.90052930393596,1.,0.765772772593386));
#24770=CARTESIAN_POINT('Ctrl Pts',(-1.89436577771388,1.,0.765913193856978));
#24771=CARTESIAN_POINT('Ctrl Pts',(-1.88820926433409,1.,0.766004837062091));
#24772=CARTESIAN_POINT('Ctrl Pts',(-1.88206215302561,1.,0.766047794851864));
#24773=CARTESIAN_POINT('Ctrl Pts',(-1.87592888967883,1.,0.766042837036744));
#24774=CARTESIAN_POINT('Ctrl Pts',(-1.86981398314341,1.,0.765990708546091));
#24775=CARTESIAN_POINT('Ctrl Pts',(-1.86372027063312,1.,0.765891519092547));
#24776=CARTESIAN_POINT('Ctrl Pts',(-1.85764741390394,1.,0.765744212909318));
#24777=CARTESIAN_POINT('Ctrl Pts',(-1.85158945130063,1.,0.765545710619062));
#24778=CARTESIAN_POINT('Ctrl Pts',(-1.84553698875924,1.,0.765291664862029));
#24779=CARTESIAN_POINT('Ctrl Pts',(-1.83948181064835,1.,0.764978057881737));
#24780=CARTESIAN_POINT('Ctrl Pts',(-1.83342077227142,1.,0.764602549687853));
#24781=CARTESIAN_POINT('Ctrl Pts',(-1.82735991200065,1.,0.764165902605995));
#24782=CARTESIAN_POINT('Ctrl Pts',(-1.82131873145266,1.,0.763673465462726));
#24783=CARTESIAN_POINT('Ctrl Pts',(-1.8153211840553,1.,0.763132003836634));
#24784=CARTESIAN_POINT('Ctrl Pts',(-1.80938551463965,1.,0.762546129463938));
#24785=CARTESIAN_POINT('Ctrl Pts',(-1.80351583877342,1.,0.761915336443547));
#24786=CARTESIAN_POINT('Ctrl Pts',(-1.79768986997783,1.,0.761229695230558));
#24787=CARTESIAN_POINT('Ctrl Pts',(-1.7918581561088,1.,0.760469555880749));
#24788=CARTESIAN_POINT('Ctrl Pts',(-1.78596964884604,1.,0.759614401110189));
#24789=CARTESIAN_POINT('Ctrl Pts',(-1.77999411220945,1.,0.758650626677518));
#24790=CARTESIAN_POINT('Ctrl Pts',(-1.77394167108292,1.,0.757578264077029));
#24791=CARTESIAN_POINT('Ctrl Pts',(-1.76789396002998,1.,0.75642189602781));
#24792=CARTESIAN_POINT('Ctrl Pts',(-1.76197817240128,1.,0.755220979974461));
#24793=CARTESIAN_POINT('Ctrl Pts',(-1.75631083600019,1.,0.754009254027829));
#24794=CARTESIAN_POINT('Ctrl Pts',(-1.75095139468794,1.,0.752797683531314));
#24795=CARTESIAN_POINT('Ctrl Pts',(-1.74585086852502,1.,0.751555614164482));
#24796=CARTESIAN_POINT('Ctrl Pts',(-1.74080458267114,1.,0.750193435981249));
#24797=CARTESIAN_POINT('Ctrl Pts',(-1.7355035168033,1.,0.74858246295687));
#24798=CARTESIAN_POINT('Ctrl Pts',(-1.72958533647714,1.,0.746574710097752));
#24799=CARTESIAN_POINT('Ctrl Pts',(-1.72268229916769,1.,0.744021445433093));
#24800=CARTESIAN_POINT('Ctrl Pts',(-1.71447789751001,1.,0.74079516202821));
#24801=CARTESIAN_POINT('Ctrl Pts',(-1.70473309004249,1.,0.736799665716932));
#24802=CARTESIAN_POINT('Ctrl Pts',(-1.69326921972915,1.,0.731963238685357));
#24803=CARTESIAN_POINT('Ctrl Pts',(-1.67996158451922,1.,0.726235967982445));
#24804=CARTESIAN_POINT('Ctrl Pts',(-1.66472880551777,1.,0.71958543378795));
#24805=CARTESIAN_POINT('Ctrl Pts',(-1.64752408828442,1.,0.711993139340447));
#24806=CARTESIAN_POINT('Ctrl Pts',(-1.6321654166204,1.,0.705159151977294));
#24807=CARTESIAN_POINT('Ctrl Pts',(-1.61974673471117,1.,0.699605146398837));
#24808=CARTESIAN_POINT('Ctrl Pts',(-1.61106790957619,1.,0.69571209787897));
#24809=CARTESIAN_POINT('Ctrl Pts',(-1.60662857109684,1.,0.693717979106305));
#24810=CARTESIAN_POINT('',(-2.0698113262342,0.,0.7455743247944));
#24811=CARTESIAN_POINT('Origin',(-2.11275013067528,0.,0.61342227326009));
#24812=CARTESIAN_POINT('',(-2.11275013067528,1.,0.61342227326009));
#24813=CARTESIAN_POINT('',(-2.0698113262342,1.,0.7455743247944));
#24814=CARTESIAN_POINT('',(-2.11275013067528,0.,0.61342227326009));
#24815=CARTESIAN_POINT('Ctrl Pts',(-1.7075470150345,-1.,0.383122945602004));
#24816=CARTESIAN_POINT('Ctrl Pts',(-1.7075470150345,1.,0.383122945602004));
#24817=CARTESIAN_POINT('Ctrl Pts',(-1.71231062891958,-1.,0.384119047315542));
#24818=CARTESIAN_POINT('Ctrl Pts',(-1.71231062891958,1.,0.384119047315542));
#24819=CARTESIAN_POINT('Ctrl Pts',(-1.72162022246158,-1.,0.38607079032701));
#24820=CARTESIAN_POINT('Ctrl Pts',(-1.72162022246158,1.,0.38607079032701));
#24821=CARTESIAN_POINT('Ctrl Pts',(-1.7349317097561,-1.,0.388877023509191));
#24822=CARTESIAN_POINT('Ctrl Pts',(-1.7349317097561,1.,0.388877023509191));
#24823=CARTESIAN_POINT('Ctrl Pts',(-1.75137405313962,-1.,0.392375812294307));
#24824=CARTESIAN_POINT('Ctrl Pts',(-1.75137405313962,1.,0.392375812294307));
#24825=CARTESIAN_POINT('Ctrl Pts',(-1.7697556004756,-1.,0.39634619612042));
#24826=CARTESIAN_POINT('Ctrl Pts',(-1.7697556004756,1.,0.39634619612042));
#24827=CARTESIAN_POINT('Ctrl Pts',(-1.78598826347533,-1.,0.39991940378308));
#24828=CARTESIAN_POINT('Ctrl Pts',(-1.78598826347533,1.,0.39991940378308));
#24829=CARTESIAN_POINT('Ctrl Pts',(-1.80012077176221,-1.,0.403107976170441));
#24830=CARTESIAN_POINT('Ctrl Pts',(-1.80012077176221,1.,0.403107976170441));
#24831=CARTESIAN_POINT('Ctrl Pts',(-1.81223801813988,-1.,0.405933518411838));
#24832=CARTESIAN_POINT('Ctrl Pts',(-1.81223801813988,1.,0.405933518411838));
#24833=CARTESIAN_POINT('Ctrl Pts',(-1.8224702267854,-1.,0.408428948108533));
#24834=CARTESIAN_POINT('Ctrl Pts',(-1.8224702267854,1.,0.408428948108533));
#24835=CARTESIAN_POINT('Ctrl Pts',(-1.83100408895216,-1.,0.410641256301675));
#24836=CARTESIAN_POINT('Ctrl Pts',(-1.83100408895216,1.,0.410641256301675));
#24837=CARTESIAN_POINT('Ctrl Pts',(-1.83808953475839,-1.,0.412633125322161));
#24838=CARTESIAN_POINT('Ctrl Pts',(-1.83808953475839,1.,0.412633125322161));
#24839=CARTESIAN_POINT('Ctrl Pts',(-1.8440575707371,-1.,0.41448743825434));
#24840=CARTESIAN_POINT('Ctrl Pts',(-1.8440575707371,1.,0.41448743825434));
#24841=CARTESIAN_POINT('Ctrl Pts',(-1.84929312929882,-1.,0.416300022038864));
#24842=CARTESIAN_POINT('Ctrl Pts',(-1.84929312929882,1.,0.416300022038864));
#24843=CARTESIAN_POINT('Ctrl Pts',(-1.85417632856234,-1.,0.418164129143534));
#24844=CARTESIAN_POINT('Ctrl Pts',(-1.85417632856234,1.,0.418164129143534));
#24845=CARTESIAN_POINT('Ctrl Pts',(-1.85903281096686,-1.,0.420157287975619));
#24846=CARTESIAN_POINT('Ctrl Pts',(-1.85903281096686,1.,0.420157287975619));
#24847=CARTESIAN_POINT('Ctrl Pts',(-1.86408083334028,-1.,0.422327307418275));
#24848=CARTESIAN_POINT('Ctrl Pts',(-1.86408083334028,1.,0.422327307418275));
#24849=CARTESIAN_POINT('Ctrl Pts',(-1.86937803944323,-1.,0.424678177291359));
#24850=CARTESIAN_POINT('Ctrl Pts',(-1.86937803944323,1.,0.424678177291359));
#24851=CARTESIAN_POINT('Ctrl Pts',(-1.87486989291484,-1.,0.427183828519102));
#24852=CARTESIAN_POINT('Ctrl Pts',(-1.87486989291484,1.,0.427183828519102));
#24853=CARTESIAN_POINT('Ctrl Pts',(-1.88044229001832,-1.,0.429803062482344));
#24854=CARTESIAN_POINT('Ctrl Pts',(-1.88044229001832,1.,0.429803062482344));
#24855=CARTESIAN_POINT('Ctrl Pts',(-1.88596913666793,-1.,0.432493038548748));
#24856=CARTESIAN_POINT('Ctrl Pts',(-1.88596913666793,1.,0.432493038548748));
#24857=CARTESIAN_POINT('Ctrl Pts',(-1.89136993975504,-1.,0.435225660963383));
#24858=CARTESIAN_POINT('Ctrl Pts',(-1.89136993975504,1.,0.435225660963383));
#24859=CARTESIAN_POINT('Ctrl Pts',(-1.89663648956466,-1.,0.437995003948244));
#24860=CARTESIAN_POINT('Ctrl Pts',(-1.89663648956466,1.,0.437995003948244));
#24861=CARTESIAN_POINT('Ctrl Pts',(-1.90180124389086,-1.,0.440807833704038));
#24862=CARTESIAN_POINT('Ctrl Pts',(-1.90180124389086,1.,0.440807833704038));
#24863=CARTESIAN_POINT('Ctrl Pts',(-1.90691756144898,-1.,0.44367755684915));
#24864=CARTESIAN_POINT('Ctrl Pts',(-1.90691756144898,1.,0.44367755684915));
#24865=CARTESIAN_POINT('Ctrl Pts',(-1.9120369998112,-1.,0.446617343485711));
#24866=CARTESIAN_POINT('Ctrl Pts',(-1.9120369998112,1.,0.446617343485711));
#24867=CARTESIAN_POINT('Ctrl Pts',(-1.91718342555755,-1.,0.449632260106662));
#24868=CARTESIAN_POINT('Ctrl Pts',(-1.91718342555755,1.,0.449632260106662));
#24869=CARTESIAN_POINT('Ctrl Pts',(-1.92235380648502,-1.,0.452719478359432));
#24870=CARTESIAN_POINT('Ctrl Pts',(-1.92235380648502,1.,0.452719478359432));
#24871=CARTESIAN_POINT('Ctrl Pts',(-1.92753067150476,-1.,0.455872005174371));
#24872=CARTESIAN_POINT('Ctrl Pts',(-1.92753067150476,1.,0.455872005174371));
#24873=CARTESIAN_POINT('Ctrl Pts',(-1.93269066517934,-1.,0.459081234547926));
#24874=CARTESIAN_POINT('Ctrl Pts',(-1.93269066517934,1.,0.459081234547926));
#24875=CARTESIAN_POINT('Ctrl Pts',(-1.93781486640821,-1.,0.462340031009056));
#24876=CARTESIAN_POINT('Ctrl Pts',(-1.93781486640821,1.,0.462340031009056));
#24877=CARTESIAN_POINT('Ctrl Pts',(-1.9428979419619,-1.,0.46564546202603));
#24878=CARTESIAN_POINT('Ctrl Pts',(-1.9428979419619,1.,0.46564546202603));
#24879=CARTESIAN_POINT('Ctrl Pts',(-1.94794381136514,-1.,0.468997482913135));
#24880=CARTESIAN_POINT('Ctrl Pts',(-1.94794381136514,1.,0.468997482913135));
#24881=CARTESIAN_POINT('Ctrl Pts',(-1.95296148278133,-1.,0.472397672264072));
#24882=CARTESIAN_POINT('Ctrl Pts',(-1.95296148278133,1.,0.472397672264072));
#24883=CARTESIAN_POINT('Ctrl Pts',(-1.95796111148177,-1.,0.475848034683176));
#24884=CARTESIAN_POINT('Ctrl Pts',(-1.95796111148177,1.,0.475848034683176));
#24885=CARTESIAN_POINT('Ctrl Pts',(-1.96294933055943,-1.,0.479349583074855));
#24886=CARTESIAN_POINT('Ctrl Pts',(-1.96294933055943,1.,0.479349583074855));
#24887=CARTESIAN_POINT('Ctrl Pts',(-1.96792703422362,-1.,0.48290166212069));
#24888=CARTESIAN_POINT('Ctrl Pts',(-1.96792703422362,1.,0.48290166212069));
#24889=CARTESIAN_POINT('Ctrl Pts',(-1.97289186263272,-1.,0.486502692907659));
#24890=CARTESIAN_POINT('Ctrl Pts',(-1.97289186263272,1.,0.486502692907659));
#24891=CARTESIAN_POINT('Ctrl Pts',(-1.97783973019229,-1.,0.490150627860952));
#24892=CARTESIAN_POINT('Ctrl Pts',(-1.97783973019229,1.,0.490150627860952));
#24893=CARTESIAN_POINT('Ctrl Pts',(-1.98276658761821,-1.,0.493843476541494));
#24894=CARTESIAN_POINT('Ctrl Pts',(-1.98276658761821,1.,0.493843476541494));
#24895=CARTESIAN_POINT('Ctrl Pts',(-1.98767044752932,-1.,0.497579909545574));
#24896=CARTESIAN_POINT('Ctrl Pts',(-1.98767044752932,1.,0.497579909545574));
#24897=CARTESIAN_POINT('Ctrl Pts',(-1.99255149126155,-1.,0.501359287727146));
#24898=CARTESIAN_POINT('Ctrl Pts',(-1.99255149126155,1.,0.501359287727146));
#24899=CARTESIAN_POINT('Ctrl Pts',(-1.99741107463572,-1.,0.505181361323026));
#24900=CARTESIAN_POINT('Ctrl Pts',(-1.99741107463572,1.,0.505181361323026));
#24901=CARTESIAN_POINT('Ctrl Pts',(-2.00225107134734,-1.,0.509046069886157));
#24902=CARTESIAN_POINT('Ctrl Pts',(-2.00225107134734,1.,0.509046069886157));
#24903=CARTESIAN_POINT('Ctrl Pts',(-2.00707309946949,-1.,0.512953306961792));
#24904=CARTESIAN_POINT('Ctrl Pts',(-2.00707309946949,1.,0.512953306961792));
#24905=CARTESIAN_POINT('Ctrl Pts',(-2.01187773939242,-1.,0.516902681728687));
#24906=CARTESIAN_POINT('Ctrl Pts',(-2.01187773939242,1.,0.516902681728687));
#24907=CARTESIAN_POINT('Ctrl Pts',(-2.01666477917286,-1.,0.52089359039937));
#24908=CARTESIAN_POINT('Ctrl Pts',(-2.01666477917286,1.,0.52089359039937));
#24909=CARTESIAN_POINT('Ctrl Pts',(-2.02143356304698,-1.,0.524925318333476));
#24910=CARTESIAN_POINT('Ctrl Pts',(-2.02143356304698,1.,0.524925318333476));
#24911=CARTESIAN_POINT('Ctrl Pts',(-2.0261832908329,-1.,0.528997127241914));
#24912=CARTESIAN_POINT('Ctrl Pts',(-2.0261832908329,1.,0.528997127241914));
#24913=CARTESIAN_POINT('Ctrl Pts',(-2.03091336214426,-1.,0.533108355132976));
#24914=CARTESIAN_POINT('Ctrl Pts',(-2.03091336214426,1.,0.533108355132976));
#24915=CARTESIAN_POINT('Ctrl Pts',(-2.03562362954037,-1.,0.537258489833262));
#24916=CARTESIAN_POINT('Ctrl Pts',(-2.03562362954037,1.,0.537258489833262));
#24917=CARTESIAN_POINT('Ctrl Pts',(-2.04031422690527,-1.,0.541447120615659));
#24918=CARTESIAN_POINT('Ctrl Pts',(-2.04031422690527,1.,0.541447120615659));
#24919=CARTESIAN_POINT('Ctrl Pts',(-2.04498544714588,-1.,0.54567390381743));
#24920=CARTESIAN_POINT('Ctrl Pts',(-2.04498544714588,1.,0.54567390381743));
#24921=CARTESIAN_POINT('Ctrl Pts',(-2.04963761077958,-1.,0.549938525150295));
#24922=CARTESIAN_POINT('Ctrl Pts',(-2.04963761077958,1.,0.549938525150295));
#24923=CARTESIAN_POINT('Ctrl Pts',(-2.05427091604413,-1.,0.554240657463906));
#24924=CARTESIAN_POINT('Ctrl Pts',(-2.05427091604413,1.,0.554240657463906));
#24925=CARTESIAN_POINT('Ctrl Pts',(-2.05888537756462,-1.,0.558579940185151));
#24926=CARTESIAN_POINT('Ctrl Pts',(-2.05888537756462,1.,0.558579940185151));
#24927=CARTESIAN_POINT('Ctrl Pts',(-2.06348090160589,-1.,0.562955993082261));
#24928=CARTESIAN_POINT('Ctrl Pts',(-2.06348090160589,1.,0.562955993082261));
#24929=CARTESIAN_POINT('Ctrl Pts',(-2.06805732997334,-1.,0.567368421181087));
#24930=CARTESIAN_POINT('Ctrl Pts',(-2.06805732997334,1.,0.567368421181087));
#24931=CARTESIAN_POINT('Ctrl Pts',(-2.07261449292824,-1.,0.571816823242603));
#24932=CARTESIAN_POINT('Ctrl Pts',(-2.07261449292824,1.,0.571816823242603));
#24933=CARTESIAN_POINT('Ctrl Pts',(-2.07715226767559,-1.,0.576300797416844));
#24934=CARTESIAN_POINT('Ctrl Pts',(-2.07715226767559,1.,0.576300797416844));
#24935=CARTESIAN_POINT('Ctrl Pts',(-2.08167059018418,-1.,0.580819952108063));
#24936=CARTESIAN_POINT('Ctrl Pts',(-2.08167059018418,1.,0.580819952108063));
#24937=CARTESIAN_POINT('Ctrl Pts',(-2.08616943727951,-1.,0.585373918991617));
#24938=CARTESIAN_POINT('Ctrl Pts',(-2.08616943727951,1.,0.585373918991617));
#24939=CARTESIAN_POINT('Ctrl Pts',(-2.09064881812129,-1.,0.589962365403406));
#24940=CARTESIAN_POINT('Ctrl Pts',(-2.09064881812129,1.,0.589962365403406));
#24941=CARTESIAN_POINT('Ctrl Pts',(-2.0951087622027,-1.,0.594585006052162));
#24942=CARTESIAN_POINT('Ctrl Pts',(-2.0951087622027,1.,0.594585006052162));
#24943=CARTESIAN_POINT('Ctrl Pts',(-2.0995493086477,-1.,0.599241616420533));
#24944=CARTESIAN_POINT('Ctrl Pts',(-2.0995493086477,1.,0.599241616420533));
#24945=CARTESIAN_POINT('Ctrl Pts',(-2.10397049886949,-1.,0.60393203073603));
#24946=CARTESIAN_POINT('Ctrl Pts',(-2.10397049886949,1.,0.60393203073603));
#24947=CARTESIAN_POINT('Ctrl Pts',(-2.1074919961518,-1.,0.607711315454876));
#24948=CARTESIAN_POINT('Ctrl Pts',(-2.1074919961518,1.,0.607711315454876));
#24949=CARTESIAN_POINT('Ctrl Pts',(-2.11012443807238,-1.,0.610560911689899));
#24950=CARTESIAN_POINT('Ctrl Pts',(-2.11012443807238,1.,0.610560911689899));
#24951=CARTESIAN_POINT('Ctrl Pts',(-2.11187554259986,-1.,0.6124673655618));
#24952=CARTESIAN_POINT('Ctrl Pts',(-2.11187554259986,1.,0.6124673655618));
#24953=CARTESIAN_POINT('Ctrl Pts',(-2.11275013067528,-1.,0.61342227326009));
#24954=CARTESIAN_POINT('Ctrl Pts',(-2.11275013067528,1.,0.61342227326009));
#24955=CARTESIAN_POINT('',(-1.7075470150345,1.,0.383122945602004));
#24956=CARTESIAN_POINT('Ctrl Pts',(-1.7075470150345,1.,0.383122945602004));
#24957=CARTESIAN_POINT('Ctrl Pts',(-1.71231062891958,1.,0.384119047315542));
#24958=CARTESIAN_POINT('Ctrl Pts',(-1.72162022246158,1.,0.38607079032701));
#24959=CARTESIAN_POINT('Ctrl Pts',(-1.7349317097561,1.,0.388877023509191));
#24960=CARTESIAN_POINT('Ctrl Pts',(-1.75137405313962,1.,0.392375812294307));
#24961=CARTESIAN_POINT('Ctrl Pts',(-1.7697556004756,1.,0.39634619612042));
#24962=CARTESIAN_POINT('Ctrl Pts',(-1.78598826347533,1.,0.39991940378308));
#24963=CARTESIAN_POINT('Ctrl Pts',(-1.80012077176221,1.,0.403107976170441));
#24964=CARTESIAN_POINT('Ctrl Pts',(-1.81223801813988,1.,0.405933518411838));
#24965=CARTESIAN_POINT('Ctrl Pts',(-1.8224702267854,1.,0.408428948108533));
#24966=CARTESIAN_POINT('Ctrl Pts',(-1.83100408895216,1.,0.410641256301675));
#24967=CARTESIAN_POINT('Ctrl Pts',(-1.83808953475839,1.,0.412633125322161));
#24968=CARTESIAN_POINT('Ctrl Pts',(-1.8440575707371,1.,0.41448743825434));
#24969=CARTESIAN_POINT('Ctrl Pts',(-1.84929312929882,1.,0.416300022038864));
#24970=CARTESIAN_POINT('Ctrl Pts',(-1.85417632856234,1.,0.418164129143534));
#24971=CARTESIAN_POINT('Ctrl Pts',(-1.85903281096686,1.,0.420157287975619));
#24972=CARTESIAN_POINT('Ctrl Pts',(-1.86408083334028,1.,0.422327307418275));
#24973=CARTESIAN_POINT('Ctrl Pts',(-1.86937803944323,1.,0.424678177291359));
#24974=CARTESIAN_POINT('Ctrl Pts',(-1.87486989291484,1.,0.427183828519102));
#24975=CARTESIAN_POINT('Ctrl Pts',(-1.88044229001832,1.,0.429803062482344));
#24976=CARTESIAN_POINT('Ctrl Pts',(-1.88596913666793,1.,0.432493038548748));
#24977=CARTESIAN_POINT('Ctrl Pts',(-1.89136993975504,1.,0.435225660963383));
#24978=CARTESIAN_POINT('Ctrl Pts',(-1.89663648956466,1.,0.437995003948244));
#24979=CARTESIAN_POINT('Ctrl Pts',(-1.90180124389086,1.,0.440807833704038));
#24980=CARTESIAN_POINT('Ctrl Pts',(-1.90691756144898,1.,0.44367755684915));
#24981=CARTESIAN_POINT('Ctrl Pts',(-1.9120369998112,1.,0.446617343485711));
#24982=CARTESIAN_POINT('Ctrl Pts',(-1.91718342555755,1.,0.449632260106662));
#24983=CARTESIAN_POINT('Ctrl Pts',(-1.92235380648502,1.,0.452719478359432));
#24984=CARTESIAN_POINT('Ctrl Pts',(-1.92753067150476,1.,0.455872005174371));
#24985=CARTESIAN_POINT('Ctrl Pts',(-1.93269066517934,1.,0.459081234547926));
#24986=CARTESIAN_POINT('Ctrl Pts',(-1.93781486640821,1.,0.462340031009056));
#24987=CARTESIAN_POINT('Ctrl Pts',(-1.9428979419619,1.,0.46564546202603));
#24988=CARTESIAN_POINT('Ctrl Pts',(-1.94794381136514,1.,0.468997482913135));
#24989=CARTESIAN_POINT('Ctrl Pts',(-1.95296148278133,1.,0.472397672264072));
#24990=CARTESIAN_POINT('Ctrl Pts',(-1.95796111148177,1.,0.475848034683176));
#24991=CARTESIAN_POINT('Ctrl Pts',(-1.96294933055943,1.,0.479349583074855));
#24992=CARTESIAN_POINT('Ctrl Pts',(-1.96792703422362,1.,0.48290166212069));
#24993=CARTESIAN_POINT('Ctrl Pts',(-1.97289186263272,1.,0.486502692907659));
#24994=CARTESIAN_POINT('Ctrl Pts',(-1.97783973019229,1.,0.490150627860952));
#24995=CARTESIAN_POINT('Ctrl Pts',(-1.98276658761821,1.,0.493843476541494));
#24996=CARTESIAN_POINT('Ctrl Pts',(-1.98767044752932,1.,0.497579909545574));
#24997=CARTESIAN_POINT('Ctrl Pts',(-1.99255149126155,1.,0.501359287727146));
#24998=CARTESIAN_POINT('Ctrl Pts',(-1.99741107463572,1.,0.505181361323026));
#24999=CARTESIAN_POINT('Ctrl Pts',(-2.00225107134734,1.,0.509046069886157));
#25000=CARTESIAN_POINT('Ctrl Pts',(-2.00707309946949,1.,0.512953306961792));
#25001=CARTESIAN_POINT('Ctrl Pts',(-2.01187773939242,1.,0.516902681728687));
#25002=CARTESIAN_POINT('Ctrl Pts',(-2.01666477917286,1.,0.52089359039937));
#25003=CARTESIAN_POINT('Ctrl Pts',(-2.02143356304698,1.,0.524925318333476));
#25004=CARTESIAN_POINT('Ctrl Pts',(-2.0261832908329,1.,0.528997127241914));
#25005=CARTESIAN_POINT('Ctrl Pts',(-2.03091336214426,1.,0.533108355132976));
#25006=CARTESIAN_POINT('Ctrl Pts',(-2.03562362954037,1.,0.537258489833262));
#25007=CARTESIAN_POINT('Ctrl Pts',(-2.04031422690527,1.,0.541447120615659));
#25008=CARTESIAN_POINT('Ctrl Pts',(-2.04498544714588,1.,0.54567390381743));
#25009=CARTESIAN_POINT('Ctrl Pts',(-2.04963761077958,1.,0.549938525150295));
#25010=CARTESIAN_POINT('Ctrl Pts',(-2.05427091604413,1.,0.554240657463906));
#25011=CARTESIAN_POINT('Ctrl Pts',(-2.05888537756462,1.,0.558579940185151));
#25012=CARTESIAN_POINT('Ctrl Pts',(-2.06348090160589,1.,0.562955993082261));
#25013=CARTESIAN_POINT('Ctrl Pts',(-2.06805732997334,1.,0.567368421181087));
#25014=CARTESIAN_POINT('Ctrl Pts',(-2.07261449292824,1.,0.571816823242603));
#25015=CARTESIAN_POINT('Ctrl Pts',(-2.07715226767559,1.,0.576300797416844));
#25016=CARTESIAN_POINT('Ctrl Pts',(-2.08167059018418,1.,0.580819952108063));
#25017=CARTESIAN_POINT('Ctrl Pts',(-2.08616943727951,1.,0.585373918991617));
#25018=CARTESIAN_POINT('Ctrl Pts',(-2.09064881812129,1.,0.589962365403406));
#25019=CARTESIAN_POINT('Ctrl Pts',(-2.0951087622027,1.,0.594585006052162));
#25020=CARTESIAN_POINT('Ctrl Pts',(-2.0995493086477,1.,0.599241616420533));
#25021=CARTESIAN_POINT('Ctrl Pts',(-2.10397049886949,1.,0.60393203073603));
#25022=CARTESIAN_POINT('Ctrl Pts',(-2.1074919961518,1.,0.607711315454876));
#25023=CARTESIAN_POINT('Ctrl Pts',(-2.11012443807238,1.,0.610560911689899));
#25024=CARTESIAN_POINT('Ctrl Pts',(-2.11187554259986,1.,0.6124673655618));
#25025=CARTESIAN_POINT('Ctrl Pts',(-2.11275013067528,1.,0.61342227326009));
#25026=CARTESIAN_POINT('',(-1.7075470150345,0.,0.383122945602003));
#25027=CARTESIAN_POINT('Origin',(0.,0.,0.));
#25028=CARTESIAN_POINT('',(-1.74236521665491,1.,0.163289472382896));
#25029=CARTESIAN_POINT('Origin',(0.,1.,0.));
#25030=CARTESIAN_POINT('',(-1.74236521665491,0.,0.163289472382896));
#25031=CARTESIAN_POINT('Ctrl Pts',(-2.19890268624765,-1.,0.069476445021958));
#25032=CARTESIAN_POINT('Ctrl Pts',(-2.19890268624765,1.,0.069476445021958));
#25033=CARTESIAN_POINT('Ctrl Pts',(-2.19777582085423,-1.,0.0701143536325489));
#25034=CARTESIAN_POINT('Ctrl Pts',(-2.19777582085423,1.,0.0701143536325489));
#25035=CARTESIAN_POINT('Ctrl Pts',(-2.19552129484002,-1.,0.0713863779526153));
#25036=CARTESIAN_POINT('Ctrl Pts',(-2.19552129484002,1.,0.0713863779526153));
#25037=CARTESIAN_POINT('Ctrl Pts',(-2.19213712013662,-1.,0.0732830357306724));
#25038=CARTESIAN_POINT('Ctrl Pts',(-2.19213712013662,1.,0.0732830357306724));
#25039=CARTESIAN_POINT('Ctrl Pts',(-2.1876201139953,-1.,0.0757891465836146));
#25040=CARTESIAN_POINT('Ctrl Pts',(-2.1876201139953,1.,0.0757891465836146));
#25041=CARTESIAN_POINT('Ctrl Pts',(-2.18196589448887,-1.,0.0788837727685241));
#25042=CARTESIAN_POINT('Ctrl Pts',(-2.18196589448887,1.,0.0788837727685241));
#25043=CARTESIAN_POINT('Ctrl Pts',(-2.176303712113,-1.,0.0819402680872764));
#25044=CARTESIAN_POINT('Ctrl Pts',(-2.176303712113,1.,0.0819402680872764));
#25045=CARTESIAN_POINT('Ctrl Pts',(-2.17063357870952,-1.,0.0849584620835371));
#25046=CARTESIAN_POINT('Ctrl Pts',(-2.17063357870952,1.,0.0849584620835371));
#25047=CARTESIAN_POINT('Ctrl Pts',(-2.16495552645014,-1.,0.0879381291386921));
#25048=CARTESIAN_POINT('Ctrl Pts',(-2.16495552645014,1.,0.0879381291386921));
#25049=CARTESIAN_POINT('Ctrl Pts',(-2.15926961544516,-1.,0.0908789888107264));
#25050=CARTESIAN_POINT('Ctrl Pts',(-2.15926961544516,1.,0.0908789888107264));
#25051=CARTESIAN_POINT('Ctrl Pts',(-2.1535759397817,-1.,0.0937807218867642));
#25052=CARTESIAN_POINT('Ctrl Pts',(-2.1535759397817,1.,0.0937807218867642));
#25053=CARTESIAN_POINT('Ctrl Pts',(-2.14787463531795,-1.,0.0966429852305457));
#25054=CARTESIAN_POINT('Ctrl Pts',(-2.14787463531795,1.,0.0966429852305457));
#25055=CARTESIAN_POINT('Ctrl Pts',(-2.14216588396025,-1.,0.0994654261990914));
#25056=CARTESIAN_POINT('Ctrl Pts',(-2.14216588396025,1.,0.0994654261990914));
#25057=CARTESIAN_POINT('Ctrl Pts',(-2.13644992667165,-1.,0.1022477005561));
#25058=CARTESIAN_POINT('Ctrl Pts',(-2.13644992667165,1.,0.1022477005561));
#25059=CARTESIAN_POINT('Ctrl Pts',(-2.13072704887293,-1.,0.104989479152739));
#25060=CARTESIAN_POINT('Ctrl Pts',(-2.13072704887293,1.,0.104989479152739));
#25061=CARTESIAN_POINT('Ctrl Pts',(-2.12499752307,-1.,0.10769043523109));
#25062=CARTESIAN_POINT('Ctrl Pts',(-2.12499752307,1.,0.10769043523109));
#25063=CARTESIAN_POINT('Ctrl Pts',(-2.11926155590865,-1.,0.110350236135025));
#25064=CARTESIAN_POINT('Ctrl Pts',(-2.11926155590865,1.,0.110350236135025));
#25065=CARTESIAN_POINT('Ctrl Pts',(-2.11351924490306,-1.,0.112968534419737));
#25066=CARTESIAN_POINT('Ctrl Pts',(-2.11351924490306,1.,0.112968534419737));
#25067=CARTESIAN_POINT('Ctrl Pts',(-2.10777050261309,-1.,0.115544957687926));
#25068=CARTESIAN_POINT('Ctrl Pts',(-2.10777050261309,1.,0.115544957687926));
#25069=CARTESIAN_POINT('Ctrl Pts',(-2.102015121329,-1.,0.118079107988355));
#25070=CARTESIAN_POINT('Ctrl Pts',(-2.102015121329,1.,0.118079107988355));
#25071=CARTESIAN_POINT('Ctrl Pts',(-2.0962529286773,-1.,0.120570567965122));
#25072=CARTESIAN_POINT('Ctrl Pts',(-2.0962529286773,1.,0.120570567965122));
#25073=CARTESIAN_POINT('Ctrl Pts',(-2.09048392424825,-1.,0.123018905621083));
#25074=CARTESIAN_POINT('Ctrl Pts',(-2.09048392424825,1.,0.123018905621083));
#25075=CARTESIAN_POINT('Ctrl Pts',(-2.08470840653643,-1.,0.125423679412061));
#25076=CARTESIAN_POINT('Ctrl Pts',(-2.08470840653643,1.,0.125423679412061));
#25077=CARTESIAN_POINT('Ctrl Pts',(-2.07892715110987,-1.,0.12778444527612));
#25078=CARTESIAN_POINT('Ctrl Pts',(-2.07892715110987,1.,0.12778444527612));
#25079=CARTESIAN_POINT('Ctrl Pts',(-2.07314114713063,-1.,0.130100748328403));
#25080=CARTESIAN_POINT('Ctrl Pts',(-2.07314114713063,1.,0.130100748328403));
#25081=CARTESIAN_POINT('Ctrl Pts',(-2.06735123910326,-1.,0.13237211154771));
#25082=CARTESIAN_POINT('Ctrl Pts',(-2.06735123910326,1.,0.13237211154771));
#25083=CARTESIAN_POINT('Ctrl Pts',(-2.06155781517842,-1.,0.134598026192106));
#25084=CARTESIAN_POINT('Ctrl Pts',(-2.06155781517842,1.,0.134598026192106));
#25085=CARTESIAN_POINT('Ctrl Pts',(-2.05576044414264,-1.,0.136777941218043));
#25086=CARTESIAN_POINT('Ctrl Pts',(-2.05576044414264,1.,0.136777941218043));
#25087=CARTESIAN_POINT('Ctrl Pts',(-2.04995762001328,-1.,0.138911255368966));
#25088=CARTESIAN_POINT('Ctrl Pts',(-2.04995762001328,1.,0.138911255368966));
#25089=CARTESIAN_POINT('Ctrl Pts',(-2.04414757947916,-1.,0.140997332152546));
#25090=CARTESIAN_POINT('Ctrl Pts',(-2.04414757947916,1.,0.140997332152546));
#25091=CARTESIAN_POINT('Ctrl Pts',(-2.03832911025912,-1.,0.143035515058209));
#25092=CARTESIAN_POINT('Ctrl Pts',(-2.03832911025912,1.,0.143035515058209));
#25093=CARTESIAN_POINT('Ctrl Pts',(-2.03250223739942,-1.,0.145025140186057));
#25094=CARTESIAN_POINT('Ctrl Pts',(-2.03250223739942,1.,0.145025140186057));
#25095=CARTESIAN_POINT('Ctrl Pts',(-2.02666926182017,-1.,0.146965557332583));
#25096=CARTESIAN_POINT('Ctrl Pts',(-2.02666926182017,1.,0.146965557332583));
#25097=CARTESIAN_POINT('Ctrl Pts',(-2.02083464969894,-1.,0.148856124775337));
#25098=CARTESIAN_POINT('Ctrl Pts',(-2.02083464969894,1.,0.148856124775337));
#25099=CARTESIAN_POINT('Ctrl Pts',(-2.01500291940238,-1.,0.150696157673078));
#25100=CARTESIAN_POINT('Ctrl Pts',(-2.01500291940238,1.,0.150696157673078));
#25101=CARTESIAN_POINT('Ctrl Pts',(-2.00917680318424,-1.,0.15248488362145));
#25102=CARTESIAN_POINT('Ctrl Pts',(-2.00917680318424,1.,0.15248488362145));
#25103=CARTESIAN_POINT('Ctrl Pts',(-2.00335565310543,-1.,0.154221403049722));
#25104=CARTESIAN_POINT('Ctrl Pts',(-2.00335565310543,1.,0.154221403049722));
#25105=CARTESIAN_POINT('Ctrl Pts',(-1.99753284771497,-1.,0.155904629548783));
#25106=CARTESIAN_POINT('Ctrl Pts',(-1.99753284771497,1.,0.155904629548783));
#25107=CARTESIAN_POINT('Ctrl Pts',(-1.99169810931908,-1.,0.157533331459227));
#25108=CARTESIAN_POINT('Ctrl Pts',(-1.99169810931908,1.,0.157533331459227));
#25109=CARTESIAN_POINT('Ctrl Pts',(-1.98584238283292,-1.,0.159106226437299));
#25110=CARTESIAN_POINT('Ctrl Pts',(-1.98584238283292,1.,0.159106226437299));
#25111=CARTESIAN_POINT('Ctrl Pts',(-1.97996195437559,-1.,0.160622060784611));
#25112=CARTESIAN_POINT('Ctrl Pts',(-1.97996195437559,1.,0.160622060784611));
#25113=CARTESIAN_POINT('Ctrl Pts',(-1.97406280235188,-1.,0.162079693556288));
#25114=CARTESIAN_POINT('Ctrl Pts',(-1.97406280235188,1.,0.162079693556288));
#25115=CARTESIAN_POINT('Ctrl Pts',(-1.96816512677967,-1.,0.163478185457734));
#25116=CARTESIAN_POINT('Ctrl Pts',(-1.96816512677967,1.,0.163478185457734));
#25117=CARTESIAN_POINT('Ctrl Pts',(-1.96229379940136,-1.,0.164816568920269));
#25118=CARTESIAN_POINT('Ctrl Pts',(-1.96229379940136,1.,0.164816568920269));
#25119=CARTESIAN_POINT('Ctrl Pts',(-1.9564675971873,-1.,0.166093592002812));
#25120=CARTESIAN_POINT('Ctrl Pts',(-1.9564675971873,1.,0.166093592002812));
#25121=CARTESIAN_POINT('Ctrl Pts',(-1.95069027794294,-1.,0.167307501784475));
#25122=CARTESIAN_POINT('Ctrl Pts',(-1.95069027794294,1.,0.167307501784475));
#25123=CARTESIAN_POINT('Ctrl Pts',(-1.94493757756931,-1.,0.168455741607556));
#25124=CARTESIAN_POINT('Ctrl Pts',(-1.94493757756931,1.,0.168455741607556));
#25125=CARTESIAN_POINT('Ctrl Pts',(-1.93915639211581,-1.,0.169534904817491));
#25126=CARTESIAN_POINT('Ctrl Pts',(-1.93915639211581,1.,0.169534904817491));
#25127=CARTESIAN_POINT('Ctrl Pts',(-1.93329183155539,-1.,0.170541253116201));
#25128=CARTESIAN_POINT('Ctrl Pts',(-1.93329183155539,1.,0.170541253116201));
#25129=CARTESIAN_POINT('Ctrl Pts',(-1.92731093582036,-1.,0.171471191532988));
#25130=CARTESIAN_POINT('Ctrl Pts',(-1.92731093582036,1.,0.171471191532988));
#25131=CARTESIAN_POINT('Ctrl Pts',(-1.9212233439798,-1.,0.172321621259514));
#25132=CARTESIAN_POINT('Ctrl Pts',(-1.9212233439798,1.,0.172321621259514));
#25133=CARTESIAN_POINT('Ctrl Pts',(-1.91511429159527,-1.,0.173090695383496));
#25134=CARTESIAN_POINT('Ctrl Pts',(-1.91511429159527,1.,0.173090695383496));
#25135=CARTESIAN_POINT('Ctrl Pts',(-1.90911693975267,-1.,0.173776635257817));
#25136=CARTESIAN_POINT('Ctrl Pts',(-1.90911693975267,1.,0.173776635257817));
#25137=CARTESIAN_POINT('Ctrl Pts',(-1.90335253862834,-1.,0.174375518661085));
#25138=CARTESIAN_POINT('Ctrl Pts',(-1.90335253862834,1.,0.174375518661085));
#25139=CARTESIAN_POINT('Ctrl Pts',(-1.89788101117132,-1.,0.174879405091263));
#25140=CARTESIAN_POINT('Ctrl Pts',(-1.89788101117132,1.,0.174879405091263));
#25141=CARTESIAN_POINT('Ctrl Pts',(-1.892646301985,-1.,0.175274276190844));
#25142=CARTESIAN_POINT('Ctrl Pts',(-1.892646301985,1.,0.175274276190844));
#25143=CARTESIAN_POINT('Ctrl Pts',(-1.88742606273259,-1.,0.175538155840648));
#25144=CARTESIAN_POINT('Ctrl Pts',(-1.88742606273259,1.,0.175538155840648));
#25145=CARTESIAN_POINT('Ctrl Pts',(-1.88188663145367,-1.,0.175644148889698));
#25146=CARTESIAN_POINT('Ctrl Pts',(-1.88188663145367,1.,0.175644148889698));
#25147=CARTESIAN_POINT('Ctrl Pts',(-1.87563767773588,-1.,0.175563480746485));
#25148=CARTESIAN_POINT('Ctrl Pts',(-1.87563767773588,1.,0.175563480746485));
#25149=CARTESIAN_POINT('Ctrl Pts',(-1.86828349694799,-1.,0.175268337590758));
#25150=CARTESIAN_POINT('Ctrl Pts',(-1.86828349694799,1.,0.175268337590758));
#25151=CARTESIAN_POINT('Ctrl Pts',(-1.85948367088837,-1.,0.17473525927603));
#25152=CARTESIAN_POINT('Ctrl Pts',(-1.85948367088837,1.,0.17473525927603));
#25153=CARTESIAN_POINT('Ctrl Pts',(-1.8489811319852,-1.,0.173946627587731));
#25154=CARTESIAN_POINT('Ctrl Pts',(-1.8489811319852,1.,0.173946627587731));
#25155=CARTESIAN_POINT('Ctrl Pts',(-1.83658380527692,-1.,0.1728894428919));
#25156=CARTESIAN_POINT('Ctrl Pts',(-1.83658380527692,1.,0.1728894428919));
#25157=CARTESIAN_POINT('Ctrl Pts',(-1.82215766811545,-1.,0.171554770204119));
#25158=CARTESIAN_POINT('Ctrl Pts',(-1.82215766811545,1.,0.171554770204119));
#25159=CARTESIAN_POINT('Ctrl Pts',(-1.80561530629706,-1.,0.169936923904608));
#25160=CARTESIAN_POINT('Ctrl Pts',(-1.80561530629706,1.,0.169936923904608));
#25161=CARTESIAN_POINT('Ctrl Pts',(-1.7869064998507,-1.,0.168032772805197));
#25162=CARTESIAN_POINT('Ctrl Pts',(-1.7869064998507,1.,0.168032772805197));
#25163=CARTESIAN_POINT('Ctrl Pts',(-1.77018771684844,-1.,0.1662793551464));
#25164=CARTESIAN_POINT('Ctrl Pts',(-1.77018771684844,1.,0.1662793551464));
#25165=CARTESIAN_POINT('Ctrl Pts',(-1.75666056638427,-1.,0.164834765707158));
#25166=CARTESIAN_POINT('Ctrl Pts',(-1.75666056638427,1.,0.164834765707158));
#25167=CARTESIAN_POINT('Ctrl Pts',(-1.7472034950333,-1.,0.163814161002002));
#25168=CARTESIAN_POINT('Ctrl Pts',(-1.7472034950333,1.,0.163814161002002));
#25169=CARTESIAN_POINT('Ctrl Pts',(-1.74236521665491,-1.,0.163289472382896));
#25170=CARTESIAN_POINT('Ctrl Pts',(-1.74236521665491,1.,0.163289472382896));
#25171=CARTESIAN_POINT('',(-2.19890268624765,1.,0.069476445021958));
#25172=CARTESIAN_POINT('Ctrl Pts',(-2.19890268624765,1.,0.069476445021958));
#25173=CARTESIAN_POINT('Ctrl Pts',(-2.19777582085423,1.,0.0701143536325489));
#25174=CARTESIAN_POINT('Ctrl Pts',(-2.19552129484002,1.,0.0713863779526153));
#25175=CARTESIAN_POINT('Ctrl Pts',(-2.19213712013662,1.,0.0732830357306724));
#25176=CARTESIAN_POINT('Ctrl Pts',(-2.1876201139953,1.,0.0757891465836146));
#25177=CARTESIAN_POINT('Ctrl Pts',(-2.18196589448887,1.,0.0788837727685241));
#25178=CARTESIAN_POINT('Ctrl Pts',(-2.176303712113,1.,0.0819402680872764));
#25179=CARTESIAN_POINT('Ctrl Pts',(-2.17063357870952,1.,0.0849584620835371));
#25180=CARTESIAN_POINT('Ctrl Pts',(-2.16495552645014,1.,0.0879381291386921));
#25181=CARTESIAN_POINT('Ctrl Pts',(-2.15926961544516,1.,0.0908789888107264));
#25182=CARTESIAN_POINT('Ctrl Pts',(-2.1535759397817,1.,0.0937807218867642));
#25183=CARTESIAN_POINT('Ctrl Pts',(-2.14787463531795,1.,0.0966429852305457));
#25184=CARTESIAN_POINT('Ctrl Pts',(-2.14216588396025,1.,0.0994654261990914));
#25185=CARTESIAN_POINT('Ctrl Pts',(-2.13644992667165,1.,0.1022477005561));
#25186=CARTESIAN_POINT('Ctrl Pts',(-2.13072704887293,1.,0.104989479152739));
#25187=CARTESIAN_POINT('Ctrl Pts',(-2.12499752307,1.,0.10769043523109));
#25188=CARTESIAN_POINT('Ctrl Pts',(-2.11926155590865,1.,0.110350236135025));
#25189=CARTESIAN_POINT('Ctrl Pts',(-2.11351924490306,1.,0.112968534419737));
#25190=CARTESIAN_POINT('Ctrl Pts',(-2.10777050261309,1.,0.115544957687926));
#25191=CARTESIAN_POINT('Ctrl Pts',(-2.102015121329,1.,0.118079107988355));
#25192=CARTESIAN_POINT('Ctrl Pts',(-2.0962529286773,1.,0.120570567965122));
#25193=CARTESIAN_POINT('Ctrl Pts',(-2.09048392424825,1.,0.123018905621083));
#25194=CARTESIAN_POINT('Ctrl Pts',(-2.08470840653643,1.,0.125423679412061));
#25195=CARTESIAN_POINT('Ctrl Pts',(-2.07892715110987,1.,0.12778444527612));
#25196=CARTESIAN_POINT('Ctrl Pts',(-2.07314114713063,1.,0.130100748328403));
#25197=CARTESIAN_POINT('Ctrl Pts',(-2.06735123910326,1.,0.13237211154771));
#25198=CARTESIAN_POINT('Ctrl Pts',(-2.06155781517842,1.,0.134598026192106));
#25199=CARTESIAN_POINT('Ctrl Pts',(-2.05576044414264,1.,0.136777941218043));
#25200=CARTESIAN_POINT('Ctrl Pts',(-2.04995762001328,1.,0.138911255368966));
#25201=CARTESIAN_POINT('Ctrl Pts',(-2.04414757947916,1.,0.140997332152546));
#25202=CARTESIAN_POINT('Ctrl Pts',(-2.03832911025912,1.,0.143035515058209));
#25203=CARTESIAN_POINT('Ctrl Pts',(-2.03250223739942,1.,0.145025140186057));
#25204=CARTESIAN_POINT('Ctrl Pts',(-2.02666926182017,1.,0.146965557332583));
#25205=CARTESIAN_POINT('Ctrl Pts',(-2.02083464969894,1.,0.148856124775337));
#25206=CARTESIAN_POINT('Ctrl Pts',(-2.01500291940238,1.,0.150696157673078));
#25207=CARTESIAN_POINT('Ctrl Pts',(-2.00917680318424,1.,0.15248488362145));
#25208=CARTESIAN_POINT('Ctrl Pts',(-2.00335565310543,1.,0.154221403049722));
#25209=CARTESIAN_POINT('Ctrl Pts',(-1.99753284771497,1.,0.155904629548783));
#25210=CARTESIAN_POINT('Ctrl Pts',(-1.99169810931908,1.,0.157533331459227));
#25211=CARTESIAN_POINT('Ctrl Pts',(-1.98584238283292,1.,0.159106226437299));
#25212=CARTESIAN_POINT('Ctrl Pts',(-1.97996195437559,1.,0.160622060784611));
#25213=CARTESIAN_POINT('Ctrl Pts',(-1.97406280235188,1.,0.162079693556288));
#25214=CARTESIAN_POINT('Ctrl Pts',(-1.96816512677967,1.,0.163478185457734));
#25215=CARTESIAN_POINT('Ctrl Pts',(-1.96229379940136,1.,0.164816568920269));
#25216=CARTESIAN_POINT('Ctrl Pts',(-1.9564675971873,1.,0.166093592002812));
#25217=CARTESIAN_POINT('Ctrl Pts',(-1.95069027794294,1.,0.167307501784475));
#25218=CARTESIAN_POINT('Ctrl Pts',(-1.94493757756931,1.,0.168455741607556));
#25219=CARTESIAN_POINT('Ctrl Pts',(-1.93915639211581,1.,0.169534904817491));
#25220=CARTESIAN_POINT('Ctrl Pts',(-1.93329183155539,1.,0.170541253116201));
#25221=CARTESIAN_POINT('Ctrl Pts',(-1.92731093582036,1.,0.171471191532988));
#25222=CARTESIAN_POINT('Ctrl Pts',(-1.9212233439798,1.,0.172321621259514));
#25223=CARTESIAN_POINT('Ctrl Pts',(-1.91511429159527,1.,0.173090695383496));
#25224=CARTESIAN_POINT('Ctrl Pts',(-1.90911693975267,1.,0.173776635257817));
#25225=CARTESIAN_POINT('Ctrl Pts',(-1.90335253862834,1.,0.174375518661085));
#25226=CARTESIAN_POINT('Ctrl Pts',(-1.89788101117132,1.,0.174879405091263));
#25227=CARTESIAN_POINT('Ctrl Pts',(-1.892646301985,1.,0.175274276190844));
#25228=CARTESIAN_POINT('Ctrl Pts',(-1.88742606273259,1.,0.175538155840648));
#25229=CARTESIAN_POINT('Ctrl Pts',(-1.88188663145367,1.,0.175644148889698));
#25230=CARTESIAN_POINT('Ctrl Pts',(-1.87563767773588,1.,0.175563480746485));
#25231=CARTESIAN_POINT('Ctrl Pts',(-1.86828349694799,1.,0.175268337590758));
#25232=CARTESIAN_POINT('Ctrl Pts',(-1.85948367088837,1.,0.17473525927603));
#25233=CARTESIAN_POINT('Ctrl Pts',(-1.8489811319852,1.,0.173946627587731));
#25234=CARTESIAN_POINT('Ctrl Pts',(-1.83658380527692,1.,0.1728894428919));
#25235=CARTESIAN_POINT('Ctrl Pts',(-1.82215766811545,1.,0.171554770204119));
#25236=CARTESIAN_POINT('Ctrl Pts',(-1.80561530629706,1.,0.169936923904608));
#25237=CARTESIAN_POINT('Ctrl Pts',(-1.7869064998507,1.,0.168032772805197));
#25238=CARTESIAN_POINT('Ctrl Pts',(-1.77018771684844,1.,0.1662793551464));
#25239=CARTESIAN_POINT('Ctrl Pts',(-1.75666056638427,1.,0.164834765707158));
#25240=CARTESIAN_POINT('Ctrl Pts',(-1.7472034950333,1.,0.163814161002002));
#25241=CARTESIAN_POINT('Ctrl Pts',(-1.74236521665491,1.,0.163289472382896));
#25242=CARTESIAN_POINT('',(-2.19890268624765,0.,0.069476445021958));
#25243=CARTESIAN_POINT('Origin',(-2.19890268624765,0.,-0.0694764450219585));
#25244=CARTESIAN_POINT('',(-2.19890268624765,1.,-0.0694764450219585));
#25245=CARTESIAN_POINT('',(-2.19890268624765,1.,0.069476445021958));
#25246=CARTESIAN_POINT('',(-2.19890268624765,0.,-0.0694764450219585));
#25247=CARTESIAN_POINT('Ctrl Pts',(-1.74236521665491,-1.,-0.163289472382896));
#25248=CARTESIAN_POINT('Ctrl Pts',(-1.74236521665491,1.,-0.163289472382896));
#25249=CARTESIAN_POINT('Ctrl Pts',(-1.74720349503904,-1.,-0.163814161002474));
#25250=CARTESIAN_POINT('Ctrl Pts',(-1.74720349503904,1.,-0.163814161002474));
#25251=CARTESIAN_POINT('Ctrl Pts',(-1.75666056640041,-1.,-0.164834765708484));
#25252=CARTESIAN_POINT('Ctrl Pts',(-1.75666056640041,1.,-0.164834765708484));
#25253=CARTESIAN_POINT('Ctrl Pts',(-1.77018771687692,-1.,-0.166279355148738));
#25254=CARTESIAN_POINT('Ctrl Pts',(-1.77018771687692,1.,-0.166279355148738));
#25255=CARTESIAN_POINT('Ctrl Pts',(-1.78690649988931,-1.,-0.16803277280837));
#25256=CARTESIAN_POINT('Ctrl Pts',(-1.78690649988931,1.,-0.16803277280837));
#25257=CARTESIAN_POINT('Ctrl Pts',(-1.80561530633924,-1.,-0.169936923908078));
#25258=CARTESIAN_POINT('Ctrl Pts',(-1.80561530633924,1.,-0.169936923908078));
#25259=CARTESIAN_POINT('Ctrl Pts',(-1.82215766815414,-1.,-0.171554770207306));
#25260=CARTESIAN_POINT('Ctrl Pts',(-1.82215766815414,1.,-0.171554770207306));
#25261=CARTESIAN_POINT('Ctrl Pts',(-1.83658380530747,-1.,-0.17288944289442));
#25262=CARTESIAN_POINT('Ctrl Pts',(-1.83658380530747,1.,-0.17288944289442));
#25263=CARTESIAN_POINT('Ctrl Pts',(-1.84898113200543,-1.,-0.173946627589401));
#25264=CARTESIAN_POINT('Ctrl Pts',(-1.84898113200543,1.,-0.173946627589401));
#25265=CARTESIAN_POINT('Ctrl Pts',(-1.85948367089838,-1.,-0.174735259276856));
#25266=CARTESIAN_POINT('Ctrl Pts',(-1.85948367089838,1.,-0.174735259276856));
#25267=CARTESIAN_POINT('Ctrl Pts',(-1.86828349694972,-1.,-0.175268337590901));
#25268=CARTESIAN_POINT('Ctrl Pts',(-1.86828349694972,1.,-0.175268337590901));
#25269=CARTESIAN_POINT('Ctrl Pts',(-1.87563767773249,-1.,-0.175563480746205));
#25270=CARTESIAN_POINT('Ctrl Pts',(-1.87563767773249,1.,-0.175563480746205));
#25271=CARTESIAN_POINT('Ctrl Pts',(-1.88188663144846,-1.,-0.175644148889271));
#25272=CARTESIAN_POINT('Ctrl Pts',(-1.88188663144846,1.,-0.175644148889271));
#25273=CARTESIAN_POINT('Ctrl Pts',(-1.88742606272818,-1.,-0.175538155840286));
#25274=CARTESIAN_POINT('Ctrl Pts',(-1.88742606272818,1.,-0.175538155840286));
#25275=CARTESIAN_POINT('Ctrl Pts',(-1.89264630198279,-1.,-0.175274276190664));
#25276=CARTESIAN_POINT('Ctrl Pts',(-1.89264630198279,1.,-0.175274276190664));
#25277=CARTESIAN_POINT('Ctrl Pts',(-1.89788101117148,-1.,-0.174879405091277));
#25278=CARTESIAN_POINT('Ctrl Pts',(-1.89788101117148,1.,-0.174879405091277));
#25279=CARTESIAN_POINT('Ctrl Pts',(-1.90335253863003,-1.,-0.174375518661222));
#25280=CARTESIAN_POINT('Ctrl Pts',(-1.90335253863003,1.,-0.174375518661222));
#25281=CARTESIAN_POINT('Ctrl Pts',(-1.90911693975475,-1.,-0.173776635257984));
#25282=CARTESIAN_POINT('Ctrl Pts',(-1.90911693975475,1.,-0.173776635257984));
#25283=CARTESIAN_POINT('Ctrl Pts',(-1.91511429159681,-1.,-0.173090695383619));
#25284=CARTESIAN_POINT('Ctrl Pts',(-1.91511429159681,1.,-0.173090695383619));
#25285=CARTESIAN_POINT('Ctrl Pts',(-1.92122334398034,-1.,-0.172321621259557));
#25286=CARTESIAN_POINT('Ctrl Pts',(-1.92122334398034,1.,-0.172321621259557));
#25287=CARTESIAN_POINT('Ctrl Pts',(-1.92731093582,-1.,-0.17147119153296));
#25288=CARTESIAN_POINT('Ctrl Pts',(-1.92731093582,1.,-0.17147119153296));
#25289=CARTESIAN_POINT('Ctrl Pts',(-1.93329183155455,-1.,-0.170541253116136));
#25290=CARTESIAN_POINT('Ctrl Pts',(-1.93329183155455,1.,-0.170541253116136));
#25291=CARTESIAN_POINT('Ctrl Pts',(-1.93915639211497,-1.,-0.169534904817425));
#25292=CARTESIAN_POINT('Ctrl Pts',(-1.93915639211497,1.,-0.169534904817425));
#25293=CARTESIAN_POINT('Ctrl Pts',(-1.94493757756879,-1.,-0.168455741607516));
#25294=CARTESIAN_POINT('Ctrl Pts',(-1.94493757756879,1.,-0.168455741607516));
#25295=CARTESIAN_POINT('Ctrl Pts',(-1.95069027794286,-1.,-0.167307501784469));
#25296=CARTESIAN_POINT('Ctrl Pts',(-1.95069027794286,1.,-0.167307501784469));
#25297=CARTESIAN_POINT('Ctrl Pts',(-1.95646759718755,-1.,-0.166093592002833));
#25298=CARTESIAN_POINT('Ctrl Pts',(-1.95646759718755,1.,-0.166093592002833));
#25299=CARTESIAN_POINT('Ctrl Pts',(-1.96229379940174,-1.,-0.1648165689203));
#25300=CARTESIAN_POINT('Ctrl Pts',(-1.96229379940174,1.,-0.1648165689203));
#25301=CARTESIAN_POINT('Ctrl Pts',(-1.96816512678,-1.,-0.16347818545776));
#25302=CARTESIAN_POINT('Ctrl Pts',(-1.96816512678,1.,-0.16347818545776));
#25303=CARTESIAN_POINT('Ctrl Pts',(-1.97406280235204,-1.,-0.162079693556302));
#25304=CARTESIAN_POINT('Ctrl Pts',(-1.97406280235204,1.,-0.162079693556302));
#25305=CARTESIAN_POINT('Ctrl Pts',(-1.97996195437557,-1.,-0.16062206078461));
#25306=CARTESIAN_POINT('Ctrl Pts',(-1.97996195437557,1.,-0.16062206078461));
#25307=CARTESIAN_POINT('Ctrl Pts',(-1.98584238283279,-1.,-0.159106226437289));
#25308=CARTESIAN_POINT('Ctrl Pts',(-1.98584238283279,1.,-0.159106226437289));
#25309=CARTESIAN_POINT('Ctrl Pts',(-1.99169810931893,-1.,-0.157533331459215));
#25310=CARTESIAN_POINT('Ctrl Pts',(-1.99169810931893,1.,-0.157533331459215));
#25311=CARTESIAN_POINT('Ctrl Pts',(-1.99753284771487,-1.,-0.155904629548775));
#25312=CARTESIAN_POINT('Ctrl Pts',(-1.99753284771487,1.,-0.155904629548775));
#25313=CARTESIAN_POINT('Ctrl Pts',(-2.00335565310539,-1.,-0.154221403049719));
#25314=CARTESIAN_POINT('Ctrl Pts',(-2.00335565310539,1.,-0.154221403049719));
#25315=CARTESIAN_POINT('Ctrl Pts',(-2.00917680318426,-1.,-0.152484883621452));
#25316=CARTESIAN_POINT('Ctrl Pts',(-2.00917680318426,1.,-0.152484883621452));
#25317=CARTESIAN_POINT('Ctrl Pts',(-2.01500291940243,-1.,-0.150696157673084));
#25318=CARTESIAN_POINT('Ctrl Pts',(-2.01500291940243,1.,-0.150696157673084));
#25319=CARTESIAN_POINT('Ctrl Pts',(-2.02083464969897,-1.,-0.148856124775343));
#25320=CARTESIAN_POINT('Ctrl Pts',(-2.02083464969897,1.,-0.148856124775343));
#25321=CARTESIAN_POINT('Ctrl Pts',(-2.02666926182017,-1.,-0.146965557332586));
#25322=CARTESIAN_POINT('Ctrl Pts',(-2.02666926182017,1.,-0.146965557332586));
#25323=CARTESIAN_POINT('Ctrl Pts',(-2.03250223739941,-1.,-0.145025140186058));
#25324=CARTESIAN_POINT('Ctrl Pts',(-2.03250223739941,1.,-0.145025140186058));
#25325=CARTESIAN_POINT('Ctrl Pts',(-2.03832911025913,-1.,-0.143035515058208));
#25326=CARTESIAN_POINT('Ctrl Pts',(-2.03832911025913,1.,-0.143035515058208));
#25327=CARTESIAN_POINT('Ctrl Pts',(-2.04414757947919,-1.,-0.140997332152545));
#25328=CARTESIAN_POINT('Ctrl Pts',(-2.04414757947919,1.,-0.140997332152545));
#25329=CARTESIAN_POINT('Ctrl Pts',(-2.04995762001333,-1.,-0.138911255368966));
#25330=CARTESIAN_POINT('Ctrl Pts',(-2.04995762001333,1.,-0.138911255368966));
#25331=CARTESIAN_POINT('Ctrl Pts',(-2.0557604441427,-1.,-0.136777941218044));
#25332=CARTESIAN_POINT('Ctrl Pts',(-2.0557604441427,1.,-0.136777941218044));
#25333=CARTESIAN_POINT('Ctrl Pts',(-2.06155781517844,-1.,-0.134598026192107));
#25334=CARTESIAN_POINT('Ctrl Pts',(-2.06155781517844,1.,-0.134598026192107));
#25335=CARTESIAN_POINT('Ctrl Pts',(-2.06735123910319,-1.,-0.13237211154771));
#25336=CARTESIAN_POINT('Ctrl Pts',(-2.06735123910319,1.,-0.13237211154771));
#25337=CARTESIAN_POINT('Ctrl Pts',(-2.07314114713047,-1.,-0.130100748328401));
#25338=CARTESIAN_POINT('Ctrl Pts',(-2.07314114713047,1.,-0.130100748328401));
#25339=CARTESIAN_POINT('Ctrl Pts',(-2.07892715110967,-1.,-0.127784445276116));
#25340=CARTESIAN_POINT('Ctrl Pts',(-2.07892715110967,1.,-0.127784445276116));
#25341=CARTESIAN_POINT('Ctrl Pts',(-2.08470840653628,-1.,-0.125423679412058));
#25342=CARTESIAN_POINT('Ctrl Pts',(-2.08470840653628,1.,-0.125423679412058));
#25343=CARTESIAN_POINT('Ctrl Pts',(-2.09048392424826,-1.,-0.123018905621083));
#25344=CARTESIAN_POINT('Ctrl Pts',(-2.09048392424826,1.,-0.123018905621083));
#25345=CARTESIAN_POINT('Ctrl Pts',(-2.09625292867756,-1.,-0.120570567965129));
#25346=CARTESIAN_POINT('Ctrl Pts',(-2.09625292867756,1.,-0.120570567965129));
#25347=CARTESIAN_POINT('Ctrl Pts',(-2.10201512132945,-1.,-0.118079107988368));
#25348=CARTESIAN_POINT('Ctrl Pts',(-2.10201512132945,1.,-0.118079107988368));
#25349=CARTESIAN_POINT('Ctrl Pts',(-2.10777050261359,-1.,-0.11554495768794));
#25350=CARTESIAN_POINT('Ctrl Pts',(-2.10777050261359,1.,-0.11554495768794));
#25351=CARTESIAN_POINT('Ctrl Pts',(-2.11351924490335,-1.,-0.112968534419746));
#25352=CARTESIAN_POINT('Ctrl Pts',(-2.11351924490335,1.,-0.112968534419746));
#25353=CARTESIAN_POINT('Ctrl Pts',(-2.11926155590849,-1.,-0.11035023613502));
#25354=CARTESIAN_POINT('Ctrl Pts',(-2.11926155590849,1.,-0.11035023613502));
#25355=CARTESIAN_POINT('Ctrl Pts',(-2.12499752306927,-1.,-0.107690435231068));
#25356=CARTESIAN_POINT('Ctrl Pts',(-2.12499752306927,1.,-0.107690435231068));
#25357=CARTESIAN_POINT('Ctrl Pts',(-2.1307270488718,-1.,-0.104989479152703));
#25358=CARTESIAN_POINT('Ctrl Pts',(-2.1307270488718,1.,-0.104989479152703));
#25359=CARTESIAN_POINT('Ctrl Pts',(-2.13644992667052,-1.,-0.102247700556064));
#25360=CARTESIAN_POINT('Ctrl Pts',(-2.13644992667052,1.,-0.102247700556064));
#25361=CARTESIAN_POINT('Ctrl Pts',(-2.14216588395974,-1.,-0.0994654261990744));
#25362=CARTESIAN_POINT('Ctrl Pts',(-2.14216588395974,1.,-0.0994654261990744));
#25363=CARTESIAN_POINT('Ctrl Pts',(-2.14787463531864,-1.,-0.096642985230569));
#25364=CARTESIAN_POINT('Ctrl Pts',(-2.14787463531864,1.,-0.096642985230569));
#25365=CARTESIAN_POINT('Ctrl Pts',(-2.15357593978377,-1.,-0.0937807218868346));
#25366=CARTESIAN_POINT('Ctrl Pts',(-2.15357593978377,1.,-0.0937807218868346));
#25367=CARTESIAN_POINT('Ctrl Pts',(-2.15926961544808,-1.,-0.0908789888108267));
#25368=CARTESIAN_POINT('Ctrl Pts',(-2.15926961544808,1.,-0.0908789888108267));
#25369=CARTESIAN_POINT('Ctrl Pts',(-2.16495552645275,-1.,-0.0879381291387824));
#25370=CARTESIAN_POINT('Ctrl Pts',(-2.16495552645275,1.,-0.0879381291387824));
#25371=CARTESIAN_POINT('Ctrl Pts',(-2.17063357871031,-1.,-0.0849584620835644));
#25372=CARTESIAN_POINT('Ctrl Pts',(-2.17063357871031,1.,-0.0849584620835644));
#25373=CARTESIAN_POINT('Ctrl Pts',(-2.1763037121106,-1.,-0.0819402680871941));
#25374=CARTESIAN_POINT('Ctrl Pts',(-2.1763037121106,1.,-0.0819402680871941));
#25375=CARTESIAN_POINT('Ctrl Pts',(-2.18196589448304,-1.,-0.0788837727683229));
#25376=CARTESIAN_POINT('Ctrl Pts',(-2.18196589448304,1.,-0.0788837727683229));
#25377=CARTESIAN_POINT('Ctrl Pts',(-2.1876201139874,-1.,-0.0757891465833413));
#25378=CARTESIAN_POINT('Ctrl Pts',(-2.1876201139874,1.,-0.0757891465833413));
#25379=CARTESIAN_POINT('Ctrl Pts',(-2.19213712012956,-1.,-0.0732830357304277));
#25380=CARTESIAN_POINT('Ctrl Pts',(-2.19213712012956,1.,-0.0732830357304277));
#25381=CARTESIAN_POINT('Ctrl Pts',(-2.19552129483562,-1.,-0.0713863779524629));
#25382=CARTESIAN_POINT('Ctrl Pts',(-2.19552129483562,1.,-0.0713863779524629));
#25383=CARTESIAN_POINT('Ctrl Pts',(-2.19777582085261,-1.,-0.0701143536324927));
#25384=CARTESIAN_POINT('Ctrl Pts',(-2.19777582085261,1.,-0.0701143536324927));
#25385=CARTESIAN_POINT('Ctrl Pts',(-2.19890268624765,-1.,-0.0694764450219585));
#25386=CARTESIAN_POINT('Ctrl Pts',(-2.19890268624765,1.,-0.0694764450219585));
#25387=CARTESIAN_POINT('',(-1.74236521665491,1.,-0.163289472382896));
#25388=CARTESIAN_POINT('Ctrl Pts',(-1.74236521665491,1.,-0.163289472382896));
#25389=CARTESIAN_POINT('Ctrl Pts',(-1.74720349503904,1.,-0.163814161002474));
#25390=CARTESIAN_POINT('Ctrl Pts',(-1.75666056640041,1.,-0.164834765708484));
#25391=CARTESIAN_POINT('Ctrl Pts',(-1.77018771687692,1.,-0.166279355148738));
#25392=CARTESIAN_POINT('Ctrl Pts',(-1.78690649988931,1.,-0.16803277280837));
#25393=CARTESIAN_POINT('Ctrl Pts',(-1.80561530633924,1.,-0.169936923908078));
#25394=CARTESIAN_POINT('Ctrl Pts',(-1.82215766815414,1.,-0.171554770207306));
#25395=CARTESIAN_POINT('Ctrl Pts',(-1.83658380530747,1.,-0.17288944289442));
#25396=CARTESIAN_POINT('Ctrl Pts',(-1.84898113200543,1.,-0.173946627589401));
#25397=CARTESIAN_POINT('Ctrl Pts',(-1.85948367089838,1.,-0.174735259276856));
#25398=CARTESIAN_POINT('Ctrl Pts',(-1.86828349694972,1.,-0.175268337590901));
#25399=CARTESIAN_POINT('Ctrl Pts',(-1.87563767773249,1.,-0.175563480746205));
#25400=CARTESIAN_POINT('Ctrl Pts',(-1.88188663144846,1.,-0.175644148889271));
#25401=CARTESIAN_POINT('Ctrl Pts',(-1.88742606272818,1.,-0.175538155840286));
#25402=CARTESIAN_POINT('Ctrl Pts',(-1.89264630198279,1.,-0.175274276190664));
#25403=CARTESIAN_POINT('Ctrl Pts',(-1.89788101117148,1.,-0.174879405091277));
#25404=CARTESIAN_POINT('Ctrl Pts',(-1.90335253863003,1.,-0.174375518661222));
#25405=CARTESIAN_POINT('Ctrl Pts',(-1.90911693975475,1.,-0.173776635257984));
#25406=CARTESIAN_POINT('Ctrl Pts',(-1.91511429159681,1.,-0.173090695383619));
#25407=CARTESIAN_POINT('Ctrl Pts',(-1.92122334398034,1.,-0.172321621259557));
#25408=CARTESIAN_POINT('Ctrl Pts',(-1.92731093582,1.,-0.17147119153296));
#25409=CARTESIAN_POINT('Ctrl Pts',(-1.93329183155455,1.,-0.170541253116136));
#25410=CARTESIAN_POINT('Ctrl Pts',(-1.93915639211497,1.,-0.169534904817425));
#25411=CARTESIAN_POINT('Ctrl Pts',(-1.94493757756879,1.,-0.168455741607516));
#25412=CARTESIAN_POINT('Ctrl Pts',(-1.95069027794286,1.,-0.167307501784469));
#25413=CARTESIAN_POINT('Ctrl Pts',(-1.95646759718755,1.,-0.166093592002833));
#25414=CARTESIAN_POINT('Ctrl Pts',(-1.96229379940174,1.,-0.1648165689203));
#25415=CARTESIAN_POINT('Ctrl Pts',(-1.96816512678,1.,-0.16347818545776));
#25416=CARTESIAN_POINT('Ctrl Pts',(-1.97406280235204,1.,-0.162079693556302));
#25417=CARTESIAN_POINT('Ctrl Pts',(-1.97996195437557,1.,-0.16062206078461));
#25418=CARTESIAN_POINT('Ctrl Pts',(-1.98584238283279,1.,-0.159106226437289));
#25419=CARTESIAN_POINT('Ctrl Pts',(-1.99169810931893,1.,-0.157533331459215));
#25420=CARTESIAN_POINT('Ctrl Pts',(-1.99753284771487,1.,-0.155904629548775));
#25421=CARTESIAN_POINT('Ctrl Pts',(-2.00335565310539,1.,-0.154221403049719));
#25422=CARTESIAN_POINT('Ctrl Pts',(-2.00917680318426,1.,-0.152484883621452));
#25423=CARTESIAN_POINT('Ctrl Pts',(-2.01500291940243,1.,-0.150696157673084));
#25424=CARTESIAN_POINT('Ctrl Pts',(-2.02083464969897,1.,-0.148856124775343));
#25425=CARTESIAN_POINT('Ctrl Pts',(-2.02666926182017,1.,-0.146965557332586));
#25426=CARTESIAN_POINT('Ctrl Pts',(-2.03250223739941,1.,-0.145025140186058));
#25427=CARTESIAN_POINT('Ctrl Pts',(-2.03832911025913,1.,-0.143035515058208));
#25428=CARTESIAN_POINT('Ctrl Pts',(-2.04414757947919,1.,-0.140997332152545));
#25429=CARTESIAN_POINT('Ctrl Pts',(-2.04995762001333,1.,-0.138911255368966));
#25430=CARTESIAN_POINT('Ctrl Pts',(-2.0557604441427,1.,-0.136777941218044));
#25431=CARTESIAN_POINT('Ctrl Pts',(-2.06155781517844,1.,-0.134598026192107));
#25432=CARTESIAN_POINT('Ctrl Pts',(-2.06735123910319,1.,-0.13237211154771));
#25433=CARTESIAN_POINT('Ctrl Pts',(-2.07314114713047,1.,-0.130100748328401));
#25434=CARTESIAN_POINT('Ctrl Pts',(-2.07892715110967,1.,-0.127784445276116));
#25435=CARTESIAN_POINT('Ctrl Pts',(-2.08470840653628,1.,-0.125423679412058));
#25436=CARTESIAN_POINT('Ctrl Pts',(-2.09048392424826,1.,-0.123018905621083));
#25437=CARTESIAN_POINT('Ctrl Pts',(-2.09625292867756,1.,-0.120570567965129));
#25438=CARTESIAN_POINT('Ctrl Pts',(-2.10201512132945,1.,-0.118079107988368));
#25439=CARTESIAN_POINT('Ctrl Pts',(-2.10777050261359,1.,-0.11554495768794));
#25440=CARTESIAN_POINT('Ctrl Pts',(-2.11351924490335,1.,-0.112968534419746));
#25441=CARTESIAN_POINT('Ctrl Pts',(-2.11926155590849,1.,-0.11035023613502));
#25442=CARTESIAN_POINT('Ctrl Pts',(-2.12499752306927,1.,-0.107690435231068));
#25443=CARTESIAN_POINT('Ctrl Pts',(-2.1307270488718,1.,-0.104989479152703));
#25444=CARTESIAN_POINT('Ctrl Pts',(-2.13644992667052,1.,-0.102247700556064));
#25445=CARTESIAN_POINT('Ctrl Pts',(-2.14216588395974,1.,-0.0994654261990744));
#25446=CARTESIAN_POINT('Ctrl Pts',(-2.14787463531864,1.,-0.096642985230569));
#25447=CARTESIAN_POINT('Ctrl Pts',(-2.15357593978377,1.,-0.0937807218868346));
#25448=CARTESIAN_POINT('Ctrl Pts',(-2.15926961544808,1.,-0.0908789888108267));
#25449=CARTESIAN_POINT('Ctrl Pts',(-2.16495552645275,1.,-0.0879381291387824));
#25450=CARTESIAN_POINT('Ctrl Pts',(-2.17063357871031,1.,-0.0849584620835644));
#25451=CARTESIAN_POINT('Ctrl Pts',(-2.1763037121106,1.,-0.0819402680871941));
#25452=CARTESIAN_POINT('Ctrl Pts',(-2.18196589448304,1.,-0.0788837727683229));
#25453=CARTESIAN_POINT('Ctrl Pts',(-2.1876201139874,1.,-0.0757891465833413));
#25454=CARTESIAN_POINT('Ctrl Pts',(-2.19213712012956,1.,-0.0732830357304277));
#25455=CARTESIAN_POINT('Ctrl Pts',(-2.19552129483562,1.,-0.0713863779524629));
#25456=CARTESIAN_POINT('Ctrl Pts',(-2.19777582085261,1.,-0.0701143536324927));
#25457=CARTESIAN_POINT('Ctrl Pts',(-2.19890268624765,1.,-0.0694764450219585));
#25458=CARTESIAN_POINT('',(-1.74236521665491,0.,-0.163289472382896));
#25459=CARTESIAN_POINT('Origin',(0.,0.,0.));
#25460=CARTESIAN_POINT('',(-1.7075470150345,1.,-0.383122945602004));
#25461=CARTESIAN_POINT('Origin',(0.,1.,0.));
#25462=CARTESIAN_POINT('',(-1.7075470150345,0.,-0.383122945602004));
#25463=CARTESIAN_POINT('Ctrl Pts',(-2.11275013067528,-1.,-0.61342227326009));
#25464=CARTESIAN_POINT('Ctrl Pts',(-2.11275013067528,1.,-0.61342227326009));
#25465=CARTESIAN_POINT('Ctrl Pts',(-2.11187554260142,-1.,-0.61246736556225));
#25466=CARTESIAN_POINT('Ctrl Pts',(-2.11187554260142,1.,-0.61246736556225));
#25467=CARTESIAN_POINT('Ctrl Pts',(-2.11012443807661,-1.,-0.610560911691113));
#25468=CARTESIAN_POINT('Ctrl Pts',(-2.11012443807661,1.,-0.610560911691113));
#25469=CARTESIAN_POINT('Ctrl Pts',(-2.10749199615859,-1.,-0.607711315456826));
#25470=CARTESIAN_POINT('Ctrl Pts',(-2.10749199615859,1.,-0.607711315456826));
#25471=CARTESIAN_POINT('Ctrl Pts',(-2.10397049887709,-1.,-0.603932030738212));
#25472=CARTESIAN_POINT('Ctrl Pts',(-2.10397049887709,1.,-0.603932030738212));
#25473=CARTESIAN_POINT('Ctrl Pts',(-2.09954930865331,-1.,-0.599241616422144));
#25474=CARTESIAN_POINT('Ctrl Pts',(-2.09954930865331,1.,-0.599241616422144));
#25475=CARTESIAN_POINT('Ctrl Pts',(-2.09510876220501,-1.,-0.594585006052823));
#25476=CARTESIAN_POINT('Ctrl Pts',(-2.09510876220501,1.,-0.594585006052823));
#25477=CARTESIAN_POINT('Ctrl Pts',(-2.09064881812053,-1.,-0.589962365403189));
#25478=CARTESIAN_POINT('Ctrl Pts',(-2.09064881812053,1.,-0.589962365403189));
#25479=CARTESIAN_POINT('Ctrl Pts',(-2.086169437277,-1.,-0.585373918990895));
#25480=CARTESIAN_POINT('Ctrl Pts',(-2.086169437277,1.,-0.585373918990895));
#25481=CARTESIAN_POINT('Ctrl Pts',(-2.08167059018138,-1.,-0.580819952107257));
#25482=CARTESIAN_POINT('Ctrl Pts',(-2.08167059018138,1.,-0.580819952107257));
#25483=CARTESIAN_POINT('Ctrl Pts',(-2.07715226767361,-1.,-0.576300797416274));
#25484=CARTESIAN_POINT('Ctrl Pts',(-2.07715226767361,1.,-0.576300797416274));
#25485=CARTESIAN_POINT('Ctrl Pts',(-2.07261449292757,-1.,-0.571816823242411));
#25486=CARTESIAN_POINT('Ctrl Pts',(-2.07261449292757,1.,-0.571816823242411));
#25487=CARTESIAN_POINT('Ctrl Pts',(-2.06805732997383,-1.,-0.567368421181229));
#25488=CARTESIAN_POINT('Ctrl Pts',(-2.06805732997383,1.,-0.567368421181229));
#25489=CARTESIAN_POINT('Ctrl Pts',(-2.06348090160697,-1.,-0.562955993082574));
#25490=CARTESIAN_POINT('Ctrl Pts',(-2.06348090160697,1.,-0.562955993082574));
#25491=CARTESIAN_POINT('Ctrl Pts',(-2.05888537756571,-1.,-0.558579940185467));
#25492=CARTESIAN_POINT('Ctrl Pts',(-2.05888537756571,1.,-0.558579940185467));
#25493=CARTESIAN_POINT('Ctrl Pts',(-2.05427091604482,-1.,-0.554240657464109));
#25494=CARTESIAN_POINT('Ctrl Pts',(-2.05427091604482,1.,-0.554240657464109));
#25495=CARTESIAN_POINT('Ctrl Pts',(-2.04963761077974,-1.,-0.549938525150342));
#25496=CARTESIAN_POINT('Ctrl Pts',(-2.04963761077974,1.,-0.549938525150342));
#25497=CARTESIAN_POINT('Ctrl Pts',(-2.0449854471456,-1.,-0.545673903817348));
#25498=CARTESIAN_POINT('Ctrl Pts',(-2.0449854471456,1.,-0.545673903817348));
#25499=CARTESIAN_POINT('Ctrl Pts',(-2.0403142269048,-1.,-0.54144712061552));
#25500=CARTESIAN_POINT('Ctrl Pts',(-2.0403142269048,1.,-0.54144712061552));
#25501=CARTESIAN_POINT('Ctrl Pts',(-2.03562362953993,-1.,-0.537258489833134));
#25502=CARTESIAN_POINT('Ctrl Pts',(-2.03562362953993,1.,-0.537258489833134));
#25503=CARTESIAN_POINT('Ctrl Pts',(-2.03091336214401,-1.,-0.533108355132905));
#25504=CARTESIAN_POINT('Ctrl Pts',(-2.03091336214401,1.,-0.533108355132905));
#25505=CARTESIAN_POINT('Ctrl Pts',(-2.02618329083289,-1.,-0.52899712724191));
#25506=CARTESIAN_POINT('Ctrl Pts',(-2.02618329083289,1.,-0.52899712724191));
#25507=CARTESIAN_POINT('Ctrl Pts',(-2.02143356304712,-1.,-0.524925318333518));
#25508=CARTESIAN_POINT('Ctrl Pts',(-2.02143356304712,1.,-0.524925318333518));
#25509=CARTESIAN_POINT('Ctrl Pts',(-2.01666477917305,-1.,-0.520893590399428));
#25510=CARTESIAN_POINT('Ctrl Pts',(-2.01666477917305,1.,-0.520893590399428));
#25511=CARTESIAN_POINT('Ctrl Pts',(-2.01187773939257,-1.,-0.516902681728733));
#25512=CARTESIAN_POINT('Ctrl Pts',(-2.01187773939257,1.,-0.516902681728733));
#25513=CARTESIAN_POINT('Ctrl Pts',(-2.00707309946955,-1.,-0.512953306961813));
#25514=CARTESIAN_POINT('Ctrl Pts',(-2.00707309946955,1.,-0.512953306961813));
#25515=CARTESIAN_POINT('Ctrl Pts',(-2.00225107134733,-1.,-0.509046069886152));
#25516=CARTESIAN_POINT('Ctrl Pts',(-2.00225107134733,1.,-0.509046069886152));
#25517=CARTESIAN_POINT('Ctrl Pts',(-1.99741107463567,-1.,-0.505181361323011));
#25518=CARTESIAN_POINT('Ctrl Pts',(-1.99741107463567,1.,-0.505181361323011));
#25519=CARTESIAN_POINT('Ctrl Pts',(-1.9925514912615,-1.,-0.501359287727129));
#25520=CARTESIAN_POINT('Ctrl Pts',(-1.9925514912615,1.,-0.501359287727129));
#25521=CARTESIAN_POINT('Ctrl Pts',(-1.98767044752929,-1.,-0.497579909545564));
#25522=CARTESIAN_POINT('Ctrl Pts',(-1.98767044752929,1.,-0.497579909545564));
#25523=CARTESIAN_POINT('Ctrl Pts',(-1.9827665876182,-1.,-0.493843476541492));
#25524=CARTESIAN_POINT('Ctrl Pts',(-1.9827665876182,1.,-0.493843476541492));
#25525=CARTESIAN_POINT('Ctrl Pts',(-1.97783973019229,-1.,-0.490150627860955));
#25526=CARTESIAN_POINT('Ctrl Pts',(-1.97783973019229,1.,-0.490150627860955));
#25527=CARTESIAN_POINT('Ctrl Pts',(-1.97289186263272,-1.,-0.486502692907661));
#25528=CARTESIAN_POINT('Ctrl Pts',(-1.97289186263272,1.,-0.486502692907661));
#25529=CARTESIAN_POINT('Ctrl Pts',(-1.96792703422358,-1.,-0.482901662120686));
#25530=CARTESIAN_POINT('Ctrl Pts',(-1.96792703422358,1.,-0.482901662120686));
#25531=CARTESIAN_POINT('Ctrl Pts',(-1.96294933055938,-1.,-0.479349583074846));
#25532=CARTESIAN_POINT('Ctrl Pts',(-1.96294933055938,1.,-0.479349583074846));
#25533=CARTESIAN_POINT('Ctrl Pts',(-1.95796111148175,-1.,-0.475848034683171));
#25534=CARTESIAN_POINT('Ctrl Pts',(-1.95796111148175,1.,-0.475848034683171));
#25535=CARTESIAN_POINT('Ctrl Pts',(-1.95296148278136,-1.,-0.472397672264079));
#25536=CARTESIAN_POINT('Ctrl Pts',(-1.95296148278136,1.,-0.472397672264079));
#25537=CARTESIAN_POINT('Ctrl Pts',(-1.94794381136524,-1.,-0.468997482913158));
#25538=CARTESIAN_POINT('Ctrl Pts',(-1.94794381136524,1.,-0.468997482913158));
#25539=CARTESIAN_POINT('Ctrl Pts',(-1.94289794196205,-1.,-0.465645462026064));
#25540=CARTESIAN_POINT('Ctrl Pts',(-1.94289794196205,1.,-0.465645462026064));
#25541=CARTESIAN_POINT('Ctrl Pts',(-1.93781486640834,-1.,-0.462340031009087));
#25542=CARTESIAN_POINT('Ctrl Pts',(-1.93781486640834,1.,-0.462340031009087));
#25543=CARTESIAN_POINT('Ctrl Pts',(-1.93269066517936,-1.,-0.459081234547931));
#25544=CARTESIAN_POINT('Ctrl Pts',(-1.93269066517936,1.,-0.459081234547931));
#25545=CARTESIAN_POINT('Ctrl Pts',(-1.92753067150461,-1.,-0.455872005174335));
#25546=CARTESIAN_POINT('Ctrl Pts',(-1.92753067150461,1.,-0.455872005174335));
#25547=CARTESIAN_POINT('Ctrl Pts',(-1.9223538064847,-1.,-0.452719478359356));
#25548=CARTESIAN_POINT('Ctrl Pts',(-1.9223538064847,1.,-0.452719478359356));
#25549=CARTESIAN_POINT('Ctrl Pts',(-1.91718342555717,-1.,-0.449632260106572));
#25550=CARTESIAN_POINT('Ctrl Pts',(-1.91718342555717,1.,-0.449632260106572));
#25551=CARTESIAN_POINT('Ctrl Pts',(-1.91203699981095,-1.,-0.446617343485651));
#25552=CARTESIAN_POINT('Ctrl Pts',(-1.91203699981095,1.,-0.446617343485651));
#25553=CARTESIAN_POINT('Ctrl Pts',(-1.90691756144906,-1.,-0.44367755684917));
#25554=CARTESIAN_POINT('Ctrl Pts',(-1.90691756144906,1.,-0.44367755684917));
#25555=CARTESIAN_POINT('Ctrl Pts',(-1.90180124389137,-1.,-0.44080783370416));
#25556=CARTESIAN_POINT('Ctrl Pts',(-1.90180124389137,1.,-0.44080783370416));
#25557=CARTESIAN_POINT('Ctrl Pts',(-1.89663648956549,-1.,-0.437995003948443));
#25558=CARTESIAN_POINT('Ctrl Pts',(-1.89663648956549,1.,-0.437995003948443));
#25559=CARTESIAN_POINT('Ctrl Pts',(-1.89136993975585,-1.,-0.43522566096358));
#25560=CARTESIAN_POINT('Ctrl Pts',(-1.89136993975585,1.,-0.43522566096358));
#25561=CARTESIAN_POINT('Ctrl Pts',(-1.88596913666828,-1.,-0.432493038548833));
#25562=CARTESIAN_POINT('Ctrl Pts',(-1.88596913666828,1.,-0.432493038548833));
#25563=CARTESIAN_POINT('Ctrl Pts',(-1.88044229001778,-1.,-0.429803062482217));
#25564=CARTESIAN_POINT('Ctrl Pts',(-1.88044229001778,1.,-0.429803062482217));
#25565=CARTESIAN_POINT('Ctrl Pts',(-1.87486989291333,-1.,-0.427183828518743));
#25566=CARTESIAN_POINT('Ctrl Pts',(-1.87486989291333,1.,-0.427183828518743));
#25567=CARTESIAN_POINT('Ctrl Pts',(-1.8693780394412,-1.,-0.424678177290876));
#25568=CARTESIAN_POINT('Ctrl Pts',(-1.8693780394412,1.,-0.424678177290876));
#25569=CARTESIAN_POINT('Ctrl Pts',(-1.86408083333863,-1.,-0.422327307417884));
#25570=CARTESIAN_POINT('Ctrl Pts',(-1.86408083333863,1.,-0.422327307417884));
#25571=CARTESIAN_POINT('Ctrl Pts',(-1.8590328109667,-1.,-0.420157287975583));
#25572=CARTESIAN_POINT('Ctrl Pts',(-1.8590328109667,1.,-0.420157287975583));
#25573=CARTESIAN_POINT('Ctrl Pts',(-1.8541763285645,-1.,-0.418164129144045));
#25574=CARTESIAN_POINT('Ctrl Pts',(-1.8541763285645,1.,-0.418164129144045));
#25575=CARTESIAN_POINT('Ctrl Pts',(-1.84929312930314,-1.,-0.416300022039885));
#25576=CARTESIAN_POINT('Ctrl Pts',(-1.84929312930314,1.,-0.416300022039885));
#25577=CARTESIAN_POINT('Ctrl Pts',(-1.84405757074218,-1.,-0.414487438255542));
#25578=CARTESIAN_POINT('Ctrl Pts',(-1.84405757074218,1.,-0.414487438255542));
#25579=CARTESIAN_POINT('Ctrl Pts',(-1.8380895347617,-1.,-0.412633125322945));
#25580=CARTESIAN_POINT('Ctrl Pts',(-1.8380895347617,1.,-0.412633125322945));
#25581=CARTESIAN_POINT('Ctrl Pts',(-1.83100408895047,-1.,-0.410641256301276));
#25582=CARTESIAN_POINT('Ctrl Pts',(-1.83100408895047,1.,-0.410641256301276));
#25583=CARTESIAN_POINT('Ctrl Pts',(-1.82247022677562,-1.,-0.408428948106227));
#25584=CARTESIAN_POINT('Ctrl Pts',(-1.82247022677562,1.,-0.408428948106227));
#25585=CARTESIAN_POINT('Ctrl Pts',(-1.81223801812013,-1.,-0.405933518407175));
#25586=CARTESIAN_POINT('Ctrl Pts',(-1.81223801812013,1.,-0.405933518407175));
#25587=CARTESIAN_POINT('Ctrl Pts',(-1.80012077173238,-1.,-0.403107976163396));
#25588=CARTESIAN_POINT('Ctrl Pts',(-1.80012077173238,1.,-0.403107976163396));
#25589=CARTESIAN_POINT('Ctrl Pts',(-1.78598826343754,-1.,-0.399919403774155));
#25590=CARTESIAN_POINT('Ctrl Pts',(-1.78598826343754,1.,-0.399919403774155));
#25591=CARTESIAN_POINT('Ctrl Pts',(-1.76975560043442,-1.,-0.396346196110688));
#25592=CARTESIAN_POINT('Ctrl Pts',(-1.76975560043442,1.,-0.396346196110688));
#25593=CARTESIAN_POINT('Ctrl Pts',(-1.75137405310193,-1.,-0.392375812285395));
#25594=CARTESIAN_POINT('Ctrl Pts',(-1.75137405310193,1.,-0.392375812285395));
#25595=CARTESIAN_POINT('Ctrl Pts',(-1.73493170972829,-1.,-0.388877023502615));
#25596=CARTESIAN_POINT('Ctrl Pts',(-1.73493170972829,1.,-0.388877023502615));
#25597=CARTESIAN_POINT('Ctrl Pts',(-1.72162022244582,-1.,-0.386070790323281));
#25598=CARTESIAN_POINT('Ctrl Pts',(-1.72162022244582,1.,-0.386070790323281));
#25599=CARTESIAN_POINT('Ctrl Pts',(-1.71231062891398,-1.,-0.384119047314215));
#25600=CARTESIAN_POINT('Ctrl Pts',(-1.71231062891398,1.,-0.384119047314215));
#25601=CARTESIAN_POINT('Ctrl Pts',(-1.7075470150345,-1.,-0.383122945602004));
#25602=CARTESIAN_POINT('Ctrl Pts',(-1.7075470150345,1.,-0.383122945602004));
#25603=CARTESIAN_POINT('',(-2.11275013067528,1.,-0.61342227326009));
#25604=CARTESIAN_POINT('Ctrl Pts',(-2.11275013067528,1.,-0.61342227326009));
#25605=CARTESIAN_POINT('Ctrl Pts',(-2.11187554260142,1.,-0.61246736556225));
#25606=CARTESIAN_POINT('Ctrl Pts',(-2.11012443807661,1.,-0.610560911691113));
#25607=CARTESIAN_POINT('Ctrl Pts',(-2.10749199615859,1.,-0.607711315456826));
#25608=CARTESIAN_POINT('Ctrl Pts',(-2.10397049887709,1.,-0.603932030738212));
#25609=CARTESIAN_POINT('Ctrl Pts',(-2.09954930865331,1.,-0.599241616422144));
#25610=CARTESIAN_POINT('Ctrl Pts',(-2.09510876220501,1.,-0.594585006052823));
#25611=CARTESIAN_POINT('Ctrl Pts',(-2.09064881812053,1.,-0.589962365403189));
#25612=CARTESIAN_POINT('Ctrl Pts',(-2.086169437277,1.,-0.585373918990895));
#25613=CARTESIAN_POINT('Ctrl Pts',(-2.08167059018138,1.,-0.580819952107257));
#25614=CARTESIAN_POINT('Ctrl Pts',(-2.07715226767361,1.,-0.576300797416274));
#25615=CARTESIAN_POINT('Ctrl Pts',(-2.07261449292757,1.,-0.571816823242411));
#25616=CARTESIAN_POINT('Ctrl Pts',(-2.06805732997383,1.,-0.567368421181229));
#25617=CARTESIAN_POINT('Ctrl Pts',(-2.06348090160697,1.,-0.562955993082574));
#25618=CARTESIAN_POINT('Ctrl Pts',(-2.05888537756571,1.,-0.558579940185467));
#25619=CARTESIAN_POINT('Ctrl Pts',(-2.05427091604482,1.,-0.554240657464109));
#25620=CARTESIAN_POINT('Ctrl Pts',(-2.04963761077974,1.,-0.549938525150342));
#25621=CARTESIAN_POINT('Ctrl Pts',(-2.0449854471456,1.,-0.545673903817348));
#25622=CARTESIAN_POINT('Ctrl Pts',(-2.0403142269048,1.,-0.54144712061552));
#25623=CARTESIAN_POINT('Ctrl Pts',(-2.03562362953993,1.,-0.537258489833134));
#25624=CARTESIAN_POINT('Ctrl Pts',(-2.03091336214401,1.,-0.533108355132905));
#25625=CARTESIAN_POINT('Ctrl Pts',(-2.02618329083289,1.,-0.52899712724191));
#25626=CARTESIAN_POINT('Ctrl Pts',(-2.02143356304712,1.,-0.524925318333518));
#25627=CARTESIAN_POINT('Ctrl Pts',(-2.01666477917305,1.,-0.520893590399428));
#25628=CARTESIAN_POINT('Ctrl Pts',(-2.01187773939257,1.,-0.516902681728733));
#25629=CARTESIAN_POINT('Ctrl Pts',(-2.00707309946955,1.,-0.512953306961813));
#25630=CARTESIAN_POINT('Ctrl Pts',(-2.00225107134733,1.,-0.509046069886152));
#25631=CARTESIAN_POINT('Ctrl Pts',(-1.99741107463567,1.,-0.505181361323011));
#25632=CARTESIAN_POINT('Ctrl Pts',(-1.9925514912615,1.,-0.501359287727129));
#25633=CARTESIAN_POINT('Ctrl Pts',(-1.98767044752929,1.,-0.497579909545564));
#25634=CARTESIAN_POINT('Ctrl Pts',(-1.9827665876182,1.,-0.493843476541492));
#25635=CARTESIAN_POINT('Ctrl Pts',(-1.97783973019229,1.,-0.490150627860955));
#25636=CARTESIAN_POINT('Ctrl Pts',(-1.97289186263272,1.,-0.486502692907661));
#25637=CARTESIAN_POINT('Ctrl Pts',(-1.96792703422358,1.,-0.482901662120686));
#25638=CARTESIAN_POINT('Ctrl Pts',(-1.96294933055938,1.,-0.479349583074846));
#25639=CARTESIAN_POINT('Ctrl Pts',(-1.95796111148175,1.,-0.475848034683171));
#25640=CARTESIAN_POINT('Ctrl Pts',(-1.95296148278136,1.,-0.472397672264079));
#25641=CARTESIAN_POINT('Ctrl Pts',(-1.94794381136524,1.,-0.468997482913158));
#25642=CARTESIAN_POINT('Ctrl Pts',(-1.94289794196205,1.,-0.465645462026064));
#25643=CARTESIAN_POINT('Ctrl Pts',(-1.93781486640834,1.,-0.462340031009087));
#25644=CARTESIAN_POINT('Ctrl Pts',(-1.93269066517936,1.,-0.459081234547931));
#25645=CARTESIAN_POINT('Ctrl Pts',(-1.92753067150461,1.,-0.455872005174335));
#25646=CARTESIAN_POINT('Ctrl Pts',(-1.9223538064847,1.,-0.452719478359356));
#25647=CARTESIAN_POINT('Ctrl Pts',(-1.91718342555717,1.,-0.449632260106572));
#25648=CARTESIAN_POINT('Ctrl Pts',(-1.91203699981095,1.,-0.446617343485651));
#25649=CARTESIAN_POINT('Ctrl Pts',(-1.90691756144906,1.,-0.44367755684917));
#25650=CARTESIAN_POINT('Ctrl Pts',(-1.90180124389137,1.,-0.44080783370416));
#25651=CARTESIAN_POINT('Ctrl Pts',(-1.89663648956549,1.,-0.437995003948443));
#25652=CARTESIAN_POINT('Ctrl Pts',(-1.89136993975585,1.,-0.43522566096358));
#25653=CARTESIAN_POINT('Ctrl Pts',(-1.88596913666828,1.,-0.432493038548833));
#25654=CARTESIAN_POINT('Ctrl Pts',(-1.88044229001778,1.,-0.429803062482217));
#25655=CARTESIAN_POINT('Ctrl Pts',(-1.87486989291333,1.,-0.427183828518743));
#25656=CARTESIAN_POINT('Ctrl Pts',(-1.8693780394412,1.,-0.424678177290876));
#25657=CARTESIAN_POINT('Ctrl Pts',(-1.86408083333863,1.,-0.422327307417884));
#25658=CARTESIAN_POINT('Ctrl Pts',(-1.8590328109667,1.,-0.420157287975583));
#25659=CARTESIAN_POINT('Ctrl Pts',(-1.8541763285645,1.,-0.418164129144045));
#25660=CARTESIAN_POINT('Ctrl Pts',(-1.84929312930314,1.,-0.416300022039885));
#25661=CARTESIAN_POINT('Ctrl Pts',(-1.84405757074218,1.,-0.414487438255542));
#25662=CARTESIAN_POINT('Ctrl Pts',(-1.8380895347617,1.,-0.412633125322945));
#25663=CARTESIAN_POINT('Ctrl Pts',(-1.83100408895047,1.,-0.410641256301276));
#25664=CARTESIAN_POINT('Ctrl Pts',(-1.82247022677562,1.,-0.408428948106227));
#25665=CARTESIAN_POINT('Ctrl Pts',(-1.81223801812013,1.,-0.405933518407175));
#25666=CARTESIAN_POINT('Ctrl Pts',(-1.80012077173238,1.,-0.403107976163396));
#25667=CARTESIAN_POINT('Ctrl Pts',(-1.78598826343754,1.,-0.399919403774155));
#25668=CARTESIAN_POINT('Ctrl Pts',(-1.76975560043442,1.,-0.396346196110688));
#25669=CARTESIAN_POINT('Ctrl Pts',(-1.75137405310193,1.,-0.392375812285395));
#25670=CARTESIAN_POINT('Ctrl Pts',(-1.73493170972829,1.,-0.388877023502615));
#25671=CARTESIAN_POINT('Ctrl Pts',(-1.72162022244582,1.,-0.386070790323281));
#25672=CARTESIAN_POINT('Ctrl Pts',(-1.71231062891398,1.,-0.384119047314215));
#25673=CARTESIAN_POINT('Ctrl Pts',(-1.7075470150345,1.,-0.383122945602004));
#25674=CARTESIAN_POINT('',(-2.11275013067528,0.,-0.61342227326009));
#25675=CARTESIAN_POINT('Origin',(-2.0698113262342,0.,-0.745574324794401));
#25676=CARTESIAN_POINT('',(-2.0698113262342,1.,-0.745574324794401));
#25677=CARTESIAN_POINT('',(-2.11275013067528,1.,-0.61342227326009));
#25678=CARTESIAN_POINT('',(-2.0698113262342,0.,-0.745574324794401));
#25679=CARTESIAN_POINT('Ctrl Pts',(-1.60662857109684,-1.,-0.693717979106306));
#25680=CARTESIAN_POINT('Ctrl Pts',(-1.60662857109684,1.,-0.693717979106306));
#25681=CARTESIAN_POINT('Ctrl Pts',(-1.61106790958151,-1.,-0.695712097881194));
#25682=CARTESIAN_POINT('Ctrl Pts',(-1.61106790958151,1.,-0.695712097881194));
#25683=CARTESIAN_POINT('Ctrl Pts',(-1.61974673472612,-1.,-0.699605146405088));
#25684=CARTESIAN_POINT('Ctrl Pts',(-1.61974673472612,1.,-0.699605146405088));
#25685=CARTESIAN_POINT('Ctrl Pts',(-1.63216541664676,-1.,-0.705159151988319));
#25686=CARTESIAN_POINT('Ctrl Pts',(-1.63216541664676,1.,-0.705159151988319));
#25687=CARTESIAN_POINT('Ctrl Pts',(-1.64752408832016,-1.,-0.711993139355394));
#25688=CARTESIAN_POINT('Ctrl Pts',(-1.64752408832016,1.,-0.711993139355394));
#25689=CARTESIAN_POINT('Ctrl Pts',(-1.6647288055568,-1.,-0.719585433804282));
#25690=CARTESIAN_POINT('Ctrl Pts',(-1.6647288055568,1.,-0.719585433804282));
#25691=CARTESIAN_POINT('Ctrl Pts',(-1.67996158455503,-1.,-0.726235967997433));
#25692=CARTESIAN_POINT('Ctrl Pts',(-1.67996158455503,1.,-0.726235967997433));
#25693=CARTESIAN_POINT('Ctrl Pts',(-1.69326921975743,-1.,-0.731963238697195));
#25694=CARTESIAN_POINT('Ctrl Pts',(-1.69326921975743,1.,-0.731963238697195));
#25695=CARTESIAN_POINT('Ctrl Pts',(-1.70473309006121,-1.,-0.736799665724771));
#25696=CARTESIAN_POINT('Ctrl Pts',(-1.70473309006121,1.,-0.736799665724771));
#25697=CARTESIAN_POINT('Ctrl Pts',(-1.71447789751927,-1.,-0.740795162032087));
#25698=CARTESIAN_POINT('Ctrl Pts',(-1.71447789751927,1.,-0.740795162032087));
#25699=CARTESIAN_POINT('Ctrl Pts',(-1.7226822991693,-1.,-0.744021445433764));
#25700=CARTESIAN_POINT('Ctrl Pts',(-1.7226822991693,1.,-0.744021445433764));
#25701=CARTESIAN_POINT('Ctrl Pts',(-1.72958533647399,-1.,-0.746574710096436));
#25702=CARTESIAN_POINT('Ctrl Pts',(-1.72958533647399,1.,-0.746574710096436));
#25703=CARTESIAN_POINT('Ctrl Pts',(-1.73550351679848,-1.,-0.748582462954854));
#25704=CARTESIAN_POINT('Ctrl Pts',(-1.73550351679848,1.,-0.748582462954854));
#25705=CARTESIAN_POINT('Ctrl Pts',(-1.74080458266705,-1.,-0.75019343597954));
#25706=CARTESIAN_POINT('Ctrl Pts',(-1.74080458266705,1.,-0.75019343597954));
#25707=CARTESIAN_POINT('Ctrl Pts',(-1.74585086852298,-1.,-0.751555614163629));
#25708=CARTESIAN_POINT('Ctrl Pts',(-1.74585086852298,1.,-0.751555614163629));
#25709=CARTESIAN_POINT('Ctrl Pts',(-1.75095139468809,-1.,-0.752797683531377));
#25710=CARTESIAN_POINT('Ctrl Pts',(-1.75095139468809,1.,-0.752797683531377));
#25711=CARTESIAN_POINT('Ctrl Pts',(-1.75631083600175,-1.,-0.75400925402848));
#25712=CARTESIAN_POINT('Ctrl Pts',(-1.75631083600175,1.,-0.75400925402848));
#25713=CARTESIAN_POINT('Ctrl Pts',(-1.7619781724032,-1.,-0.755220979975262));
#25714=CARTESIAN_POINT('Ctrl Pts',(-1.7619781724032,1.,-0.755220979975262));
#25715=CARTESIAN_POINT('Ctrl Pts',(-1.76789396003141,-1.,-0.756421896028403));
#25716=CARTESIAN_POINT('Ctrl Pts',(-1.76789396003141,1.,-0.756421896028403));
#25717=CARTESIAN_POINT('Ctrl Pts',(-1.77394167108342,-1.,-0.757578264077238));
#25718=CARTESIAN_POINT('Ctrl Pts',(-1.77394167108342,1.,-0.757578264077238));
#25719=CARTESIAN_POINT('Ctrl Pts',(-1.77999411220912,-1.,-0.75865062667738));
#25720=CARTESIAN_POINT('Ctrl Pts',(-1.77999411220912,1.,-0.75865062667738));
#25721=CARTESIAN_POINT('Ctrl Pts',(-1.78596964884526,-1.,-0.759614401109868));
#25722=CARTESIAN_POINT('Ctrl Pts',(-1.78596964884526,1.,-0.759614401109868));
#25723=CARTESIAN_POINT('Ctrl Pts',(-1.79185815610802,-1.,-0.760469555880425));
#25724=CARTESIAN_POINT('Ctrl Pts',(-1.79185815610802,1.,-0.760469555880425));
#25725=CARTESIAN_POINT('Ctrl Pts',(-1.79768986997735,-1.,-0.761229695230359));
#25726=CARTESIAN_POINT('Ctrl Pts',(-1.79768986997735,1.,-0.761229695230359));
#25727=CARTESIAN_POINT('Ctrl Pts',(-1.80351583877334,-1.,-0.761915336443515));
#25728=CARTESIAN_POINT('Ctrl Pts',(-1.80351583877334,1.,-0.761915336443515));
#25729=CARTESIAN_POINT('Ctrl Pts',(-1.80938551463989,-1.,-0.762546129464036));
#25730=CARTESIAN_POINT('Ctrl Pts',(-1.80938551463989,1.,-0.762546129464036));
#25731=CARTESIAN_POINT('Ctrl Pts',(-1.81532118405566,-1.,-0.763132003836783));
#25732=CARTESIAN_POINT('Ctrl Pts',(-1.81532118405566,1.,-0.763132003836783));
#25733=CARTESIAN_POINT('Ctrl Pts',(-1.82131873145297,-1.,-0.763673465462854));
#25734=CARTESIAN_POINT('Ctrl Pts',(-1.82131873145297,1.,-0.763673465462854));
#25735=CARTESIAN_POINT('Ctrl Pts',(-1.8273599120008,-1.,-0.764165902606055));
#25736=CARTESIAN_POINT('Ctrl Pts',(-1.8273599120008,1.,-0.764165902606055));
#25737=CARTESIAN_POINT('Ctrl Pts',(-1.8334207722714,-1.,-0.764602549687845));
#25738=CARTESIAN_POINT('Ctrl Pts',(-1.8334207722714,1.,-0.764602549687845));
#25739=CARTESIAN_POINT('Ctrl Pts',(-1.83948181064823,-1.,-0.764978057881687));
#25740=CARTESIAN_POINT('Ctrl Pts',(-1.83948181064823,1.,-0.764978057881687));
#25741=CARTESIAN_POINT('Ctrl Pts',(-1.8455369887591,-1.,-0.765291664861971));
#25742=CARTESIAN_POINT('Ctrl Pts',(-1.8455369887591,1.,-0.765291664861971));
#25743=CARTESIAN_POINT('Ctrl Pts',(-1.85158945130054,-1.,-0.765545710619023));
#25744=CARTESIAN_POINT('Ctrl Pts',(-1.85158945130054,1.,-0.765545710619023));
#25745=CARTESIAN_POINT('Ctrl Pts',(-1.85764741390391,-1.,-0.765744212909305));
#25746=CARTESIAN_POINT('Ctrl Pts',(-1.85764741390391,1.,-0.765744212909305));
#25747=CARTESIAN_POINT('Ctrl Pts',(-1.86372027063314,-1.,-0.765891519092557));
#25748=CARTESIAN_POINT('Ctrl Pts',(-1.86372027063314,1.,-0.765891519092557));
#25749=CARTESIAN_POINT('Ctrl Pts',(-1.86981398314345,-1.,-0.765990708546111));
#25750=CARTESIAN_POINT('Ctrl Pts',(-1.86981398314345,1.,-0.765990708546111));
#25751=CARTESIAN_POINT('Ctrl Pts',(-1.87592888967886,-1.,-0.766042837036759));
#25752=CARTESIAN_POINT('Ctrl Pts',(-1.87592888967886,1.,-0.766042837036759));
#25753=CARTESIAN_POINT('Ctrl Pts',(-1.88206215302561,-1.,-0.766047794851868));
#25754=CARTESIAN_POINT('Ctrl Pts',(-1.88206215302561,1.,-0.766047794851868));
#25755=CARTESIAN_POINT('Ctrl Pts',(-1.88820926433409,-1.,-0.76600483706209));
#25756=CARTESIAN_POINT('Ctrl Pts',(-1.88820926433409,1.,-0.76600483706209));
#25757=CARTESIAN_POINT('Ctrl Pts',(-1.89436577771389,-1.,-0.765913193856979));
#25758=CARTESIAN_POINT('Ctrl Pts',(-1.89436577771389,1.,-0.765913193856979));
#25759=CARTESIAN_POINT('Ctrl Pts',(-1.90052930393599,-1.,-0.765772772593395));
#25760=CARTESIAN_POINT('Ctrl Pts',(-1.90052930393599,1.,-0.765772772593395));
#25761=CARTESIAN_POINT('Ctrl Pts',(-1.90669961402362,-1.,-0.765584196937936));
#25762=CARTESIAN_POINT('Ctrl Pts',(-1.90669961402362,1.,-0.765584196937936));
#25763=CARTESIAN_POINT('Ctrl Pts',(-1.91287765805174,-1.,-0.765348465884739));
#25764=CARTESIAN_POINT('Ctrl Pts',(-1.91287765805174,1.,-0.765348465884739));
#25765=CARTESIAN_POINT('Ctrl Pts',(-1.91906491634197,-1.,-0.765066729667095));
#25766=CARTESIAN_POINT('Ctrl Pts',(-1.91906491634197,1.,-0.765066729667095));
#25767=CARTESIAN_POINT('Ctrl Pts',(-1.92526263537041,-1.,-0.764740025488189));
#25768=CARTESIAN_POINT('Ctrl Pts',(-1.92526263537041,1.,-0.764740025488189));
#25769=CARTESIAN_POINT('Ctrl Pts',(-1.93147105496367,-1.,-0.764369010673889));
#25770=CARTESIAN_POINT('Ctrl Pts',(-1.93147105496367,1.,-0.764369010673889));
#25771=CARTESIAN_POINT('Ctrl Pts',(-1.93768964875867,-1.,-0.763954049121393));
#25772=CARTESIAN_POINT('Ctrl Pts',(-1.93768964875867,1.,-0.763954049121393));
#25773=CARTESIAN_POINT('Ctrl Pts',(-1.94391746617626,-1.,-0.76349533353858));
#25774=CARTESIAN_POINT('Ctrl Pts',(-1.94391746617626,1.,-0.76349533353858));
#25775=CARTESIAN_POINT('Ctrl Pts',(-1.95015342590025,-1.,-0.762992990878774));
#25776=CARTESIAN_POINT('Ctrl Pts',(-1.95015342590025,1.,-0.762992990878774));
#25777=CARTESIAN_POINT('Ctrl Pts',(-1.95639665309893,-1.,-0.762447203806263));
#25778=CARTESIAN_POINT('Ctrl Pts',(-1.95639665309893,1.,-0.762447203806263));
#25779=CARTESIAN_POINT('Ctrl Pts',(-1.96264672744229,-1.,-0.761858300014575));
#25780=CARTESIAN_POINT('Ctrl Pts',(-1.96264672744229,1.,-0.761858300014575));
#25781=CARTESIAN_POINT('Ctrl Pts',(-1.96890351582545,-1.,-0.761226690483986));
#25782=CARTESIAN_POINT('Ctrl Pts',(-1.96890351582545,1.,-0.761226690483986));
#25783=CARTESIAN_POINT('Ctrl Pts',(-1.97516705321521,-1.,-0.760552825409855));
#25784=CARTESIAN_POINT('Ctrl Pts',(-1.97516705321521,1.,-0.760552825409855));
#25785=CARTESIAN_POINT('Ctrl Pts',(-1.98143741418156,-1.,-0.759837147452135));
#25786=CARTESIAN_POINT('Ctrl Pts',(-1.98143741418156,1.,-0.759837147452135));
#25787=CARTESIAN_POINT('Ctrl Pts',(-1.98771456680806,-1.,-0.759080037802242));
#25788=CARTESIAN_POINT('Ctrl Pts',(-1.98771456680806,1.,-0.759080037802242));
#25789=CARTESIAN_POINT('Ctrl Pts',(-1.9939983109871,-1.,-0.758281796766377));
#25790=CARTESIAN_POINT('Ctrl Pts',(-1.9939983109871,1.,-0.758281796766377));
#25791=CARTESIAN_POINT('Ctrl Pts',(-2.00028834739072,-1.,-0.757442676862341));
#25792=CARTESIAN_POINT('Ctrl Pts',(-2.00028834739072,1.,-0.757442676862341));
#25793=CARTESIAN_POINT('Ctrl Pts',(-2.00658431587682,-1.,-0.756562904646496));
#25794=CARTESIAN_POINT('Ctrl Pts',(-2.00658431587682,1.,-0.756562904646496));
#25795=CARTESIAN_POINT('Ctrl Pts',(-2.01288584328149,-1.,-0.7556427049581));
#25796=CARTESIAN_POINT('Ctrl Pts',(-2.01288584328149,1.,-0.7556427049581));
#25797=CARTESIAN_POINT('Ctrl Pts',(-2.01919259406003,-1.,-0.75468233072352));
#25798=CARTESIAN_POINT('Ctrl Pts',(-2.01919259406003,1.,-0.75468233072352));
#25799=CARTESIAN_POINT('Ctrl Pts',(-2.02550428623587,-1.,-0.753682061113765));
#25800=CARTESIAN_POINT('Ctrl Pts',(-2.02550428623587,1.,-0.753682061113765));
#25801=CARTESIAN_POINT('Ctrl Pts',(-2.03182068456467,-1.,-0.752642180488104));
#25802=CARTESIAN_POINT('Ctrl Pts',(-2.03182068456467,1.,-0.752642180488104));
#25803=CARTESIAN_POINT('Ctrl Pts',(-2.03814160092173,-1.,-0.751562963361383));
#25804=CARTESIAN_POINT('Ctrl Pts',(-2.03814160092173,1.,-0.751562963361383));
#25805=CARTESIAN_POINT('Ctrl Pts',(-2.04446689147754,-1.,-0.750444657874758));
#25806=CARTESIAN_POINT('Ctrl Pts',(-2.04446689147754,1.,-0.750444657874758));
#25807=CARTESIAN_POINT('Ctrl Pts',(-2.05079645591606,-1.,-0.749287468663053));
#25808=CARTESIAN_POINT('Ctrl Pts',(-2.05079645591606,1.,-0.749287468663053));
#25809=CARTESIAN_POINT('Ctrl Pts',(-2.05713023030263,-1.,-0.748091554181101));
#25810=CARTESIAN_POINT('Ctrl Pts',(-2.05713023030263,1.,-0.748091554181101));
#25811=CARTESIAN_POINT('Ctrl Pts',(-2.06220058927162,-1.,-0.747103932785504));
#25812=CARTESIAN_POINT('Ctrl Pts',(-2.06220058927162,1.,-0.747103932785504));
#25813=CARTESIAN_POINT('Ctrl Pts',(-2.06600523016401,-1.,-0.746345871542695));
#25814=CARTESIAN_POINT('Ctrl Pts',(-2.06600523016401,1.,-0.746345871542695));
#25815=CARTESIAN_POINT('Ctrl Pts',(-2.06854248895575,-1.,-0.74583279137781));
#25816=CARTESIAN_POINT('Ctrl Pts',(-2.06854248895575,1.,-0.74583279137781));
#25817=CARTESIAN_POINT('Ctrl Pts',(-2.0698113262342,-1.,-0.745574324794401));
#25818=CARTESIAN_POINT('Ctrl Pts',(-2.0698113262342,1.,-0.745574324794401));
#25819=CARTESIAN_POINT('',(-1.60662857109684,1.,-0.693717979106306));
#25820=CARTESIAN_POINT('Ctrl Pts',(-1.60662857109684,1.,-0.693717979106306));
#25821=CARTESIAN_POINT('Ctrl Pts',(-1.61106790958151,1.,-0.695712097881194));
#25822=CARTESIAN_POINT('Ctrl Pts',(-1.61974673472612,1.,-0.699605146405088));
#25823=CARTESIAN_POINT('Ctrl Pts',(-1.63216541664676,1.,-0.705159151988319));
#25824=CARTESIAN_POINT('Ctrl Pts',(-1.64752408832016,1.,-0.711993139355394));
#25825=CARTESIAN_POINT('Ctrl Pts',(-1.6647288055568,1.,-0.719585433804282));
#25826=CARTESIAN_POINT('Ctrl Pts',(-1.67996158455503,1.,-0.726235967997433));
#25827=CARTESIAN_POINT('Ctrl Pts',(-1.69326921975743,1.,-0.731963238697195));
#25828=CARTESIAN_POINT('Ctrl Pts',(-1.70473309006121,1.,-0.736799665724771));
#25829=CARTESIAN_POINT('Ctrl Pts',(-1.71447789751927,1.,-0.740795162032087));
#25830=CARTESIAN_POINT('Ctrl Pts',(-1.7226822991693,1.,-0.744021445433764));
#25831=CARTESIAN_POINT('Ctrl Pts',(-1.72958533647399,1.,-0.746574710096436));
#25832=CARTESIAN_POINT('Ctrl Pts',(-1.73550351679848,1.,-0.748582462954854));
#25833=CARTESIAN_POINT('Ctrl Pts',(-1.74080458266705,1.,-0.75019343597954));
#25834=CARTESIAN_POINT('Ctrl Pts',(-1.74585086852298,1.,-0.751555614163629));
#25835=CARTESIAN_POINT('Ctrl Pts',(-1.75095139468809,1.,-0.752797683531377));
#25836=CARTESIAN_POINT('Ctrl Pts',(-1.75631083600175,1.,-0.75400925402848));
#25837=CARTESIAN_POINT('Ctrl Pts',(-1.7619781724032,1.,-0.755220979975262));
#25838=CARTESIAN_POINT('Ctrl Pts',(-1.76789396003141,1.,-0.756421896028403));
#25839=CARTESIAN_POINT('Ctrl Pts',(-1.77394167108342,1.,-0.757578264077238));
#25840=CARTESIAN_POINT('Ctrl Pts',(-1.77999411220912,1.,-0.75865062667738));
#25841=CARTESIAN_POINT('Ctrl Pts',(-1.78596964884526,1.,-0.759614401109868));
#25842=CARTESIAN_POINT('Ctrl Pts',(-1.79185815610802,1.,-0.760469555880425));
#25843=CARTESIAN_POINT('Ctrl Pts',(-1.79768986997735,1.,-0.761229695230359));
#25844=CARTESIAN_POINT('Ctrl Pts',(-1.80351583877334,1.,-0.761915336443515));
#25845=CARTESIAN_POINT('Ctrl Pts',(-1.80938551463989,1.,-0.762546129464036));
#25846=CARTESIAN_POINT('Ctrl Pts',(-1.81532118405566,1.,-0.763132003836783));
#25847=CARTESIAN_POINT('Ctrl Pts',(-1.82131873145297,1.,-0.763673465462854));
#25848=CARTESIAN_POINT('Ctrl Pts',(-1.8273599120008,1.,-0.764165902606055));
#25849=CARTESIAN_POINT('Ctrl Pts',(-1.8334207722714,1.,-0.764602549687845));
#25850=CARTESIAN_POINT('Ctrl Pts',(-1.83948181064823,1.,-0.764978057881687));
#25851=CARTESIAN_POINT('Ctrl Pts',(-1.8455369887591,1.,-0.765291664861971));
#25852=CARTESIAN_POINT('Ctrl Pts',(-1.85158945130054,1.,-0.765545710619023));
#25853=CARTESIAN_POINT('Ctrl Pts',(-1.85764741390391,1.,-0.765744212909305));
#25854=CARTESIAN_POINT('Ctrl Pts',(-1.86372027063314,1.,-0.765891519092557));
#25855=CARTESIAN_POINT('Ctrl Pts',(-1.86981398314345,1.,-0.765990708546111));
#25856=CARTESIAN_POINT('Ctrl Pts',(-1.87592888967886,1.,-0.766042837036759));
#25857=CARTESIAN_POINT('Ctrl Pts',(-1.88206215302561,1.,-0.766047794851868));
#25858=CARTESIAN_POINT('Ctrl Pts',(-1.88820926433409,1.,-0.76600483706209));
#25859=CARTESIAN_POINT('Ctrl Pts',(-1.89436577771389,1.,-0.765913193856979));
#25860=CARTESIAN_POINT('Ctrl Pts',(-1.90052930393599,1.,-0.765772772593395));
#25861=CARTESIAN_POINT('Ctrl Pts',(-1.90669961402362,1.,-0.765584196937936));
#25862=CARTESIAN_POINT('Ctrl Pts',(-1.91287765805174,1.,-0.765348465884739));
#25863=CARTESIAN_POINT('Ctrl Pts',(-1.91906491634197,1.,-0.765066729667095));
#25864=CARTESIAN_POINT('Ctrl Pts',(-1.92526263537041,1.,-0.764740025488189));
#25865=CARTESIAN_POINT('Ctrl Pts',(-1.93147105496367,1.,-0.764369010673889));
#25866=CARTESIAN_POINT('Ctrl Pts',(-1.93768964875867,1.,-0.763954049121393));
#25867=CARTESIAN_POINT('Ctrl Pts',(-1.94391746617626,1.,-0.76349533353858));
#25868=CARTESIAN_POINT('Ctrl Pts',(-1.95015342590025,1.,-0.762992990878774));
#25869=CARTESIAN_POINT('Ctrl Pts',(-1.95639665309893,1.,-0.762447203806263));
#25870=CARTESIAN_POINT('Ctrl Pts',(-1.96264672744229,1.,-0.761858300014575));
#25871=CARTESIAN_POINT('Ctrl Pts',(-1.96890351582545,1.,-0.761226690483986));
#25872=CARTESIAN_POINT('Ctrl Pts',(-1.97516705321521,1.,-0.760552825409855));
#25873=CARTESIAN_POINT('Ctrl Pts',(-1.98143741418156,1.,-0.759837147452135));
#25874=CARTESIAN_POINT('Ctrl Pts',(-1.98771456680806,1.,-0.759080037802242));
#25875=CARTESIAN_POINT('Ctrl Pts',(-1.9939983109871,1.,-0.758281796766377));
#25876=CARTESIAN_POINT('Ctrl Pts',(-2.00028834739072,1.,-0.757442676862341));
#25877=CARTESIAN_POINT('Ctrl Pts',(-2.00658431587682,1.,-0.756562904646496));
#25878=CARTESIAN_POINT('Ctrl Pts',(-2.01288584328149,1.,-0.7556427049581));
#25879=CARTESIAN_POINT('Ctrl Pts',(-2.01919259406003,1.,-0.75468233072352));
#25880=CARTESIAN_POINT('Ctrl Pts',(-2.02550428623587,1.,-0.753682061113765));
#25881=CARTESIAN_POINT('Ctrl Pts',(-2.03182068456467,1.,-0.752642180488104));
#25882=CARTESIAN_POINT('Ctrl Pts',(-2.03814160092173,1.,-0.751562963361383));
#25883=CARTESIAN_POINT('Ctrl Pts',(-2.04446689147754,1.,-0.750444657874758));
#25884=CARTESIAN_POINT('Ctrl Pts',(-2.05079645591606,1.,-0.749287468663053));
#25885=CARTESIAN_POINT('Ctrl Pts',(-2.05713023030263,1.,-0.748091554181101));
#25886=CARTESIAN_POINT('Ctrl Pts',(-2.06220058927162,1.,-0.747103932785504));
#25887=CARTESIAN_POINT('Ctrl Pts',(-2.06600523016401,1.,-0.746345871542695));
#25888=CARTESIAN_POINT('Ctrl Pts',(-2.06854248895575,1.,-0.74583279137781));
#25889=CARTESIAN_POINT('Ctrl Pts',(-2.0698113262342,1.,-0.745574324794401));
#25890=CARTESIAN_POINT('',(-1.60662857109684,0.,-0.693717979106306));
#25891=CARTESIAN_POINT('Origin',(0.,0.,0.));
#25892=CARTESIAN_POINT('',(-1.5055822144029,1.,-0.892032620296855));
#25893=CARTESIAN_POINT('Origin',(0.,1.,0.));
#25894=CARTESIAN_POINT('',(-1.5055822144029,0.,-0.892032620296855));
#25895=CARTESIAN_POINT('Ctrl Pts',(-1.81978687191668,-1.,-1.23627494547115));
#25896=CARTESIAN_POINT('Ctrl Pts',(-1.81978687191668,1.,-1.23627494547115));
#25897=CARTESIAN_POINT('Ctrl Pts',(-1.81925017193666,-1.,-1.23509651170476));
#25898=CARTESIAN_POINT('Ctrl Pts',(-1.81925017193666,1.,-1.23509651170476));
#25899=CARTESIAN_POINT('Ctrl Pts',(-1.81817389921279,-1.,-1.2327422452705));
#25900=CARTESIAN_POINT('Ctrl Pts',(-1.81817389921279,1.,-1.2327422452705));
#25901=CARTESIAN_POINT('Ctrl Pts',(-1.8165508718364,-1.,-1.2292186489137));
#25902=CARTESIAN_POINT('Ctrl Pts',(-1.8165508718364,1.,-1.2292186489137));
#25903=CARTESIAN_POINT('Ctrl Pts',(-1.81436959210434,-1.,-1.2245361330495));
#25904=CARTESIAN_POINT('Ctrl Pts',(-1.81436959210434,1.,-1.2245361330495));
#25905=CARTESIAN_POINT('Ctrl Pts',(-1.81161420806656,-1.,-1.21870906103557));
#25906=CARTESIAN_POINT('Ctrl Pts',(-1.81161420806656,1.,-1.21870906103557));
#25907=CARTESIAN_POINT('Ctrl Pts',(-1.80882996917129,-1.,-1.21290815708314));
#25908=CARTESIAN_POINT('Ctrl Pts',(-1.80882996917129,1.,-1.21290815708314));
#25909=CARTESIAN_POINT('Ctrl Pts',(-1.80601678480707,-1.,-1.20713356605475));
#25910=CARTESIAN_POINT('Ctrl Pts',(-1.80601678480707,1.,-1.20713356605475));
#25911=CARTESIAN_POINT('Ctrl Pts',(-1.80317454838603,-1.,-1.20138548938974));
#25912=CARTESIAN_POINT('Ctrl Pts',(-1.80317454838603,1.,-1.20138548938974));
#25913=CARTESIAN_POINT('Ctrl Pts',(-1.80030314369879,-1.,-1.19566418930242));
#25914=CARTESIAN_POINT('Ctrl Pts',(-1.80030314369879,1.,-1.19566418930242));
#25915=CARTESIAN_POINT('Ctrl Pts',(-1.79740245923478,-1.,-1.18996997934445));
#25916=CARTESIAN_POINT('Ctrl Pts',(-1.79740245923478,1.,-1.18996997934445));
#25917=CARTESIAN_POINT('Ctrl Pts',(-1.79447240321515,-1.,-1.18430321697432));
#25918=CARTESIAN_POINT('Ctrl Pts',(-1.79447240321515,1.,-1.18430321697432));
#25919=CARTESIAN_POINT('Ctrl Pts',(-1.79151291552689,-1.,-1.17866429440809));
#25920=CARTESIAN_POINT('Ctrl Pts',(-1.79151291552689,1.,-1.17866429440809));
#25921=CARTESIAN_POINT('Ctrl Pts',(-1.78852398877616,-1.,-1.17305363177328));
#25922=CARTESIAN_POINT('Ctrl Pts',(-1.78852398877616,1.,-1.17305363177328));
#25923=CARTESIAN_POINT('Ctrl Pts',(-1.78550566040443,-1.,-1.16747166312303));
#25924=CARTESIAN_POINT('Ctrl Pts',(-1.78550566040443,1.,-1.16747166312303));
#25925=CARTESIAN_POINT('Ctrl Pts',(-1.78245795881009,-1.,-1.16191881298499));
#25926=CARTESIAN_POINT('Ctrl Pts',(-1.78245795881009,1.,-1.16191881298499));
#25927=CARTESIAN_POINT('Ctrl Pts',(-1.77938085564275,-1.,-1.15639547194698));
#25928=CARTESIAN_POINT('Ctrl Pts',(-1.77938085564275,1.,-1.15639547194698));
#25929=CARTESIAN_POINT('Ctrl Pts',(-1.7762742255701,-1.,-1.15090197841515));
#25930=CARTESIAN_POINT('Ctrl Pts',(-1.7762742255701,1.,-1.15090197841515));
#25931=CARTESIAN_POINT('Ctrl Pts',(-1.77313777896194,-1.,-1.1454385822692));
#25932=CARTESIAN_POINT('Ctrl Pts',(-1.77313777896194,1.,-1.1454385822692));
#25933=CARTESIAN_POINT('Ctrl Pts',(-1.76997111386769,-1.,-1.14000548336975));
#25934=CARTESIAN_POINT('Ctrl Pts',(-1.76997111386769,1.,-1.14000548336975));
#25935=CARTESIAN_POINT('Ctrl Pts',(-1.76677384551862,-1.,-1.1346029180462));
#25936=CARTESIAN_POINT('Ctrl Pts',(-1.76677384551862,1.,-1.1346029180462));
#25937=CARTESIAN_POINT('Ctrl Pts',(-1.7635457196617,-1.,-1.12923123555075));
#25938=CARTESIAN_POINT('Ctrl Pts',(-1.7635457196617,1.,-1.12923123555075));
#25939=CARTESIAN_POINT('Ctrl Pts',(-1.76028671825096,-1.,-1.12389096855086));
#25940=CARTESIAN_POINT('Ctrl Pts',(-1.76028671825096,1.,-1.12389096855086));
#25941=CARTESIAN_POINT('Ctrl Pts',(-1.75699720772105,-1.,-1.11858293216763));
#25942=CARTESIAN_POINT('Ctrl Pts',(-1.75699720772105,1.,-1.11858293216763));
#25943=CARTESIAN_POINT('Ctrl Pts',(-1.7536777209463,-1.,-1.11330807582551));
#25944=CARTESIAN_POINT('Ctrl Pts',(-1.7536777209463,1.,-1.11330807582551));
#25945=CARTESIAN_POINT('Ctrl Pts',(-1.7503286607592,-1.,-1.10806728183007));
#25946=CARTESIAN_POINT('Ctrl Pts',(-1.7503286607592,1.,-1.10806728183007));
#25947=CARTESIAN_POINT('Ctrl Pts',(-1.74695004214923,-1.,-1.10286118991143));
#25948=CARTESIAN_POINT('Ctrl Pts',(-1.74695004214923,1.,-1.10286118991143));
#25949=CARTESIAN_POINT('Ctrl Pts',(-1.74354119236208,-1.,-1.09768999241225));
#25950=CARTESIAN_POINT('Ctrl Pts',(-1.74354119236208,1.,-1.09768999241225));
#25951=CARTESIAN_POINT('Ctrl Pts',(-1.74010053962247,-1.,-1.09255329056493));
#25952=CARTESIAN_POINT('Ctrl Pts',(-1.74010053962247,1.,-1.09255329056493));
#25953=CARTESIAN_POINT('Ctrl Pts',(-1.73662628326091,-1.,-1.08745056285427));
#25954=CARTESIAN_POINT('Ctrl Pts',(-1.73662628326091,1.,-1.08745056285427));
#25955=CARTESIAN_POINT('Ctrl Pts',(-1.73311705663407,-1.,-1.08238162784749));
#25956=CARTESIAN_POINT('Ctrl Pts',(-1.73311705663407,1.,-1.08238162784749));
#25957=CARTESIAN_POINT('Ctrl Pts',(-1.72957248977424,-1.,-1.0773470373727));
#25958=CARTESIAN_POINT('Ctrl Pts',(-1.72957248977424,1.,-1.0773470373727));
#25959=CARTESIAN_POINT('Ctrl Pts',(-1.72599406198488,-1.,-1.07234866990252));
#25960=CARTESIAN_POINT('Ctrl Pts',(-1.72599406198488,1.,-1.07234866990252));
#25961=CARTESIAN_POINT('Ctrl Pts',(-1.72238500928453,-1.,-1.06738966975462));
#25962=CARTESIAN_POINT('Ctrl Pts',(-1.72238500928453,1.,-1.06738966975462));
#25963=CARTESIAN_POINT('Ctrl Pts',(-1.71874858456904,-1.,-1.06247324680647));
#25964=CARTESIAN_POINT('Ctrl Pts',(-1.71874858456904,1.,-1.06247324680647));
#25965=CARTESIAN_POINT('Ctrl Pts',(-1.7150865442702,-1.,-1.05760163192479));
#25966=CARTESIAN_POINT('Ctrl Pts',(-1.7150865442702,1.,-1.05760163192479));
#25967=CARTESIAN_POINT('Ctrl Pts',(-1.71139783543989,-1.,-1.05277517202855));
#25968=CARTESIAN_POINT('Ctrl Pts',(-1.71139783543989,1.,-1.05277517202855));
#25969=CARTESIAN_POINT('Ctrl Pts',(-1.70767646263649,-1.,-1.04799085404995));
#25970=CARTESIAN_POINT('Ctrl Pts',(-1.70767646263649,1.,-1.04799085404995));
#25971=CARTESIAN_POINT('Ctrl Pts',(-1.70391338707982,-1.,-1.04324363334554));
#25972=CARTESIAN_POINT('Ctrl Pts',(-1.70391338707982,1.,-1.04324363334554));
#25973=CARTESIAN_POINT('Ctrl Pts',(-1.70010052930962,-1.,-1.03852922490789));
#25974=CARTESIAN_POINT('Ctrl Pts',(-1.70010052930962,1.,-1.03852922490789));
#25975=CARTESIAN_POINT('Ctrl Pts',(-1.69623414782771,-1.,-1.03384646003588));
#25976=CARTESIAN_POINT('Ctrl Pts',(-1.69623414782771,1.,-1.03384646003588));
#25977=CARTESIAN_POINT('Ctrl Pts',(-1.69231840863458,-1.,-1.02919977579147));
#25978=CARTESIAN_POINT('Ctrl Pts',(-1.69231840863458,1.,-1.02919977579147));
#25979=CARTESIAN_POINT('Ctrl Pts',(-1.68836910178447,-1.,-1.02460180535255));
#25980=CARTESIAN_POINT('Ctrl Pts',(-1.68836910178447,1.,-1.02460180535255));
#25981=CARTESIAN_POINT('Ctrl Pts',(-1.68440578021706,-1.,-1.02006795074201));
#25982=CARTESIAN_POINT('Ctrl Pts',(-1.68440578021706,1.,-1.02006795074201));
#25983=CARTESIAN_POINT('Ctrl Pts',(-1.68044289894798,-1.,-1.01561026162773));
#25984=CARTESIAN_POINT('Ctrl Pts',(-1.68044289894798,1.,-1.01561026162773));
#25985=CARTESIAN_POINT('Ctrl Pts',(-1.67648246776464,-1.,-1.01123236493511));
#25986=CARTESIAN_POINT('Ctrl Pts',(-1.67648246776464,1.,-1.01123236493511));
#25987=CARTESIAN_POINT('Ctrl Pts',(-1.67250335383293,-1.,-1.00692206696414));
#25988=CARTESIAN_POINT('Ctrl Pts',(-1.67250335383293,1.,-1.00692206696414));
#25989=CARTESIAN_POINT('Ctrl Pts',(-1.66846059277303,-1.,-1.00265091003727));
#25990=CARTESIAN_POINT('Ctrl Pts',(-1.66846059277303,1.,-1.00265091003727));
#25991=CARTESIAN_POINT('Ctrl Pts',(-1.66430758030376,-1.,-0.998389654952758));
#25992=CARTESIAN_POINT('Ctrl Pts',(-1.66430758030376,1.,-0.998389654952758));
#25993=CARTESIAN_POINT('Ctrl Pts',(-1.66001553809947,-1.,-0.994121836661306));
#25994=CARTESIAN_POINT('Ctrl Pts',(-1.66001553809947,1.,-0.994121836661306));
#25995=CARTESIAN_POINT('Ctrl Pts',(-1.65559044289699,-1.,-0.989855627854165));
#25996=CARTESIAN_POINT('Ctrl Pts',(-1.65559044289699,1.,-0.989855627854165));
#25997=CARTESIAN_POINT('Ctrl Pts',(-1.65110016612638,-1.,-0.985642622920821));
#25998=CARTESIAN_POINT('Ctrl Pts',(-1.65110016612638,1.,-0.985642622920821));
#25999=CARTESIAN_POINT('Ctrl Pts',(-1.64665139190656,-1.,-0.981562530939489));
#26000=CARTESIAN_POINT('Ctrl Pts',(-1.64665139190656,1.,-0.981562530939489));
#26001=CARTESIAN_POINT('Ctrl Pts',(-1.64233990826687,-1.,-0.977689794119416));
#26002=CARTESIAN_POINT('Ctrl Pts',(-1.64233990826687,1.,-0.977689794119416));
#26003=CARTESIAN_POINT('Ctrl Pts',(-1.63820952658144,-1.,-0.974066058287418));
#26004=CARTESIAN_POINT('Ctrl Pts',(-1.63820952658144,1.,-0.974066058287418));
#26005=CARTESIAN_POINT('Ctrl Pts',(-1.63420665729798,-1.,-0.970669715997509));
#26006=CARTESIAN_POINT('Ctrl Pts',(-1.63420665729798,1.,-0.970669715997509));
#26007=CARTESIAN_POINT('Ctrl Pts',(-1.63013849959461,-1.,-0.967387853230345));
#26008=CARTESIAN_POINT('Ctrl Pts',(-1.63013849959461,1.,-0.967387853230345));
#26009=CARTESIAN_POINT('Ctrl Pts',(-1.62571930670187,-1.,-0.964046107040536));
#26010=CARTESIAN_POINT('Ctrl Pts',(-1.62571930670187,1.,-0.964046107040536));
#26011=CARTESIAN_POINT('Ctrl Pts',(-1.62061638140221,-1.,-0.960438326101729));
#26012=CARTESIAN_POINT('Ctrl Pts',(-1.62061638140221,1.,-0.960438326101729));
#26013=CARTESIAN_POINT('Ctrl Pts',(-1.61449324337085,-1.,-0.956354422920671));
#26014=CARTESIAN_POINT('Ctrl Pts',(-1.61449324337085,1.,-0.956354422920671));
#26015=CARTESIAN_POINT('Ctrl Pts',(-1.60706069896936,-1.,-0.951613284356035));
#26016=CARTESIAN_POINT('Ctrl Pts',(-1.60706069896936,1.,-0.951613284356035));
#26017=CARTESIAN_POINT('Ctrl Pts',(-1.59810042043673,-1.,-0.946078063315257));
#26018=CARTESIAN_POINT('Ctrl Pts',(-1.59810042043673,1.,-0.946078063315257));
#26019=CARTESIAN_POINT('Ctrl Pts',(-1.58744937487176,-1.,-0.939646377893399));
#26020=CARTESIAN_POINT('Ctrl Pts',(-1.58744937487176,1.,-0.939646377893399));
#26021=CARTESIAN_POINT('Ctrl Pts',(-1.57499388382243,-1.,-0.932246680108685));
#26022=CARTESIAN_POINT('Ctrl Pts',(-1.57499388382243,1.,-0.932246680108685));
#26023=CARTESIAN_POINT('Ctrl Pts',(-1.56065988578893,-1.,-0.923832188944341));
#26024=CARTESIAN_POINT('Ctrl Pts',(-1.56065988578893,1.,-0.923832188944341));
#26025=CARTESIAN_POINT('Ctrl Pts',(-1.54440491149498,-1.,-0.914375919026456));
#26026=CARTESIAN_POINT('Ctrl Pts',(-1.54440491149498,1.,-0.914375919026456));
#26027=CARTESIAN_POINT('Ctrl Pts',(-1.52984849887993,-1.,-0.905967409625651));
#26028=CARTESIAN_POINT('Ctrl Pts',(-1.52984849887993,1.,-0.905967409625651));
#26029=CARTESIAN_POINT('Ctrl Pts',(-1.51805569590094,-1.,-0.899185047483511));
#26030=CARTESIAN_POINT('Ctrl Pts',(-1.51805569590094,1.,-0.899185047483511));
#26031=CARTESIAN_POINT('Ctrl Pts',(-1.50980486806688,-1.,-0.894452006964543));
#26032=CARTESIAN_POINT('Ctrl Pts',(-1.50980486806688,1.,-0.894452006964543));
#26033=CARTESIAN_POINT('Ctrl Pts',(-1.5055822144029,-1.,-0.892032620296855));
#26034=CARTESIAN_POINT('Ctrl Pts',(-1.5055822144029,1.,-0.892032620296855));
#26035=CARTESIAN_POINT('',(-1.81978687191668,1.,-1.23627494547115));
#26036=CARTESIAN_POINT('Ctrl Pts',(-1.81978687191668,1.,-1.23627494547115));
#26037=CARTESIAN_POINT('Ctrl Pts',(-1.81925017193666,1.,-1.23509651170476));
#26038=CARTESIAN_POINT('Ctrl Pts',(-1.81817389921279,1.,-1.2327422452705));
#26039=CARTESIAN_POINT('Ctrl Pts',(-1.8165508718364,1.,-1.2292186489137));
#26040=CARTESIAN_POINT('Ctrl Pts',(-1.81436959210434,1.,-1.2245361330495));
#26041=CARTESIAN_POINT('Ctrl Pts',(-1.81161420806656,1.,-1.21870906103557));
#26042=CARTESIAN_POINT('Ctrl Pts',(-1.80882996917129,1.,-1.21290815708314));
#26043=CARTESIAN_POINT('Ctrl Pts',(-1.80601678480707,1.,-1.20713356605475));
#26044=CARTESIAN_POINT('Ctrl Pts',(-1.80317454838603,1.,-1.20138548938974));
#26045=CARTESIAN_POINT('Ctrl Pts',(-1.80030314369879,1.,-1.19566418930242));
#26046=CARTESIAN_POINT('Ctrl Pts',(-1.79740245923478,1.,-1.18996997934445));
#26047=CARTESIAN_POINT('Ctrl Pts',(-1.79447240321515,1.,-1.18430321697432));
#26048=CARTESIAN_POINT('Ctrl Pts',(-1.79151291552689,1.,-1.17866429440809));
#26049=CARTESIAN_POINT('Ctrl Pts',(-1.78852398877616,1.,-1.17305363177328));
#26050=CARTESIAN_POINT('Ctrl Pts',(-1.78550566040443,1.,-1.16747166312303));
#26051=CARTESIAN_POINT('Ctrl Pts',(-1.78245795881009,1.,-1.16191881298499));
#26052=CARTESIAN_POINT('Ctrl Pts',(-1.77938085564275,1.,-1.15639547194698));
#26053=CARTESIAN_POINT('Ctrl Pts',(-1.7762742255701,1.,-1.15090197841515));
#26054=CARTESIAN_POINT('Ctrl Pts',(-1.77313777896194,1.,-1.1454385822692));
#26055=CARTESIAN_POINT('Ctrl Pts',(-1.76997111386769,1.,-1.14000548336975));
#26056=CARTESIAN_POINT('Ctrl Pts',(-1.76677384551862,1.,-1.1346029180462));
#26057=CARTESIAN_POINT('Ctrl Pts',(-1.7635457196617,1.,-1.12923123555075));
#26058=CARTESIAN_POINT('Ctrl Pts',(-1.76028671825096,1.,-1.12389096855086));
#26059=CARTESIAN_POINT('Ctrl Pts',(-1.75699720772105,1.,-1.11858293216763));
#26060=CARTESIAN_POINT('Ctrl Pts',(-1.7536777209463,1.,-1.11330807582551));
#26061=CARTESIAN_POINT('Ctrl Pts',(-1.7503286607592,1.,-1.10806728183007));
#26062=CARTESIAN_POINT('Ctrl Pts',(-1.74695004214923,1.,-1.10286118991143));
#26063=CARTESIAN_POINT('Ctrl Pts',(-1.74354119236208,1.,-1.09768999241225));
#26064=CARTESIAN_POINT('Ctrl Pts',(-1.74010053962247,1.,-1.09255329056493));
#26065=CARTESIAN_POINT('Ctrl Pts',(-1.73662628326091,1.,-1.08745056285427));
#26066=CARTESIAN_POINT('Ctrl Pts',(-1.73311705663407,1.,-1.08238162784749));
#26067=CARTESIAN_POINT('Ctrl Pts',(-1.72957248977424,1.,-1.0773470373727));
#26068=CARTESIAN_POINT('Ctrl Pts',(-1.72599406198488,1.,-1.07234866990252));
#26069=CARTESIAN_POINT('Ctrl Pts',(-1.72238500928453,1.,-1.06738966975462));
#26070=CARTESIAN_POINT('Ctrl Pts',(-1.71874858456904,1.,-1.06247324680647));
#26071=CARTESIAN_POINT('Ctrl Pts',(-1.7150865442702,1.,-1.05760163192479));
#26072=CARTESIAN_POINT('Ctrl Pts',(-1.71139783543989,1.,-1.05277517202855));
#26073=CARTESIAN_POINT('Ctrl Pts',(-1.70767646263649,1.,-1.04799085404995));
#26074=CARTESIAN_POINT('Ctrl Pts',(-1.70391338707982,1.,-1.04324363334554));
#26075=CARTESIAN_POINT('Ctrl Pts',(-1.70010052930962,1.,-1.03852922490789));
#26076=CARTESIAN_POINT('Ctrl Pts',(-1.69623414782771,1.,-1.03384646003588));
#26077=CARTESIAN_POINT('Ctrl Pts',(-1.69231840863458,1.,-1.02919977579147));
#26078=CARTESIAN_POINT('Ctrl Pts',(-1.68836910178447,1.,-1.02460180535255));
#26079=CARTESIAN_POINT('Ctrl Pts',(-1.68440578021706,1.,-1.02006795074201));
#26080=CARTESIAN_POINT('Ctrl Pts',(-1.68044289894798,1.,-1.01561026162773));
#26081=CARTESIAN_POINT('Ctrl Pts',(-1.67648246776464,1.,-1.01123236493511));
#26082=CARTESIAN_POINT('Ctrl Pts',(-1.67250335383293,1.,-1.00692206696414));
#26083=CARTESIAN_POINT('Ctrl Pts',(-1.66846059277303,1.,-1.00265091003727));
#26084=CARTESIAN_POINT('Ctrl Pts',(-1.66430758030376,1.,-0.998389654952758));
#26085=CARTESIAN_POINT('Ctrl Pts',(-1.66001553809947,1.,-0.994121836661306));
#26086=CARTESIAN_POINT('Ctrl Pts',(-1.65559044289699,1.,-0.989855627854165));
#26087=CARTESIAN_POINT('Ctrl Pts',(-1.65110016612638,1.,-0.985642622920821));
#26088=CARTESIAN_POINT('Ctrl Pts',(-1.64665139190656,1.,-0.981562530939489));
#26089=CARTESIAN_POINT('Ctrl Pts',(-1.64233990826687,1.,-0.977689794119416));
#26090=CARTESIAN_POINT('Ctrl Pts',(-1.63820952658144,1.,-0.974066058287418));
#26091=CARTESIAN_POINT('Ctrl Pts',(-1.63420665729798,1.,-0.970669715997509));
#26092=CARTESIAN_POINT('Ctrl Pts',(-1.63013849959461,1.,-0.967387853230345));
#26093=CARTESIAN_POINT('Ctrl Pts',(-1.62571930670187,1.,-0.964046107040536));
#26094=CARTESIAN_POINT('Ctrl Pts',(-1.62061638140221,1.,-0.960438326101729));
#26095=CARTESIAN_POINT('Ctrl Pts',(-1.61449324337085,1.,-0.956354422920671));
#26096=CARTESIAN_POINT('Ctrl Pts',(-1.60706069896936,1.,-0.951613284356035));
#26097=CARTESIAN_POINT('Ctrl Pts',(-1.59810042043673,1.,-0.946078063315257));
#26098=CARTESIAN_POINT('Ctrl Pts',(-1.58744937487176,1.,-0.939646377893399));
#26099=CARTESIAN_POINT('Ctrl Pts',(-1.57499388382243,1.,-0.932246680108685));
#26100=CARTESIAN_POINT('Ctrl Pts',(-1.56065988578893,1.,-0.923832188944341));
#26101=CARTESIAN_POINT('Ctrl Pts',(-1.54440491149498,1.,-0.914375919026456));
#26102=CARTESIAN_POINT('Ctrl Pts',(-1.52984849887993,1.,-0.905967409625651));
#26103=CARTESIAN_POINT('Ctrl Pts',(-1.51805569590094,1.,-0.899185047483511));
#26104=CARTESIAN_POINT('Ctrl Pts',(-1.50980486806688,1.,-0.894452006964543));
#26105=CARTESIAN_POINT('Ctrl Pts',(-1.5055822144029,1.,-0.892032620296855));
#26106=CARTESIAN_POINT('',(-1.81978687191668,0.,-1.23627494547115));
#26107=CARTESIAN_POINT('Origin',(-1.73811241238545,0.,-1.34869019493419));
#26108=CARTESIAN_POINT('',(-1.73811241238545,1.,-1.34869019493419));
#26109=CARTESIAN_POINT('',(-1.81978687191668,1.,-1.23627494547115));
#26110=CARTESIAN_POINT('',(-1.73811241238545,0.,-1.34869019493419));
#26111=CARTESIAN_POINT('Ctrl Pts',(-1.31362392696032,-1.,-1.15624053661742));
#26112=CARTESIAN_POINT('Ctrl Pts',(-1.31362392696032,1.,-1.15624053661742));
#26113=CARTESIAN_POINT('Ctrl Pts',(-1.31722977216397,-1.,-1.15950888730809));
#26114=CARTESIAN_POINT('Ctrl Pts',(-1.31722977216397,1.,-1.15950888730809));
#26115=CARTESIAN_POINT('Ctrl Pts',(-1.32428080721772,-1.,-1.16589330093588));
#26116=CARTESIAN_POINT('Ctrl Pts',(-1.32428080721772,1.,-1.16589330093588));
#26117=CARTESIAN_POINT('Ctrl Pts',(-1.33437539347008,-1.,-1.17501305789857));
#26118=CARTESIAN_POINT('Ctrl Pts',(-1.33437539347008,1.,-1.17501305789857));
#26119=CARTESIAN_POINT('Ctrl Pts',(-1.34687054001093,-1.,-1.18625865667441));
#26120=CARTESIAN_POINT('Ctrl Pts',(-1.34687054001093,1.,-1.18625865667441));
#26121=CARTESIAN_POINT('Ctrl Pts',(-1.36088705043885,-1.,-1.1987959077932));
#26122=CARTESIAN_POINT('Ctrl Pts',(-1.36088705043885,1.,-1.1987959077932));
#26123=CARTESIAN_POINT('Ctrl Pts',(-1.37331915607905,-1.,-1.20982812925645));
#26124=CARTESIAN_POINT('Ctrl Pts',(-1.37331915607905,1.,-1.20982812925645));
#26125=CARTESIAN_POINT('Ctrl Pts',(-1.38420564527715,-1.,-1.21938737280852));
#26126=CARTESIAN_POINT('Ctrl Pts',(-1.38420564527715,1.,-1.21938737280852));
#26127=CARTESIAN_POINT('Ctrl Pts',(-1.39361389568796,-1.,-1.22752961899387));
#26128=CARTESIAN_POINT('Ctrl Pts',(-1.39361389568796,1.,-1.22752961899387));
#26129=CARTESIAN_POINT('Ctrl Pts',(-1.40164708206106,-1.,-1.23434087290423));
#26130=CARTESIAN_POINT('Ctrl Pts',(-1.40164708206106,1.,-1.23434087290423));
#26131=CARTESIAN_POINT('Ctrl Pts',(-1.40845295531283,-1.,-1.23994455029534));
#26132=CARTESIAN_POINT('Ctrl Pts',(-1.40845295531283,1.,-1.23994455029534));
#26133=CARTESIAN_POINT('Ctrl Pts',(-1.41422913175179,-1.,-1.24450600513056));
#26134=CARTESIAN_POINT('Ctrl Pts',(-1.41422913175179,1.,-1.24450600513056));
#26135=CARTESIAN_POINT('Ctrl Pts',(-1.41923722596025,-1.,-1.24824430986571));
#26136=CARTESIAN_POINT('Ctrl Pts',(-1.41923722596025,1.,-1.24824430986571));
#26137=CARTESIAN_POINT('Ctrl Pts',(-1.42378102115575,-1.,-1.2514145557001));
#26138=CARTESIAN_POINT('Ctrl Pts',(-1.42378102115575,1.,-1.2514145557001));
#26139=CARTESIAN_POINT('Ctrl Pts',(-1.42815938799387,-1.,-1.25426945222639));
#26140=CARTESIAN_POINT('Ctrl Pts',(-1.42815938799387,1.,-1.25426945222639));
#26141=CARTESIAN_POINT('Ctrl Pts',(-1.43262645609691,-1.,-1.25702687965755));
#26142=CARTESIAN_POINT('Ctrl Pts',(-1.43262645609691,1.,-1.25702687965755));
#26143=CARTESIAN_POINT('Ctrl Pts',(-1.43734919180848,-1.,-1.25983531012005));
#26144=CARTESIAN_POINT('Ctrl Pts',(-1.43734919180848,1.,-1.25983531012005));
#26145=CARTESIAN_POINT('Ctrl Pts',(-1.44236470511303,-1.,-1.26273903323859));
#26146=CARTESIAN_POINT('Ctrl Pts',(-1.44236470511303,1.,-1.26273903323859));
#26147=CARTESIAN_POINT('Ctrl Pts',(-1.44761985001662,-1.,-1.26570925118868));
#26148=CARTESIAN_POINT('Ctrl Pts',(-1.44761985001662,1.,-1.26570925118868));
#26149=CARTESIAN_POINT('Ctrl Pts',(-1.45301422764247,-1.,-1.2686778680489));
#26150=CARTESIAN_POINT('Ctrl Pts',(-1.45301422764247,1.,-1.2686778680489));
#26151=CARTESIAN_POINT('Ctrl Pts',(-1.45843906294697,-1.,-1.27156805265289));
#26152=CARTESIAN_POINT('Ctrl Pts',(-1.45843906294697,1.,-1.27156805265289));
#26153=CARTESIAN_POINT('Ctrl Pts',(-1.46382431332476,-1.,-1.27433119897822));
#26154=CARTESIAN_POINT('Ctrl Pts',(-1.46382431332476,1.,-1.27433119897822));
#26155=CARTESIAN_POINT('Ctrl Pts',(-1.46916035917133,-1.,-1.27696414831089));
#26156=CARTESIAN_POINT('Ctrl Pts',(-1.46916035917133,1.,-1.27696414831089));
#26157=CARTESIAN_POINT('Ctrl Pts',(-1.4744717526707,-1.,-1.2794891824849));
#26158=CARTESIAN_POINT('Ctrl Pts',(-1.4744717526707,1.,-1.2794891824849));
#26159=CARTESIAN_POINT('Ctrl Pts',(-1.47980070347095,-1.,-1.28194158939517));
#26160=CARTESIAN_POINT('Ctrl Pts',(-1.47980070347095,1.,-1.28194158939517));
#26161=CARTESIAN_POINT('Ctrl Pts',(-1.4851881711891,-1.,-1.28435533880201));
#26162=CARTESIAN_POINT('Ctrl Pts',(-1.4851881711891,1.,-1.28435533880201));
#26163=CARTESIAN_POINT('Ctrl Pts',(-1.4906522831278,-1.,-1.2867467611644));
#26164=CARTESIAN_POINT('Ctrl Pts',(-1.4906522831278,1.,-1.2867467611644));
#26165=CARTESIAN_POINT('Ctrl Pts',(-1.49618896881754,-1.,-1.28911506584254));
#26166=CARTESIAN_POINT('Ctrl Pts',(-1.49618896881754,1.,-1.28911506584254));
#26167=CARTESIAN_POINT('Ctrl Pts',(-1.50178230149776,-1.,-1.29145022885181));
#26168=CARTESIAN_POINT('Ctrl Pts',(-1.50178230149776,1.,-1.29145022885181));
#26169=CARTESIAN_POINT('Ctrl Pts',(-1.50741159078365,-1.,-1.29373841372842));
#26170=CARTESIAN_POINT('Ctrl Pts',(-1.50741159078365,1.,-1.29373841372842));
#26171=CARTESIAN_POINT('Ctrl Pts',(-1.51305994241402,-1.,-1.29596850710509));
#26172=CARTESIAN_POINT('Ctrl Pts',(-1.51305994241402,1.,-1.29596850710509));
#26173=CARTESIAN_POINT('Ctrl Pts',(-1.51872184912724,-1.,-1.29813791800747));
#26174=CARTESIAN_POINT('Ctrl Pts',(-1.51872184912724,1.,-1.29813791800747));
#26175=CARTESIAN_POINT('Ctrl Pts',(-1.52439957861062,-1.,-1.30024984366328));
#26176=CARTESIAN_POINT('Ctrl Pts',(-1.52439957861062,1.,-1.30024984366328));
#26177=CARTESIAN_POINT('Ctrl Pts',(-1.53009970283891,-1.,-1.30231064395568));
#26178=CARTESIAN_POINT('Ctrl Pts',(-1.53009970283891,1.,-1.30231064395568));
#26179=CARTESIAN_POINT('Ctrl Pts',(-1.53582981268977,-1.,-1.30432735639489));
#26180=CARTESIAN_POINT('Ctrl Pts',(-1.53582981268977,1.,-1.30432735639489));
#26181=CARTESIAN_POINT('Ctrl Pts',(-1.54159462645432,-1.,-1.30630475189556));
#26182=CARTESIAN_POINT('Ctrl Pts',(-1.54159462645432,1.,-1.30630475189556));
#26183=CARTESIAN_POINT('Ctrl Pts',(-1.54739413957185,-1.,-1.30824393907473));
#26184=CARTESIAN_POINT('Ctrl Pts',(-1.54739413957185,1.,-1.30824393907473));
#26185=CARTESIAN_POINT('Ctrl Pts',(-1.55322568759481,-1.,-1.31014393684222));
#26186=CARTESIAN_POINT('Ctrl Pts',(-1.55322568759481,1.,-1.31014393684222));
#26187=CARTESIAN_POINT('Ctrl Pts',(-1.55908521254821,-1.,-1.31200264341696));
#26188=CARTESIAN_POINT('Ctrl Pts',(-1.55908521254821,1.,-1.31200264341696));
#26189=CARTESIAN_POINT('Ctrl Pts',(-1.56496872402353,-1.,-1.31381795281002));
#26190=CARTESIAN_POINT('Ctrl Pts',(-1.56496872402353,1.,-1.31381795281002));
#26191=CARTESIAN_POINT('Ctrl Pts',(-1.57087397835723,-1.,-1.31558903860016));
#26192=CARTESIAN_POINT('Ctrl Pts',(-1.57087397835723,1.,-1.31558903860016));
#26193=CARTESIAN_POINT('Ctrl Pts',(-1.5768005650559,-1.,-1.31731642317187));
#26194=CARTESIAN_POINT('Ctrl Pts',(-1.5768005650559,1.,-1.31731642317187));
#26195=CARTESIAN_POINT('Ctrl Pts',(-1.58274907898834,-1.,-1.31900135021432));
#26196=CARTESIAN_POINT('Ctrl Pts',(-1.58274907898834,1.,-1.31900135021432));
#26197=CARTESIAN_POINT('Ctrl Pts',(-1.58872057258245,-1.,-1.32064537110892));
#26198=CARTESIAN_POINT('Ctrl Pts',(-1.58872057258245,1.,-1.32064537110892));
#26199=CARTESIAN_POINT('Ctrl Pts',(-1.59471591079403,-1.,-1.32224985747682));
#26200=CARTESIAN_POINT('Ctrl Pts',(-1.59471591079403,1.,-1.32224985747682));
#26201=CARTESIAN_POINT('Ctrl Pts',(-1.60073511858687,-1.,-1.32381550858256));
#26202=CARTESIAN_POINT('Ctrl Pts',(-1.60073511858687,1.,-1.32381550858256));
#26203=CARTESIAN_POINT('Ctrl Pts',(-1.60677758290954,-1.,-1.32534250785782));
#26204=CARTESIAN_POINT('Ctrl Pts',(-1.60677758290954,1.,-1.32534250785782));
#26205=CARTESIAN_POINT('Ctrl Pts',(-1.6128423401575,-1.,-1.32683074483356));
#26206=CARTESIAN_POINT('Ctrl Pts',(-1.6128423401575,1.,-1.32683074483356));
#26207=CARTESIAN_POINT('Ctrl Pts',(-1.61892832270724,-1.,-1.32828000610449));
#26208=CARTESIAN_POINT('Ctrl Pts',(-1.61892832270724,1.,-1.32828000610449));
#26209=CARTESIAN_POINT('Ctrl Pts',(-1.62503464209797,-1.,-1.3296901950568));
#26210=CARTESIAN_POINT('Ctrl Pts',(-1.62503464209797,1.,-1.3296901950568));
#26211=CARTESIAN_POINT('Ctrl Pts',(-1.63116079730923,-1.,-1.33106149345645));
#26212=CARTESIAN_POINT('Ctrl Pts',(-1.63116079730923,1.,-1.33106149345645));
#26213=CARTESIAN_POINT('Ctrl Pts',(-1.63730653475089,-1.,-1.33239425103724));
#26214=CARTESIAN_POINT('Ctrl Pts',(-1.63730653475089,1.,-1.33239425103724));
#26215=CARTESIAN_POINT('Ctrl Pts',(-1.6434717485603,-1.,-1.33368890676572));
#26216=CARTESIAN_POINT('Ctrl Pts',(-1.6434717485603,1.,-1.33368890676572));
#26217=CARTESIAN_POINT('Ctrl Pts',(-1.6496563728683,-1.,-1.33494590467993));
#26218=CARTESIAN_POINT('Ctrl Pts',(-1.6496563728683,1.,-1.33494590467993));
#26219=CARTESIAN_POINT('Ctrl Pts',(-1.65586025952593,-1.,-1.33616559745172));
#26220=CARTESIAN_POINT('Ctrl Pts',(-1.65586025952593,1.,-1.33616559745172));
#26221=CARTESIAN_POINT('Ctrl Pts',(-1.66208312541983,-1.,-1.33734820885262));
#26222=CARTESIAN_POINT('Ctrl Pts',(-1.66208312541983,1.,-1.33734820885262));
#26223=CARTESIAN_POINT('Ctrl Pts',(-1.66832460783989,-1.,-1.33849388654388));
#26224=CARTESIAN_POINT('Ctrl Pts',(-1.66832460783989,1.,-1.33849388654388));
#26225=CARTESIAN_POINT('Ctrl Pts',(-1.67458429426086,-1.,-1.3396027347034));
#26226=CARTESIAN_POINT('Ctrl Pts',(-1.67458429426086,1.,-1.3396027347034));
#26227=CARTESIAN_POINT('Ctrl Pts',(-1.68086176030362,-1.,-1.34067485185203));
#26228=CARTESIAN_POINT('Ctrl Pts',(-1.68086176030362,1.,-1.34067485185203));
#26229=CARTESIAN_POINT('Ctrl Pts',(-1.68715660868764,-1.,-1.341710374848));
#26230=CARTESIAN_POINT('Ctrl Pts',(-1.68715660868764,1.,-1.341710374848));
#26231=CARTESIAN_POINT('Ctrl Pts',(-1.6934684849687,-1.,-1.34270948206319));
#26232=CARTESIAN_POINT('Ctrl Pts',(-1.6934684849687,1.,-1.34270948206319));
#26233=CARTESIAN_POINT('Ctrl Pts',(-1.69979707754427,-1.,-1.34367237124483));
#26234=CARTESIAN_POINT('Ctrl Pts',(-1.69979707754427,1.,-1.34367237124483));
#26235=CARTESIAN_POINT('Ctrl Pts',(-1.70614212266738,-1.,-1.34459924533831));
#26236=CARTESIAN_POINT('Ctrl Pts',(-1.70614212266738,1.,-1.34459924533831));
#26237=CARTESIAN_POINT('Ctrl Pts',(-1.71250340686822,-1.,-1.34549029589416));
#26238=CARTESIAN_POINT('Ctrl Pts',(-1.71250340686822,1.,-1.34549029589416));
#26239=CARTESIAN_POINT('Ctrl Pts',(-1.7188807715049,-1.,-1.34634568653227));
#26240=CARTESIAN_POINT('Ctrl Pts',(-1.7188807715049,1.,-1.34634568653227));
#26241=CARTESIAN_POINT('Ctrl Pts',(-1.72527410680674,-1.,-1.34716554819527));
#26242=CARTESIAN_POINT('Ctrl Pts',(-1.72527410680674,1.,-1.34716554819527));
#26243=CARTESIAN_POINT('Ctrl Pts',(-1.7304014965394,-1.,-1.34779309152035));
#26244=CARTESIAN_POINT('Ctrl Pts',(-1.7304014965394,1.,-1.34779309152035));
#26245=CARTESIAN_POINT('Ctrl Pts',(-1.73425417885907,-1.,-1.34824783112887));
#26246=CARTESIAN_POINT('Ctrl Pts',(-1.73425417885907,1.,-1.34824783112887));
#26247=CARTESIAN_POINT('Ctrl Pts',(-1.73682580585691,-1.,-1.34854391898045));
#26248=CARTESIAN_POINT('Ctrl Pts',(-1.73682580585691,1.,-1.34854391898045));
#26249=CARTESIAN_POINT('Ctrl Pts',(-1.73811241238545,-1.,-1.34869019493419));
#26250=CARTESIAN_POINT('Ctrl Pts',(-1.73811241238545,1.,-1.34869019493419));
#26251=CARTESIAN_POINT('',(-1.31362392696032,1.,-1.15624053661742));
#26252=CARTESIAN_POINT('Ctrl Pts',(-1.31362392696032,1.,-1.15624053661742));
#26253=CARTESIAN_POINT('Ctrl Pts',(-1.31722977216397,1.,-1.15950888730809));
#26254=CARTESIAN_POINT('Ctrl Pts',(-1.32428080721772,1.,-1.16589330093588));
#26255=CARTESIAN_POINT('Ctrl Pts',(-1.33437539347008,1.,-1.17501305789857));
#26256=CARTESIAN_POINT('Ctrl Pts',(-1.34687054001093,1.,-1.18625865667441));
#26257=CARTESIAN_POINT('Ctrl Pts',(-1.36088705043885,1.,-1.1987959077932));
#26258=CARTESIAN_POINT('Ctrl Pts',(-1.37331915607905,1.,-1.20982812925645));
#26259=CARTESIAN_POINT('Ctrl Pts',(-1.38420564527715,1.,-1.21938737280852));
#26260=CARTESIAN_POINT('Ctrl Pts',(-1.39361389568796,1.,-1.22752961899387));
#26261=CARTESIAN_POINT('Ctrl Pts',(-1.40164708206106,1.,-1.23434087290423));
#26262=CARTESIAN_POINT('Ctrl Pts',(-1.40845295531283,1.,-1.23994455029534));
#26263=CARTESIAN_POINT('Ctrl Pts',(-1.41422913175179,1.,-1.24450600513056));
#26264=CARTESIAN_POINT('Ctrl Pts',(-1.41923722596025,1.,-1.24824430986571));
#26265=CARTESIAN_POINT('Ctrl Pts',(-1.42378102115575,1.,-1.2514145557001));
#26266=CARTESIAN_POINT('Ctrl Pts',(-1.42815938799387,1.,-1.25426945222639));
#26267=CARTESIAN_POINT('Ctrl Pts',(-1.43262645609691,1.,-1.25702687965755));
#26268=CARTESIAN_POINT('Ctrl Pts',(-1.43734919180848,1.,-1.25983531012005));
#26269=CARTESIAN_POINT('Ctrl Pts',(-1.44236470511303,1.,-1.26273903323859));
#26270=CARTESIAN_POINT('Ctrl Pts',(-1.44761985001662,1.,-1.26570925118868));
#26271=CARTESIAN_POINT('Ctrl Pts',(-1.45301422764247,1.,-1.2686778680489));
#26272=CARTESIAN_POINT('Ctrl Pts',(-1.45843906294697,1.,-1.27156805265289));
#26273=CARTESIAN_POINT('Ctrl Pts',(-1.46382431332476,1.,-1.27433119897822));
#26274=CARTESIAN_POINT('Ctrl Pts',(-1.46916035917133,1.,-1.27696414831089));
#26275=CARTESIAN_POINT('Ctrl Pts',(-1.4744717526707,1.,-1.2794891824849));
#26276=CARTESIAN_POINT('Ctrl Pts',(-1.47980070347095,1.,-1.28194158939517));
#26277=CARTESIAN_POINT('Ctrl Pts',(-1.4851881711891,1.,-1.28435533880201));
#26278=CARTESIAN_POINT('Ctrl Pts',(-1.4906522831278,1.,-1.2867467611644));
#26279=CARTESIAN_POINT('Ctrl Pts',(-1.49618896881754,1.,-1.28911506584254));
#26280=CARTESIAN_POINT('Ctrl Pts',(-1.50178230149776,1.,-1.29145022885181));
#26281=CARTESIAN_POINT('Ctrl Pts',(-1.50741159078365,1.,-1.29373841372842));
#26282=CARTESIAN_POINT('Ctrl Pts',(-1.51305994241402,1.,-1.29596850710509));
#26283=CARTESIAN_POINT('Ctrl Pts',(-1.51872184912724,1.,-1.29813791800747));
#26284=CARTESIAN_POINT('Ctrl Pts',(-1.52439957861062,1.,-1.30024984366328));
#26285=CARTESIAN_POINT('Ctrl Pts',(-1.53009970283891,1.,-1.30231064395568));
#26286=CARTESIAN_POINT('Ctrl Pts',(-1.53582981268977,1.,-1.30432735639489));
#26287=CARTESIAN_POINT('Ctrl Pts',(-1.54159462645432,1.,-1.30630475189556));
#26288=CARTESIAN_POINT('Ctrl Pts',(-1.54739413957185,1.,-1.30824393907473));
#26289=CARTESIAN_POINT('Ctrl Pts',(-1.55322568759481,1.,-1.31014393684222));
#26290=CARTESIAN_POINT('Ctrl Pts',(-1.55908521254821,1.,-1.31200264341696));
#26291=CARTESIAN_POINT('Ctrl Pts',(-1.56496872402353,1.,-1.31381795281002));
#26292=CARTESIAN_POINT('Ctrl Pts',(-1.57087397835723,1.,-1.31558903860016));
#26293=CARTESIAN_POINT('Ctrl Pts',(-1.5768005650559,1.,-1.31731642317187));
#26294=CARTESIAN_POINT('Ctrl Pts',(-1.58274907898834,1.,-1.31900135021432));
#26295=CARTESIAN_POINT('Ctrl Pts',(-1.58872057258245,1.,-1.32064537110892));
#26296=CARTESIAN_POINT('Ctrl Pts',(-1.59471591079403,1.,-1.32224985747682));
#26297=CARTESIAN_POINT('Ctrl Pts',(-1.60073511858687,1.,-1.32381550858256));
#26298=CARTESIAN_POINT('Ctrl Pts',(-1.60677758290954,1.,-1.32534250785782));
#26299=CARTESIAN_POINT('Ctrl Pts',(-1.6128423401575,1.,-1.32683074483356));
#26300=CARTESIAN_POINT('Ctrl Pts',(-1.61892832270724,1.,-1.32828000610449));
#26301=CARTESIAN_POINT('Ctrl Pts',(-1.62503464209797,1.,-1.3296901950568));
#26302=CARTESIAN_POINT('Ctrl Pts',(-1.63116079730923,1.,-1.33106149345645));
#26303=CARTESIAN_POINT('Ctrl Pts',(-1.63730653475089,1.,-1.33239425103724));
#26304=CARTESIAN_POINT('Ctrl Pts',(-1.6434717485603,1.,-1.33368890676572));
#26305=CARTESIAN_POINT('Ctrl Pts',(-1.6496563728683,1.,-1.33494590467993));
#26306=CARTESIAN_POINT('Ctrl Pts',(-1.65586025952593,1.,-1.33616559745172));
#26307=CARTESIAN_POINT('Ctrl Pts',(-1.66208312541983,1.,-1.33734820885262));
#26308=CARTESIAN_POINT('Ctrl Pts',(-1.66832460783989,1.,-1.33849388654388));
#26309=CARTESIAN_POINT('Ctrl Pts',(-1.67458429426086,1.,-1.3396027347034));
#26310=CARTESIAN_POINT('Ctrl Pts',(-1.68086176030362,1.,-1.34067485185203));
#26311=CARTESIAN_POINT('Ctrl Pts',(-1.68715660868764,1.,-1.341710374848));
#26312=CARTESIAN_POINT('Ctrl Pts',(-1.6934684849687,1.,-1.34270948206319));
#26313=CARTESIAN_POINT('Ctrl Pts',(-1.69979707754427,1.,-1.34367237124483));
#26314=CARTESIAN_POINT('Ctrl Pts',(-1.70614212266738,1.,-1.34459924533831));
#26315=CARTESIAN_POINT('Ctrl Pts',(-1.71250340686822,1.,-1.34549029589416));
#26316=CARTESIAN_POINT('Ctrl Pts',(-1.7188807715049,1.,-1.34634568653227));
#26317=CARTESIAN_POINT('Ctrl Pts',(-1.72527410680674,1.,-1.34716554819527));
#26318=CARTESIAN_POINT('Ctrl Pts',(-1.7304014965394,1.,-1.34779309152035));
#26319=CARTESIAN_POINT('Ctrl Pts',(-1.73425417885907,1.,-1.34824783112887));
#26320=CARTESIAN_POINT('Ctrl Pts',(-1.73682580585691,1.,-1.34854391898045));
#26321=CARTESIAN_POINT('Ctrl Pts',(-1.73811241238545,1.,-1.34869019493419));
#26322=CARTESIAN_POINT('',(-1.31362392696032,0.,-1.15624053661742));
#26323=CARTESIAN_POINT('Origin',(0.,0.,0.));
#26324=CARTESIAN_POINT('',(-1.15624053661742,1.,-1.31362392696033));
#26325=CARTESIAN_POINT('Origin',(0.,1.,0.));
#26326=CARTESIAN_POINT('',(-1.15624053661742,0.,-1.31362392696033));
#26327=CARTESIAN_POINT('Ctrl Pts',(-1.34869019493419,-1.,-1.73811241238545));
#26328=CARTESIAN_POINT('Ctrl Pts',(-1.34869019493419,1.,-1.73811241238545));
#26329=CARTESIAN_POINT('Ctrl Pts',(-1.34854391898145,-1.,-1.73682580585819));
#26330=CARTESIAN_POINT('Ctrl Pts',(-1.34854391898145,1.,-1.73682580585819));
#26331=CARTESIAN_POINT('Ctrl Pts',(-1.34824783113158,-1.,-1.73425417886255));
#26332=CARTESIAN_POINT('Ctrl Pts',(-1.34824783113158,1.,-1.73425417886255));
#26333=CARTESIAN_POINT('Ctrl Pts',(-1.3477930915247,-1.,-1.73040149654497));
#26334=CARTESIAN_POINT('Ctrl Pts',(-1.3477930915247,1.,-1.73040149654497));
#26335=CARTESIAN_POINT('Ctrl Pts',(-1.34716554820013,-1.,-1.72527410681298));
#26336=CARTESIAN_POINT('Ctrl Pts',(-1.34716554820013,1.,-1.72527410681298));
#26337=CARTESIAN_POINT('Ctrl Pts',(-1.34634568653586,-1.,-1.7188807715095));
#26338=CARTESIAN_POINT('Ctrl Pts',(-1.34634568653586,1.,-1.7188807715095));
#26339=CARTESIAN_POINT('Ctrl Pts',(-1.34549029589563,-1.,-1.71250340687011));
#26340=CARTESIAN_POINT('Ctrl Pts',(-1.34549029589563,1.,-1.71250340687011));
#26341=CARTESIAN_POINT('Ctrl Pts',(-1.34459924533783,-1.,-1.70614212266676));
#26342=CARTESIAN_POINT('Ctrl Pts',(-1.34459924533783,1.,-1.70614212266676));
#26343=CARTESIAN_POINT('Ctrl Pts',(-1.34367237124322,-1.,-1.69979707754221));
#26344=CARTESIAN_POINT('Ctrl Pts',(-1.34367237124322,1.,-1.69979707754221));
#26345=CARTESIAN_POINT('Ctrl Pts',(-1.34270948206139,-1.,-1.6934684849664));
#26346=CARTESIAN_POINT('Ctrl Pts',(-1.34270948206139,1.,-1.6934684849664));
#26347=CARTESIAN_POINT('Ctrl Pts',(-1.34171037484673,-1.,-1.68715660868602));
#26348=CARTESIAN_POINT('Ctrl Pts',(-1.34171037484673,1.,-1.68715660868602));
#26349=CARTESIAN_POINT('Ctrl Pts',(-1.3406748518516,-1.,-1.68086176030308));
#26350=CARTESIAN_POINT('Ctrl Pts',(-1.3406748518516,1.,-1.68086176030308));
#26351=CARTESIAN_POINT('Ctrl Pts',(-1.33960273470372,-1.,-1.67458429426126));
#26352=CARTESIAN_POINT('Ctrl Pts',(-1.33960273470372,1.,-1.67458429426126));
#26353=CARTESIAN_POINT('Ctrl Pts',(-1.33849388654458,-1.,-1.66832460784078));
#26354=CARTESIAN_POINT('Ctrl Pts',(-1.33849388654458,1.,-1.66832460784078));
#26355=CARTESIAN_POINT('Ctrl Pts',(-1.33734820885331,-1.,-1.66208312542073));
#26356=CARTESIAN_POINT('Ctrl Pts',(-1.33734820885331,1.,-1.66208312542073));
#26357=CARTESIAN_POINT('Ctrl Pts',(-1.33616559745217,-1.,-1.65586025952651));
#26358=CARTESIAN_POINT('Ctrl Pts',(-1.33616559745217,1.,-1.65586025952651));
#26359=CARTESIAN_POINT('Ctrl Pts',(-1.33494590468003,-1.,-1.64965637286843));
#26360=CARTESIAN_POINT('Ctrl Pts',(-1.33494590468003,1.,-1.64965637286843));
#26361=CARTESIAN_POINT('Ctrl Pts',(-1.33368890676554,-1.,-1.64347174856007));
#26362=CARTESIAN_POINT('Ctrl Pts',(-1.33368890676554,1.,-1.64347174856007));
#26363=CARTESIAN_POINT('Ctrl Pts',(-1.33239425103694,-1.,-1.6373065347505));
#26364=CARTESIAN_POINT('Ctrl Pts',(-1.33239425103694,1.,-1.6373065347505));
#26365=CARTESIAN_POINT('Ctrl Pts',(-1.33106149345618,-1.,-1.63116079730887));
#26366=CARTESIAN_POINT('Ctrl Pts',(-1.33106149345618,1.,-1.63116079730887));
#26367=CARTESIAN_POINT('Ctrl Pts',(-1.32969019505665,-1.,-1.62503464209777));
#26368=CARTESIAN_POINT('Ctrl Pts',(-1.32969019505665,1.,-1.62503464209777));
#26369=CARTESIAN_POINT('Ctrl Pts',(-1.32828000610448,-1.,-1.61892832270723));
#26370=CARTESIAN_POINT('Ctrl Pts',(-1.32828000610448,1.,-1.61892832270723));
#26371=CARTESIAN_POINT('Ctrl Pts',(-1.32683074483365,-1.,-1.61284234015762));
#26372=CARTESIAN_POINT('Ctrl Pts',(-1.32683074483365,1.,-1.61284234015762));
#26373=CARTESIAN_POINT('Ctrl Pts',(-1.32534250785794,-1.,-1.6067775829097));
#26374=CARTESIAN_POINT('Ctrl Pts',(-1.32534250785794,1.,-1.6067775829097));
#26375=CARTESIAN_POINT('Ctrl Pts',(-1.32381550858266,-1.,-1.600735118587));
#26376=CARTESIAN_POINT('Ctrl Pts',(-1.32381550858266,1.,-1.600735118587));
#26377=CARTESIAN_POINT('Ctrl Pts',(-1.32224985747686,-1.,-1.59471591079408));
#26378=CARTESIAN_POINT('Ctrl Pts',(-1.32224985747686,1.,-1.59471591079408));
#26379=CARTESIAN_POINT('Ctrl Pts',(-1.32064537110891,-1.,-1.58872057258244));
#26380=CARTESIAN_POINT('Ctrl Pts',(-1.32064537110891,1.,-1.58872057258244));
#26381=CARTESIAN_POINT('Ctrl Pts',(-1.31900135021428,-1.,-1.58274907898829));
#26382=CARTESIAN_POINT('Ctrl Pts',(-1.31900135021428,1.,-1.58274907898829));
#26383=CARTESIAN_POINT('Ctrl Pts',(-1.31731642317183,-1.,-1.57680056505585));
#26384=CARTESIAN_POINT('Ctrl Pts',(-1.31731642317183,1.,-1.57680056505585));
#26385=CARTESIAN_POINT('Ctrl Pts',(-1.31558903860015,-1.,-1.57087397835721));
#26386=CARTESIAN_POINT('Ctrl Pts',(-1.31558903860015,1.,-1.57087397835721));
#26387=CARTESIAN_POINT('Ctrl Pts',(-1.31381795281002,-1.,-1.56496872402352));
#26388=CARTESIAN_POINT('Ctrl Pts',(-1.31381795281002,1.,-1.56496872402352));
#26389=CARTESIAN_POINT('Ctrl Pts',(-1.31200264341696,-1.,-1.55908521254822));
#26390=CARTESIAN_POINT('Ctrl Pts',(-1.31200264341696,1.,-1.55908521254822));
#26391=CARTESIAN_POINT('Ctrl Pts',(-1.31014393684221,-1.,-1.55322568759481));
#26392=CARTESIAN_POINT('Ctrl Pts',(-1.31014393684221,1.,-1.55322568759481));
#26393=CARTESIAN_POINT('Ctrl Pts',(-1.30824393907471,-1.,-1.54739413957183));
#26394=CARTESIAN_POINT('Ctrl Pts',(-1.30824393907471,1.,-1.54739413957183));
#26395=CARTESIAN_POINT('Ctrl Pts',(-1.30630475189553,-1.,-1.54159462645428));
#26396=CARTESIAN_POINT('Ctrl Pts',(-1.30630475189553,1.,-1.54159462645428));
#26397=CARTESIAN_POINT('Ctrl Pts',(-1.30432735639487,-1.,-1.53582981268976));
#26398=CARTESIAN_POINT('Ctrl Pts',(-1.30432735639487,1.,-1.53582981268976));
#26399=CARTESIAN_POINT('Ctrl Pts',(-1.3023106439557,-1.,-1.53009970283893));
#26400=CARTESIAN_POINT('Ctrl Pts',(-1.3023106439557,1.,-1.53009970283893));
#26401=CARTESIAN_POINT('Ctrl Pts',(-1.30024984366334,-1.,-1.5243995786107));
#26402=CARTESIAN_POINT('Ctrl Pts',(-1.30024984366334,1.,-1.5243995786107));
#26403=CARTESIAN_POINT('Ctrl Pts',(-1.29813791800757,-1.,-1.51872184912735));
#26404=CARTESIAN_POINT('Ctrl Pts',(-1.29813791800757,1.,-1.51872184912735));
#26405=CARTESIAN_POINT('Ctrl Pts',(-1.29596850710518,-1.,-1.51305994241412));
#26406=CARTESIAN_POINT('Ctrl Pts',(-1.29596850710518,1.,-1.51305994241412));
#26407=CARTESIAN_POINT('Ctrl Pts',(-1.29373841372843,-1.,-1.50741159078367));
#26408=CARTESIAN_POINT('Ctrl Pts',(-1.29373841372843,1.,-1.50741159078367));
#26409=CARTESIAN_POINT('Ctrl Pts',(-1.29145022885171,-1.,-1.50178230149764));
#26410=CARTESIAN_POINT('Ctrl Pts',(-1.29145022885171,1.,-1.50178230149764));
#26411=CARTESIAN_POINT('Ctrl Pts',(-1.28911506584232,-1.,-1.49618896881729));
#26412=CARTESIAN_POINT('Ctrl Pts',(-1.28911506584232,1.,-1.49618896881729));
#26413=CARTESIAN_POINT('Ctrl Pts',(-1.28674676116415,-1.,-1.4906522831275));
#26414=CARTESIAN_POINT('Ctrl Pts',(-1.28674676116415,1.,-1.4906522831275));
#26415=CARTESIAN_POINT('Ctrl Pts',(-1.28435533880184,-1.,-1.48518817118891));
#26416=CARTESIAN_POINT('Ctrl Pts',(-1.28435533880184,1.,-1.48518817118891));
#26417=CARTESIAN_POINT('Ctrl Pts',(-1.28194158939522,-1.,-1.47980070347102));
#26418=CARTESIAN_POINT('Ctrl Pts',(-1.28194158939522,1.,-1.47980070347102));
#26419=CARTESIAN_POINT('Ctrl Pts',(-1.27948918248524,-1.,-1.4744717526711));
#26420=CARTESIAN_POINT('Ctrl Pts',(-1.27948918248524,1.,-1.4744717526711));
#26421=CARTESIAN_POINT('Ctrl Pts',(-1.27696414831144,-1.,-1.46916035917197));
#26422=CARTESIAN_POINT('Ctrl Pts',(-1.27696414831144,1.,-1.46916035917197));
#26423=CARTESIAN_POINT('Ctrl Pts',(-1.27433119897877,-1.,-1.4638243133254));
#26424=CARTESIAN_POINT('Ctrl Pts',(-1.27433119897877,1.,-1.4638243133254));
#26425=CARTESIAN_POINT('Ctrl Pts',(-1.27156805265312,-1.,-1.45843906294725));
#26426=CARTESIAN_POINT('Ctrl Pts',(-1.27156805265312,1.,-1.45843906294725));
#26427=CARTESIAN_POINT('Ctrl Pts',(-1.26867786804854,-1.,-1.45301422764205));
#26428=CARTESIAN_POINT('Ctrl Pts',(-1.26867786804854,1.,-1.45301422764205));
#26429=CARTESIAN_POINT('Ctrl Pts',(-1.26570925118767,-1.,-1.44761985001544));
#26430=CARTESIAN_POINT('Ctrl Pts',(-1.26570925118767,1.,-1.44761985001544));
#26431=CARTESIAN_POINT('Ctrl Pts',(-1.26273903323723,-1.,-1.44236470511145));
#26432=CARTESIAN_POINT('Ctrl Pts',(-1.26273903323723,1.,-1.44236470511145));
#26433=CARTESIAN_POINT('Ctrl Pts',(-1.25983531011894,-1.,-1.43734919180719));
#26434=CARTESIAN_POINT('Ctrl Pts',(-1.25983531011894,1.,-1.43734919180719));
#26435=CARTESIAN_POINT('Ctrl Pts',(-1.25702687965744,-1.,-1.43262645609679));
#26436=CARTESIAN_POINT('Ctrl Pts',(-1.25702687965744,1.,-1.43262645609679));
#26437=CARTESIAN_POINT('Ctrl Pts',(-1.25426945222783,-1.,-1.42815938799555));
#26438=CARTESIAN_POINT('Ctrl Pts',(-1.25426945222783,1.,-1.42815938799555));
#26439=CARTESIAN_POINT('Ctrl Pts',(-1.25141455570299,-1.,-1.42378102115911));
#26440=CARTESIAN_POINT('Ctrl Pts',(-1.25141455570299,1.,-1.42378102115911));
#26441=CARTESIAN_POINT('Ctrl Pts',(-1.24824430986911,-1.,-1.41923722596421));
#26442=CARTESIAN_POINT('Ctrl Pts',(-1.24824430986911,1.,-1.41923722596421));
#26443=CARTESIAN_POINT('Ctrl Pts',(-1.24450600513278,-1.,-1.41422913175437));
#26444=CARTESIAN_POINT('Ctrl Pts',(-1.24450600513278,1.,-1.41422913175437));
#26445=CARTESIAN_POINT('Ctrl Pts',(-1.23994455029421,-1.,-1.40845295531151));
#26446=CARTESIAN_POINT('Ctrl Pts',(-1.23994455029421,1.,-1.40845295531151));
#26447=CARTESIAN_POINT('Ctrl Pts',(-1.23434087289768,-1.,-1.40164708205345));
#26448=CARTESIAN_POINT('Ctrl Pts',(-1.23434087289768,1.,-1.40164708205345));
#26449=CARTESIAN_POINT('Ctrl Pts',(-1.22752961898063,-1.,-1.39361389567257));
#26450=CARTESIAN_POINT('Ctrl Pts',(-1.22752961898063,1.,-1.39361389567257));
#26451=CARTESIAN_POINT('Ctrl Pts',(-1.21938737278853,-1.,-1.38420564525391));
#26452=CARTESIAN_POINT('Ctrl Pts',(-1.21938737278853,1.,-1.38420564525391));
#26453=CARTESIAN_POINT('Ctrl Pts',(-1.20982812923113,-1.,-1.37331915604962));
#26454=CARTESIAN_POINT('Ctrl Pts',(-1.20982812923113,1.,-1.37331915604962));
#26455=CARTESIAN_POINT('Ctrl Pts',(-1.1987959077656,-1.,-1.36088705040677));
#26456=CARTESIAN_POINT('Ctrl Pts',(-1.1987959077656,1.,-1.36088705040677));
#26457=CARTESIAN_POINT('Ctrl Pts',(-1.18625865664915,-1.,-1.34687053998157));
#26458=CARTESIAN_POINT('Ctrl Pts',(-1.18625865664915,1.,-1.34687053998157));
#26459=CARTESIAN_POINT('Ctrl Pts',(-1.17501305787994,-1.,-1.33437539344842));
#26460=CARTESIAN_POINT('Ctrl Pts',(-1.17501305787994,1.,-1.33437539344842));
#26461=CARTESIAN_POINT('Ctrl Pts',(-1.16589330092532,-1.,-1.32428080720544));
#26462=CARTESIAN_POINT('Ctrl Pts',(-1.16589330092532,1.,-1.32428080720544));
#26463=CARTESIAN_POINT('Ctrl Pts',(-1.15950888730433,-1.,-1.3172297721596));
#26464=CARTESIAN_POINT('Ctrl Pts',(-1.15950888730433,1.,-1.3172297721596));
#26465=CARTESIAN_POINT('Ctrl Pts',(-1.15624053661742,-1.,-1.31362392696033));
#26466=CARTESIAN_POINT('Ctrl Pts',(-1.15624053661742,1.,-1.31362392696033));
#26467=CARTESIAN_POINT('',(-1.34869019493419,1.,-1.73811241238545));
#26468=CARTESIAN_POINT('Ctrl Pts',(-1.34869019493419,1.,-1.73811241238545));
#26469=CARTESIAN_POINT('Ctrl Pts',(-1.34854391898145,1.,-1.73682580585819));
#26470=CARTESIAN_POINT('Ctrl Pts',(-1.34824783113158,1.,-1.73425417886255));
#26471=CARTESIAN_POINT('Ctrl Pts',(-1.3477930915247,1.,-1.73040149654497));
#26472=CARTESIAN_POINT('Ctrl Pts',(-1.34716554820013,1.,-1.72527410681298));
#26473=CARTESIAN_POINT('Ctrl Pts',(-1.34634568653586,1.,-1.7188807715095));
#26474=CARTESIAN_POINT('Ctrl Pts',(-1.34549029589563,1.,-1.71250340687011));
#26475=CARTESIAN_POINT('Ctrl Pts',(-1.34459924533783,1.,-1.70614212266676));
#26476=CARTESIAN_POINT('Ctrl Pts',(-1.34367237124322,1.,-1.69979707754221));
#26477=CARTESIAN_POINT('Ctrl Pts',(-1.34270948206139,1.,-1.6934684849664));
#26478=CARTESIAN_POINT('Ctrl Pts',(-1.34171037484673,1.,-1.68715660868602));
#26479=CARTESIAN_POINT('Ctrl Pts',(-1.3406748518516,1.,-1.68086176030308));
#26480=CARTESIAN_POINT('Ctrl Pts',(-1.33960273470372,1.,-1.67458429426126));
#26481=CARTESIAN_POINT('Ctrl Pts',(-1.33849388654458,1.,-1.66832460784078));
#26482=CARTESIAN_POINT('Ctrl Pts',(-1.33734820885331,1.,-1.66208312542073));
#26483=CARTESIAN_POINT('Ctrl Pts',(-1.33616559745217,1.,-1.65586025952651));
#26484=CARTESIAN_POINT('Ctrl Pts',(-1.33494590468003,1.,-1.64965637286843));
#26485=CARTESIAN_POINT('Ctrl Pts',(-1.33368890676554,1.,-1.64347174856007));
#26486=CARTESIAN_POINT('Ctrl Pts',(-1.33239425103694,1.,-1.6373065347505));
#26487=CARTESIAN_POINT('Ctrl Pts',(-1.33106149345618,1.,-1.63116079730887));
#26488=CARTESIAN_POINT('Ctrl Pts',(-1.32969019505665,1.,-1.62503464209777));
#26489=CARTESIAN_POINT('Ctrl Pts',(-1.32828000610448,1.,-1.61892832270723));
#26490=CARTESIAN_POINT('Ctrl Pts',(-1.32683074483365,1.,-1.61284234015762));
#26491=CARTESIAN_POINT('Ctrl Pts',(-1.32534250785794,1.,-1.6067775829097));
#26492=CARTESIAN_POINT('Ctrl Pts',(-1.32381550858266,1.,-1.600735118587));
#26493=CARTESIAN_POINT('Ctrl Pts',(-1.32224985747686,1.,-1.59471591079408));
#26494=CARTESIAN_POINT('Ctrl Pts',(-1.32064537110891,1.,-1.58872057258244));
#26495=CARTESIAN_POINT('Ctrl Pts',(-1.31900135021428,1.,-1.58274907898829));
#26496=CARTESIAN_POINT('Ctrl Pts',(-1.31731642317183,1.,-1.57680056505585));
#26497=CARTESIAN_POINT('Ctrl Pts',(-1.31558903860015,1.,-1.57087397835721));
#26498=CARTESIAN_POINT('Ctrl Pts',(-1.31381795281002,1.,-1.56496872402352));
#26499=CARTESIAN_POINT('Ctrl Pts',(-1.31200264341696,1.,-1.55908521254822));
#26500=CARTESIAN_POINT('Ctrl Pts',(-1.31014393684221,1.,-1.55322568759481));
#26501=CARTESIAN_POINT('Ctrl Pts',(-1.30824393907471,1.,-1.54739413957183));
#26502=CARTESIAN_POINT('Ctrl Pts',(-1.30630475189553,1.,-1.54159462645428));
#26503=CARTESIAN_POINT('Ctrl Pts',(-1.30432735639487,1.,-1.53582981268976));
#26504=CARTESIAN_POINT('Ctrl Pts',(-1.3023106439557,1.,-1.53009970283893));
#26505=CARTESIAN_POINT('Ctrl Pts',(-1.30024984366334,1.,-1.5243995786107));
#26506=CARTESIAN_POINT('Ctrl Pts',(-1.29813791800757,1.,-1.51872184912735));
#26507=CARTESIAN_POINT('Ctrl Pts',(-1.29596850710518,1.,-1.51305994241412));
#26508=CARTESIAN_POINT('Ctrl Pts',(-1.29373841372843,1.,-1.50741159078367));
#26509=CARTESIAN_POINT('Ctrl Pts',(-1.29145022885171,1.,-1.50178230149764));
#26510=CARTESIAN_POINT('Ctrl Pts',(-1.28911506584232,1.,-1.49618896881729));
#26511=CARTESIAN_POINT('Ctrl Pts',(-1.28674676116415,1.,-1.4906522831275));
#26512=CARTESIAN_POINT('Ctrl Pts',(-1.28435533880184,1.,-1.48518817118891));
#26513=CARTESIAN_POINT('Ctrl Pts',(-1.28194158939522,1.,-1.47980070347102));
#26514=CARTESIAN_POINT('Ctrl Pts',(-1.27948918248524,1.,-1.4744717526711));
#26515=CARTESIAN_POINT('Ctrl Pts',(-1.27696414831144,1.,-1.46916035917197));
#26516=CARTESIAN_POINT('Ctrl Pts',(-1.27433119897877,1.,-1.4638243133254));
#26517=CARTESIAN_POINT('Ctrl Pts',(-1.27156805265312,1.,-1.45843906294725));
#26518=CARTESIAN_POINT('Ctrl Pts',(-1.26867786804854,1.,-1.45301422764205));
#26519=CARTESIAN_POINT('Ctrl Pts',(-1.26570925118767,1.,-1.44761985001544));
#26520=CARTESIAN_POINT('Ctrl Pts',(-1.26273903323723,1.,-1.44236470511145));
#26521=CARTESIAN_POINT('Ctrl Pts',(-1.25983531011894,1.,-1.43734919180719));
#26522=CARTESIAN_POINT('Ctrl Pts',(-1.25702687965744,1.,-1.43262645609679));
#26523=CARTESIAN_POINT('Ctrl Pts',(-1.25426945222783,1.,-1.42815938799555));
#26524=CARTESIAN_POINT('Ctrl Pts',(-1.25141455570299,1.,-1.42378102115911));
#26525=CARTESIAN_POINT('Ctrl Pts',(-1.24824430986911,1.,-1.41923722596421));
#26526=CARTESIAN_POINT('Ctrl Pts',(-1.24450600513278,1.,-1.41422913175437));
#26527=CARTESIAN_POINT('Ctrl Pts',(-1.23994455029421,1.,-1.40845295531151));
#26528=CARTESIAN_POINT('Ctrl Pts',(-1.23434087289768,1.,-1.40164708205345));
#26529=CARTESIAN_POINT('Ctrl Pts',(-1.22752961898063,1.,-1.39361389567257));
#26530=CARTESIAN_POINT('Ctrl Pts',(-1.21938737278853,1.,-1.38420564525391));
#26531=CARTESIAN_POINT('Ctrl Pts',(-1.20982812923113,1.,-1.37331915604962));
#26532=CARTESIAN_POINT('Ctrl Pts',(-1.1987959077656,1.,-1.36088705040677));
#26533=CARTESIAN_POINT('Ctrl Pts',(-1.18625865664915,1.,-1.34687053998157));
#26534=CARTESIAN_POINT('Ctrl Pts',(-1.17501305787994,1.,-1.33437539344842));
#26535=CARTESIAN_POINT('Ctrl Pts',(-1.16589330092532,1.,-1.32428080720544));
#26536=CARTESIAN_POINT('Ctrl Pts',(-1.15950888730433,1.,-1.3172297721596));
#26537=CARTESIAN_POINT('Ctrl Pts',(-1.15624053661742,1.,-1.31362392696033));
#26538=CARTESIAN_POINT('',(-1.34869019493419,0.,-1.73811241238545));
#26539=CARTESIAN_POINT('Origin',(-1.23627494547115,0.,-1.81978687191668));
#26540=CARTESIAN_POINT('',(-1.23627494547115,1.,-1.81978687191668));
#26541=CARTESIAN_POINT('',(-1.34869019493419,1.,-1.73811241238545));
#26542=CARTESIAN_POINT('',(-1.23627494547115,0.,-1.81978687191668));
#26543=CARTESIAN_POINT('Ctrl Pts',(-0.892032620296855,-1.,-1.5055822144029));
#26544=CARTESIAN_POINT('Ctrl Pts',(-0.892032620296855,1.,-1.5055822144029));
#26545=CARTESIAN_POINT('Ctrl Pts',(-0.894452006967538,-1.,-1.50980486807181));
#26546=CARTESIAN_POINT('Ctrl Pts',(-0.894452006967538,1.,-1.50980486807181));
#26547=CARTESIAN_POINT('Ctrl Pts',(-0.89918504749193,-1.,-1.51805569591479));
#26548=CARTESIAN_POINT('Ctrl Pts',(-0.89918504749193,1.,-1.51805569591479));
#26549=CARTESIAN_POINT('Ctrl Pts',(-0.905967409640499,-1.,-1.52984849890434));
#26550=CARTESIAN_POINT('Ctrl Pts',(-0.905967409640499,1.,-1.52984849890434));
#26551=CARTESIAN_POINT('Ctrl Pts',(-0.91437591904658,-1.,-1.54440491152808));
#26552=CARTESIAN_POINT('Ctrl Pts',(-0.91437591904658,1.,-1.54440491152808));
#26553=CARTESIAN_POINT('Ctrl Pts',(-0.923832188966322,-1.,-1.56065988582509));
#26554=CARTESIAN_POINT('Ctrl Pts',(-0.923832188966322,1.,-1.56065988582509));
#26555=CARTESIAN_POINT('Ctrl Pts',(-0.932246680128849,-1.,-1.57499388385561));
#26556=CARTESIAN_POINT('Ctrl Pts',(-0.932246680128849,1.,-1.57499388385561));
#26557=CARTESIAN_POINT('Ctrl Pts',(-0.939646377909319,-1.,-1.58744937489796));
#26558=CARTESIAN_POINT('Ctrl Pts',(-0.939646377909319,1.,-1.58744937489796));
#26559=CARTESIAN_POINT('Ctrl Pts',(-0.946078063325796,-1.,-1.59810042045408));
#26560=CARTESIAN_POINT('Ctrl Pts',(-0.946078063325796,1.,-1.59810042045408));
#26561=CARTESIAN_POINT('Ctrl Pts',(-0.951613284361248,-1.,-1.60706069897794));
#26562=CARTESIAN_POINT('Ctrl Pts',(-0.951613284361248,1.,-1.60706069897794));
#26563=CARTESIAN_POINT('Ctrl Pts',(-0.956354422921573,-1.,-1.61449324337233));
#26564=CARTESIAN_POINT('Ctrl Pts',(-0.956354422921573,1.,-1.61449324337233));
#26565=CARTESIAN_POINT('Ctrl Pts',(-0.960438326099958,-1.,-1.62061638139929));
#26566=CARTESIAN_POINT('Ctrl Pts',(-0.960438326099958,1.,-1.62061638139929));
#26567=CARTESIAN_POINT('Ctrl Pts',(-0.964046107037821,-1.,-1.6257193066974));
#26568=CARTESIAN_POINT('Ctrl Pts',(-0.964046107037821,1.,-1.6257193066974));
#26569=CARTESIAN_POINT('Ctrl Pts',(-0.967387853228041,-1.,-1.63013849959083));
#26570=CARTESIAN_POINT('Ctrl Pts',(-0.967387853228041,1.,-1.63013849959083));
#26571=CARTESIAN_POINT('Ctrl Pts',(-0.970669715996356,-1.,-1.63420665729609));
#26572=CARTESIAN_POINT('Ctrl Pts',(-0.970669715996356,1.,-1.63420665729609));
#26573=CARTESIAN_POINT('Ctrl Pts',(-0.974066058287501,-1.,-1.63820952658157));
#26574=CARTESIAN_POINT('Ctrl Pts',(-0.974066058287501,1.,-1.63820952658157));
#26575=CARTESIAN_POINT('Ctrl Pts',(-0.977689794120297,-1.,-1.64233990826831));
#26576=CARTESIAN_POINT('Ctrl Pts',(-0.977689794120297,1.,-1.64233990826831));
#26577=CARTESIAN_POINT('Ctrl Pts',(-0.981562530940574,-1.,-1.64665139190834));
#26578=CARTESIAN_POINT('Ctrl Pts',(-0.981562530940574,1.,-1.64665139190834));
#26579=CARTESIAN_POINT('Ctrl Pts',(-0.985642622921626,-1.,-1.6511001661277));
#26580=CARTESIAN_POINT('Ctrl Pts',(-0.985642622921626,1.,-1.6511001661277));
#26581=CARTESIAN_POINT('Ctrl Pts',(-0.98985562785445,-1.,-1.65559044289746));
#26582=CARTESIAN_POINT('Ctrl Pts',(-0.98985562785445,1.,-1.65559044289746));
#26583=CARTESIAN_POINT('Ctrl Pts',(-0.994121836661116,-1.,-1.66001553809916));
#26584=CARTESIAN_POINT('Ctrl Pts',(-0.994121836661116,1.,-1.66001553809916));
#26585=CARTESIAN_POINT('Ctrl Pts',(-0.998389654952317,-1.,-1.66430758030304));
#26586=CARTESIAN_POINT('Ctrl Pts',(-0.998389654952317,1.,-1.66430758030304));
#26587=CARTESIAN_POINT('Ctrl Pts',(-1.00265091003682,-1.,-1.66846059277231));
#26588=CARTESIAN_POINT('Ctrl Pts',(-1.00265091003682,1.,-1.66846059277231));
#26589=CARTESIAN_POINT('Ctrl Pts',(-1.00692206696387,-1.,-1.67250335383248));
#26590=CARTESIAN_POINT('Ctrl Pts',(-1.00692206696387,1.,-1.67250335383248));
#26591=CARTESIAN_POINT('Ctrl Pts',(-1.01123236493507,-1.,-1.67648246776457));
#26592=CARTESIAN_POINT('Ctrl Pts',(-1.01123236493507,1.,-1.67648246776457));
#26593=CARTESIAN_POINT('Ctrl Pts',(-1.01561026162787,-1.,-1.6804428989482));
#26594=CARTESIAN_POINT('Ctrl Pts',(-1.01561026162787,1.,-1.6804428989482));
#26595=CARTESIAN_POINT('Ctrl Pts',(-1.02006795074222,-1.,-1.68440578021739));
#26596=CARTESIAN_POINT('Ctrl Pts',(-1.02006795074222,1.,-1.68440578021739));
#26597=CARTESIAN_POINT('Ctrl Pts',(-1.02460180535272,-1.,-1.68836910178475));
#26598=CARTESIAN_POINT('Ctrl Pts',(-1.02460180535272,1.,-1.68836910178475));
#26599=CARTESIAN_POINT('Ctrl Pts',(-1.02919977579155,-1.,-1.69231840863471));
#26600=CARTESIAN_POINT('Ctrl Pts',(-1.02919977579155,1.,-1.69231840863471));
#26601=CARTESIAN_POINT('Ctrl Pts',(-1.03384646003587,-1.,-1.69623414782769));
#26602=CARTESIAN_POINT('Ctrl Pts',(-1.03384646003587,1.,-1.69623414782769));
#26603=CARTESIAN_POINT('Ctrl Pts',(-1.03852922490782,-1.,-1.70010052930951));
#26604=CARTESIAN_POINT('Ctrl Pts',(-1.03852922490782,1.,-1.70010052930951));
#26605=CARTESIAN_POINT('Ctrl Pts',(-1.04324363334546,-1.,-1.70391338707969));
#26606=CARTESIAN_POINT('Ctrl Pts',(-1.04324363334546,1.,-1.70391338707969));
#26607=CARTESIAN_POINT('Ctrl Pts',(-1.0479908540499,-1.,-1.70767646263641));
#26608=CARTESIAN_POINT('Ctrl Pts',(-1.0479908540499,1.,-1.70767646263641));
#26609=CARTESIAN_POINT('Ctrl Pts',(-1.05277517202854,-1.,-1.71139783543986));
#26610=CARTESIAN_POINT('Ctrl Pts',(-1.05277517202854,1.,-1.71139783543986));
#26611=CARTESIAN_POINT('Ctrl Pts',(-1.05760163192481,-1.,-1.71508654427022));
#26612=CARTESIAN_POINT('Ctrl Pts',(-1.05760163192481,1.,-1.71508654427022));
#26613=CARTESIAN_POINT('Ctrl Pts',(-1.0624732468065,-1.,-1.71874858456908));
#26614=CARTESIAN_POINT('Ctrl Pts',(-1.0624732468065,1.,-1.71874858456908));
#26615=CARTESIAN_POINT('Ctrl Pts',(-1.06738966975463,-1.,-1.72238500928456));
#26616=CARTESIAN_POINT('Ctrl Pts',(-1.06738966975463,1.,-1.72238500928456));
#26617=CARTESIAN_POINT('Ctrl Pts',(-1.07234866990252,-1.,-1.72599406198489));
#26618=CARTESIAN_POINT('Ctrl Pts',(-1.07234866990252,1.,-1.72599406198489));
#26619=CARTESIAN_POINT('Ctrl Pts',(-1.0773470373727,-1.,-1.72957248977424));
#26620=CARTESIAN_POINT('Ctrl Pts',(-1.0773470373727,1.,-1.72957248977424));
#26621=CARTESIAN_POINT('Ctrl Pts',(-1.08238162784749,-1.,-1.73311705663407));
#26622=CARTESIAN_POINT('Ctrl Pts',(-1.08238162784749,1.,-1.73311705663407));
#26623=CARTESIAN_POINT('Ctrl Pts',(-1.08745056285429,-1.,-1.73662628326093));
#26624=CARTESIAN_POINT('Ctrl Pts',(-1.08745056285429,1.,-1.73662628326093));
#26625=CARTESIAN_POINT('Ctrl Pts',(-1.09255329056496,-1.,-1.74010053962252));
#26626=CARTESIAN_POINT('Ctrl Pts',(-1.09255329056496,1.,-1.74010053962252));
#26627=CARTESIAN_POINT('Ctrl Pts',(-1.09768999241229,-1.,-1.74354119236212));
#26628=CARTESIAN_POINT('Ctrl Pts',(-1.09768999241229,1.,-1.74354119236212));
#26629=CARTESIAN_POINT('Ctrl Pts',(-1.10286118991144,-1.,-1.74695004214924));
#26630=CARTESIAN_POINT('Ctrl Pts',(-1.10286118991144,1.,-1.74695004214924));
#26631=CARTESIAN_POINT('Ctrl Pts',(-1.10806728183003,-1.,-1.75032866075914));
#26632=CARTESIAN_POINT('Ctrl Pts',(-1.10806728183003,1.,-1.75032866075914));
#26633=CARTESIAN_POINT('Ctrl Pts',(-1.11330807582542,-1.,-1.75367772094617));
#26634=CARTESIAN_POINT('Ctrl Pts',(-1.11330807582542,1.,-1.75367772094617));
#26635=CARTESIAN_POINT('Ctrl Pts',(-1.11858293216752,-1.,-1.75699720772089));
#26636=CARTESIAN_POINT('Ctrl Pts',(-1.11858293216752,1.,-1.75699720772089));
#26637=CARTESIAN_POINT('Ctrl Pts',(-1.12389096855078,-1.,-1.76028671825084));
#26638=CARTESIAN_POINT('Ctrl Pts',(-1.12389096855078,1.,-1.76028671825084));
#26639=CARTESIAN_POINT('Ctrl Pts',(-1.12923123555076,-1.,-1.76354571966171));
#26640=CARTESIAN_POINT('Ctrl Pts',(-1.12923123555076,1.,-1.76354571966171));
#26641=CARTESIAN_POINT('Ctrl Pts',(-1.13460291804635,-1.,-1.76677384551883));
#26642=CARTESIAN_POINT('Ctrl Pts',(-1.13460291804635,1.,-1.76677384551883));
#26643=CARTESIAN_POINT('Ctrl Pts',(-1.14000548337,-1.,-1.76997111386806));
#26644=CARTESIAN_POINT('Ctrl Pts',(-1.14000548337,1.,-1.76997111386806));
#26645=CARTESIAN_POINT('Ctrl Pts',(-1.14543858226948,-1.,-1.77313777896234));
#26646=CARTESIAN_POINT('Ctrl Pts',(-1.14543858226948,1.,-1.77313777896234));
#26647=CARTESIAN_POINT('Ctrl Pts',(-1.15090197841531,-1.,-1.77627422557034));
#26648=CARTESIAN_POINT('Ctrl Pts',(-1.15090197841531,1.,-1.77627422557034));
#26649=CARTESIAN_POINT('Ctrl Pts',(-1.15639547194689,-1.,-1.77938085564261));
#26650=CARTESIAN_POINT('Ctrl Pts',(-1.15639547194689,1.,-1.77938085564261));
#26651=CARTESIAN_POINT('Ctrl Pts',(-1.16191881298458,-1.,-1.78245795880949));
#26652=CARTESIAN_POINT('Ctrl Pts',(-1.16191881298458,1.,-1.78245795880949));
#26653=CARTESIAN_POINT('Ctrl Pts',(-1.16747166312239,-1.,-1.78550566040349));
#26654=CARTESIAN_POINT('Ctrl Pts',(-1.16747166312239,1.,-1.78550566040349));
#26655=CARTESIAN_POINT('Ctrl Pts',(-1.17305363177265,-1.,-1.78852398877523));
#26656=CARTESIAN_POINT('Ctrl Pts',(-1.17305363177265,1.,-1.78852398877523));
#26657=CARTESIAN_POINT('Ctrl Pts',(-1.17866429440781,-1.,-1.79151291552646));
#26658=CARTESIAN_POINT('Ctrl Pts',(-1.17866429440781,1.,-1.79151291552646));
#26659=CARTESIAN_POINT('Ctrl Pts',(-1.18430321697471,-1.,-1.79447240321572));
#26660=CARTESIAN_POINT('Ctrl Pts',(-1.18430321697471,1.,-1.79447240321572));
#26661=CARTESIAN_POINT('Ctrl Pts',(-1.1899699793456,-1.,-1.79740245923649));
#26662=CARTESIAN_POINT('Ctrl Pts',(-1.1899699793456,1.,-1.79740245923649));
#26663=CARTESIAN_POINT('Ctrl Pts',(-1.19566418930405,-1.,-1.80030314370121));
#26664=CARTESIAN_POINT('Ctrl Pts',(-1.19566418930405,1.,-1.80030314370121));
#26665=CARTESIAN_POINT('Ctrl Pts',(-1.2013854893912,-1.,-1.8031745483882));
#26666=CARTESIAN_POINT('Ctrl Pts',(-1.2013854893912,1.,-1.8031745483882));
#26667=CARTESIAN_POINT('Ctrl Pts',(-1.20713356605519,-1.,-1.80601678480772));
#26668=CARTESIAN_POINT('Ctrl Pts',(-1.20713356605519,1.,-1.80601678480772));
#26669=CARTESIAN_POINT('Ctrl Pts',(-1.2129081570818,-1.,-1.80882996916931));
#26670=CARTESIAN_POINT('Ctrl Pts',(-1.2129081570818,1.,-1.80882996916931));
#26671=CARTESIAN_POINT('Ctrl Pts',(-1.2187090610323,-1.,-1.81161420806172));
#26672=CARTESIAN_POINT('Ctrl Pts',(-1.2187090610323,1.,-1.81161420806172));
#26673=CARTESIAN_POINT('Ctrl Pts',(-1.22453613304507,-1.,-1.81436959209778));
#26674=CARTESIAN_POINT('Ctrl Pts',(-1.22453613304507,1.,-1.81436959209778));
#26675=CARTESIAN_POINT('Ctrl Pts',(-1.22921864890975,-1.,-1.81655087183054));
#26676=CARTESIAN_POINT('Ctrl Pts',(-1.22921864890975,1.,-1.81655087183054));
#26677=CARTESIAN_POINT('Ctrl Pts',(-1.23274224526804,-1.,-1.81817389920914));
#26678=CARTESIAN_POINT('Ctrl Pts',(-1.23274224526804,1.,-1.81817389920914));
#26679=CARTESIAN_POINT('Ctrl Pts',(-1.23509651170384,-1.,-1.81925017193531));
#26680=CARTESIAN_POINT('Ctrl Pts',(-1.23509651170384,1.,-1.81925017193531));
#26681=CARTESIAN_POINT('Ctrl Pts',(-1.23627494547115,-1.,-1.81978687191668));
#26682=CARTESIAN_POINT('Ctrl Pts',(-1.23627494547115,1.,-1.81978687191668));
#26683=CARTESIAN_POINT('',(-0.892032620296855,1.,-1.5055822144029));
#26684=CARTESIAN_POINT('Ctrl Pts',(-0.892032620296855,1.,-1.5055822144029));
#26685=CARTESIAN_POINT('Ctrl Pts',(-0.894452006967538,1.,-1.50980486807181));
#26686=CARTESIAN_POINT('Ctrl Pts',(-0.89918504749193,1.,-1.51805569591479));
#26687=CARTESIAN_POINT('Ctrl Pts',(-0.905967409640499,1.,-1.52984849890434));
#26688=CARTESIAN_POINT('Ctrl Pts',(-0.91437591904658,1.,-1.54440491152808));
#26689=CARTESIAN_POINT('Ctrl Pts',(-0.923832188966322,1.,-1.56065988582509));
#26690=CARTESIAN_POINT('Ctrl Pts',(-0.932246680128849,1.,-1.57499388385561));
#26691=CARTESIAN_POINT('Ctrl Pts',(-0.939646377909319,1.,-1.58744937489796));
#26692=CARTESIAN_POINT('Ctrl Pts',(-0.946078063325796,1.,-1.59810042045408));
#26693=CARTESIAN_POINT('Ctrl Pts',(-0.951613284361248,1.,-1.60706069897794));
#26694=CARTESIAN_POINT('Ctrl Pts',(-0.956354422921573,1.,-1.61449324337233));
#26695=CARTESIAN_POINT('Ctrl Pts',(-0.960438326099958,1.,-1.62061638139929));
#26696=CARTESIAN_POINT('Ctrl Pts',(-0.964046107037821,1.,-1.6257193066974));
#26697=CARTESIAN_POINT('Ctrl Pts',(-0.967387853228041,1.,-1.63013849959083));
#26698=CARTESIAN_POINT('Ctrl Pts',(-0.970669715996356,1.,-1.63420665729609));
#26699=CARTESIAN_POINT('Ctrl Pts',(-0.974066058287501,1.,-1.63820952658157));
#26700=CARTESIAN_POINT('Ctrl Pts',(-0.977689794120297,1.,-1.64233990826831));
#26701=CARTESIAN_POINT('Ctrl Pts',(-0.981562530940574,1.,-1.64665139190834));
#26702=CARTESIAN_POINT('Ctrl Pts',(-0.985642622921626,1.,-1.6511001661277));
#26703=CARTESIAN_POINT('Ctrl Pts',(-0.98985562785445,1.,-1.65559044289746));
#26704=CARTESIAN_POINT('Ctrl Pts',(-0.994121836661116,1.,-1.66001553809916));
#26705=CARTESIAN_POINT('Ctrl Pts',(-0.998389654952317,1.,-1.66430758030304));
#26706=CARTESIAN_POINT('Ctrl Pts',(-1.00265091003682,1.,-1.66846059277231));
#26707=CARTESIAN_POINT('Ctrl Pts',(-1.00692206696387,1.,-1.67250335383248));
#26708=CARTESIAN_POINT('Ctrl Pts',(-1.01123236493507,1.,-1.67648246776457));
#26709=CARTESIAN_POINT('Ctrl Pts',(-1.01561026162787,1.,-1.6804428989482));
#26710=CARTESIAN_POINT('Ctrl Pts',(-1.02006795074222,1.,-1.68440578021739));
#26711=CARTESIAN_POINT('Ctrl Pts',(-1.02460180535272,1.,-1.68836910178475));
#26712=CARTESIAN_POINT('Ctrl Pts',(-1.02919977579155,1.,-1.69231840863471));
#26713=CARTESIAN_POINT('Ctrl Pts',(-1.03384646003587,1.,-1.69623414782769));
#26714=CARTESIAN_POINT('Ctrl Pts',(-1.03852922490782,1.,-1.70010052930951));
#26715=CARTESIAN_POINT('Ctrl Pts',(-1.04324363334546,1.,-1.70391338707969));
#26716=CARTESIAN_POINT('Ctrl Pts',(-1.0479908540499,1.,-1.70767646263641));
#26717=CARTESIAN_POINT('Ctrl Pts',(-1.05277517202854,1.,-1.71139783543986));
#26718=CARTESIAN_POINT('Ctrl Pts',(-1.05760163192481,1.,-1.71508654427022));
#26719=CARTESIAN_POINT('Ctrl Pts',(-1.0624732468065,1.,-1.71874858456908));
#26720=CARTESIAN_POINT('Ctrl Pts',(-1.06738966975463,1.,-1.72238500928456));
#26721=CARTESIAN_POINT('Ctrl Pts',(-1.07234866990252,1.,-1.72599406198489));
#26722=CARTESIAN_POINT('Ctrl Pts',(-1.0773470373727,1.,-1.72957248977424));
#26723=CARTESIAN_POINT('Ctrl Pts',(-1.08238162784749,1.,-1.73311705663407));
#26724=CARTESIAN_POINT('Ctrl Pts',(-1.08745056285429,1.,-1.73662628326093));
#26725=CARTESIAN_POINT('Ctrl Pts',(-1.09255329056496,1.,-1.74010053962252));
#26726=CARTESIAN_POINT('Ctrl Pts',(-1.09768999241229,1.,-1.74354119236212));
#26727=CARTESIAN_POINT('Ctrl Pts',(-1.10286118991144,1.,-1.74695004214924));
#26728=CARTESIAN_POINT('Ctrl Pts',(-1.10806728183003,1.,-1.75032866075914));
#26729=CARTESIAN_POINT('Ctrl Pts',(-1.11330807582542,1.,-1.75367772094617));
#26730=CARTESIAN_POINT('Ctrl Pts',(-1.11858293216752,1.,-1.75699720772089));
#26731=CARTESIAN_POINT('Ctrl Pts',(-1.12389096855078,1.,-1.76028671825084));
#26732=CARTESIAN_POINT('Ctrl Pts',(-1.12923123555076,1.,-1.76354571966171));
#26733=CARTESIAN_POINT('Ctrl Pts',(-1.13460291804635,1.,-1.76677384551883));
#26734=CARTESIAN_POINT('Ctrl Pts',(-1.14000548337,1.,-1.76997111386806));
#26735=CARTESIAN_POINT('Ctrl Pts',(-1.14543858226948,1.,-1.77313777896234));
#26736=CARTESIAN_POINT('Ctrl Pts',(-1.15090197841531,1.,-1.77627422557034));
#26737=CARTESIAN_POINT('Ctrl Pts',(-1.15639547194689,1.,-1.77938085564261));
#26738=CARTESIAN_POINT('Ctrl Pts',(-1.16191881298458,1.,-1.78245795880949));
#26739=CARTESIAN_POINT('Ctrl Pts',(-1.16747166312239,1.,-1.78550566040349));
#26740=CARTESIAN_POINT('Ctrl Pts',(-1.17305363177265,1.,-1.78852398877523));
#26741=CARTESIAN_POINT('Ctrl Pts',(-1.17866429440781,1.,-1.79151291552646));
#26742=CARTESIAN_POINT('Ctrl Pts',(-1.18430321697471,1.,-1.79447240321572));
#26743=CARTESIAN_POINT('Ctrl Pts',(-1.1899699793456,1.,-1.79740245923649));
#26744=CARTESIAN_POINT('Ctrl Pts',(-1.19566418930405,1.,-1.80030314370121));
#26745=CARTESIAN_POINT('Ctrl Pts',(-1.2013854893912,1.,-1.8031745483882));
#26746=CARTESIAN_POINT('Ctrl Pts',(-1.20713356605519,1.,-1.80601678480772));
#26747=CARTESIAN_POINT('Ctrl Pts',(-1.2129081570818,1.,-1.80882996916931));
#26748=CARTESIAN_POINT('Ctrl Pts',(-1.2187090610323,1.,-1.81161420806172));
#26749=CARTESIAN_POINT('Ctrl Pts',(-1.22453613304507,1.,-1.81436959209778));
#26750=CARTESIAN_POINT('Ctrl Pts',(-1.22921864890975,1.,-1.81655087183054));
#26751=CARTESIAN_POINT('Ctrl Pts',(-1.23274224526804,1.,-1.81817389920914));
#26752=CARTESIAN_POINT('Ctrl Pts',(-1.23509651170384,1.,-1.81925017193531));
#26753=CARTESIAN_POINT('Ctrl Pts',(-1.23627494547115,1.,-1.81978687191668));
#26754=CARTESIAN_POINT('',(-0.892032620296856,0.,-1.5055822144029));
#26755=CARTESIAN_POINT('Origin',(0.,0.,0.));
#26756=CARTESIAN_POINT('',(-0.693717979106305,1.,-1.60662857109684));
#26757=CARTESIAN_POINT('Origin',(0.,1.,0.));
#26758=CARTESIAN_POINT('',(-0.693717979106306,0.,-1.60662857109684));
#26759=CARTESIAN_POINT('Ctrl Pts',(-0.745574324794401,-1.,-2.0698113262342));
#26760=CARTESIAN_POINT('Ctrl Pts',(-0.745574324794401,1.,-2.0698113262342));
#26761=CARTESIAN_POINT('Ctrl Pts',(-0.745832791378367,-1.,-2.06854248895728));
#26762=CARTESIAN_POINT('Ctrl Pts',(-0.745832791378367,1.,-2.06854248895728));
#26763=CARTESIAN_POINT('Ctrl Pts',(-0.7463458715442,-1.,-2.06600523016815));
#26764=CARTESIAN_POINT('Ctrl Pts',(-0.7463458715442,1.,-2.06600523016815));
#26765=CARTESIAN_POINT('Ctrl Pts',(-0.747103932787919,-1.,-2.06220058927826));
#26766=CARTESIAN_POINT('Ctrl Pts',(-0.747103932787919,1.,-2.06220058927826));
#26767=CARTESIAN_POINT('Ctrl Pts',(-0.748091554183802,-1.,-2.05713023031006));
#26768=CARTESIAN_POINT('Ctrl Pts',(-0.748091554183802,1.,-2.05713023031006));
#26769=CARTESIAN_POINT('Ctrl Pts',(-0.749287468665046,-1.,-2.05079645592154));
#26770=CARTESIAN_POINT('Ctrl Pts',(-0.749287468665046,1.,-2.05079645592154));
#26771=CARTESIAN_POINT('Ctrl Pts',(-0.750444657875576,-1.,-2.04446689147979));
#26772=CARTESIAN_POINT('Ctrl Pts',(-0.750444657875576,1.,-2.04446689147979));
#26773=CARTESIAN_POINT('Ctrl Pts',(-0.751562963361115,-1.,-2.03814160092099));
#26774=CARTESIAN_POINT('Ctrl Pts',(-0.751562963361115,1.,-2.03814160092099));
#26775=CARTESIAN_POINT('Ctrl Pts',(-0.752642180487211,-1.,-2.03182068456221));
#26776=CARTESIAN_POINT('Ctrl Pts',(-0.752642180487211,1.,-2.03182068456221));
#26777=CARTESIAN_POINT('Ctrl Pts',(-0.753682061112768,-1.,-2.02550428623313));
#26778=CARTESIAN_POINT('Ctrl Pts',(-0.753682061112768,1.,-2.02550428623313));
#26779=CARTESIAN_POINT('Ctrl Pts',(-0.754682330722816,-1.,-2.01919259405809));
#26780=CARTESIAN_POINT('Ctrl Pts',(-0.754682330722816,1.,-2.01919259405809));
#26781=CARTESIAN_POINT('Ctrl Pts',(-0.755642704957865,-1.,-2.01288584328084));
#26782=CARTESIAN_POINT('Ctrl Pts',(-0.755642704957865,1.,-2.01288584328084));
#26783=CARTESIAN_POINT('Ctrl Pts',(-0.75656290464667,-1.,-2.0065843158773));
#26784=CARTESIAN_POINT('Ctrl Pts',(-0.75656290464667,1.,-2.0065843158773));
#26785=CARTESIAN_POINT('Ctrl Pts',(-0.757442676862724,-1.,-2.00028834739178));
#26786=CARTESIAN_POINT('Ctrl Pts',(-0.757442676862724,1.,-2.00028834739178));
#26787=CARTESIAN_POINT('Ctrl Pts',(-0.758281796766761,-1.,-1.99399831098817));
#26788=CARTESIAN_POINT('Ctrl Pts',(-0.758281796766761,1.,-1.99399831098817));
#26789=CARTESIAN_POINT('Ctrl Pts',(-0.759080037802488,-1.,-1.98771456680874));
#26790=CARTESIAN_POINT('Ctrl Pts',(-0.759080037802488,1.,-1.98771456680874));
#26791=CARTESIAN_POINT('Ctrl Pts',(-0.75983714745219,-1.,-1.98143741418172));
#26792=CARTESIAN_POINT('Ctrl Pts',(-0.75983714745219,1.,-1.98143741418172));
#26793=CARTESIAN_POINT('Ctrl Pts',(-0.760552825409757,-1.,-1.97516705321494));
#26794=CARTESIAN_POINT('Ctrl Pts',(-0.760552825409757,1.,-1.97516705321494));
#26795=CARTESIAN_POINT('Ctrl Pts',(-0.76122669048382,-1.,-1.96890351582499));
#26796=CARTESIAN_POINT('Ctrl Pts',(-0.76122669048382,1.,-1.96890351582499));
#26797=CARTESIAN_POINT('Ctrl Pts',(-0.761858300014423,-1.,-1.96264672744186));
#26798=CARTESIAN_POINT('Ctrl Pts',(-0.761858300014423,1.,-1.96264672744186));
#26799=CARTESIAN_POINT('Ctrl Pts',(-0.762447203806179,-1.,-1.95639665309869));
#26800=CARTESIAN_POINT('Ctrl Pts',(-0.762447203806179,1.,-1.95639665309869));
#26801=CARTESIAN_POINT('Ctrl Pts',(-0.762992990878769,-1.,-1.95015342590024));
#26802=CARTESIAN_POINT('Ctrl Pts',(-0.762992990878769,1.,-1.95015342590024));
#26803=CARTESIAN_POINT('Ctrl Pts',(-0.763495333538629,-1.,-1.9439174661764));
#26804=CARTESIAN_POINT('Ctrl Pts',(-0.763495333538629,1.,-1.9439174661764));
#26805=CARTESIAN_POINT('Ctrl Pts',(-0.763954049121458,-1.,-1.93768964875886));
#26806=CARTESIAN_POINT('Ctrl Pts',(-0.763954049121458,1.,-1.93768964875886));
#26807=CARTESIAN_POINT('Ctrl Pts',(-0.764369010673941,-1.,-1.93147105496382));
#26808=CARTESIAN_POINT('Ctrl Pts',(-0.764369010673941,1.,-1.93147105496382));
#26809=CARTESIAN_POINT('Ctrl Pts',(-0.764740025488211,-1.,-1.92526263537048));
#26810=CARTESIAN_POINT('Ctrl Pts',(-0.764740025488211,1.,-1.92526263537048));
#26811=CARTESIAN_POINT('Ctrl Pts',(-0.765066729667088,-1.,-1.91906491634196));
#26812=CARTESIAN_POINT('Ctrl Pts',(-0.765066729667088,1.,-1.91906491634196));
#26813=CARTESIAN_POINT('Ctrl Pts',(-0.765348465884722,-1.,-1.91287765805169));
#26814=CARTESIAN_POINT('Ctrl Pts',(-0.765348465884722,1.,-1.91287765805169));
#26815=CARTESIAN_POINT('Ctrl Pts',(-0.765584196937919,-1.,-1.90669961402356));
#26816=CARTESIAN_POINT('Ctrl Pts',(-0.765584196937919,1.,-1.90669961402356));
#26817=CARTESIAN_POINT('Ctrl Pts',(-0.765772772593386,-1.,-1.90052930393596));
#26818=CARTESIAN_POINT('Ctrl Pts',(-0.765772772593386,1.,-1.90052930393596));
#26819=CARTESIAN_POINT('Ctrl Pts',(-0.765913193856978,-1.,-1.89436577771388));
#26820=CARTESIAN_POINT('Ctrl Pts',(-0.765913193856978,1.,-1.89436577771388));
#26821=CARTESIAN_POINT('Ctrl Pts',(-0.766004837062091,-1.,-1.88820926433409));
#26822=CARTESIAN_POINT('Ctrl Pts',(-0.766004837062091,1.,-1.88820926433409));
#26823=CARTESIAN_POINT('Ctrl Pts',(-0.766047794851865,-1.,-1.88206215302561));
#26824=CARTESIAN_POINT('Ctrl Pts',(-0.766047794851865,1.,-1.88206215302561));
#26825=CARTESIAN_POINT('Ctrl Pts',(-0.766042837036744,-1.,-1.87592888967883));
#26826=CARTESIAN_POINT('Ctrl Pts',(-0.766042837036744,1.,-1.87592888967883));
#26827=CARTESIAN_POINT('Ctrl Pts',(-0.765990708546091,-1.,-1.86981398314341));
#26828=CARTESIAN_POINT('Ctrl Pts',(-0.765990708546091,1.,-1.86981398314341));
#26829=CARTESIAN_POINT('Ctrl Pts',(-0.765891519092547,-1.,-1.86372027063312));
#26830=CARTESIAN_POINT('Ctrl Pts',(-0.765891519092547,1.,-1.86372027063312));
#26831=CARTESIAN_POINT('Ctrl Pts',(-0.765744212909318,-1.,-1.85764741390394));
#26832=CARTESIAN_POINT('Ctrl Pts',(-0.765744212909318,1.,-1.85764741390394));
#26833=CARTESIAN_POINT('Ctrl Pts',(-0.765545710619062,-1.,-1.85158945130063));
#26834=CARTESIAN_POINT('Ctrl Pts',(-0.765545710619062,1.,-1.85158945130063));
#26835=CARTESIAN_POINT('Ctrl Pts',(-0.765291664862029,-1.,-1.84553698875924));
#26836=CARTESIAN_POINT('Ctrl Pts',(-0.765291664862029,1.,-1.84553698875924));
#26837=CARTESIAN_POINT('Ctrl Pts',(-0.764978057881737,-1.,-1.83948181064835));
#26838=CARTESIAN_POINT('Ctrl Pts',(-0.764978057881737,1.,-1.83948181064835));
#26839=CARTESIAN_POINT('Ctrl Pts',(-0.764602549687853,-1.,-1.83342077227142));
#26840=CARTESIAN_POINT('Ctrl Pts',(-0.764602549687853,1.,-1.83342077227142));
#26841=CARTESIAN_POINT('Ctrl Pts',(-0.764165902605995,-1.,-1.82735991200065));
#26842=CARTESIAN_POINT('Ctrl Pts',(-0.764165902605995,1.,-1.82735991200065));
#26843=CARTESIAN_POINT('Ctrl Pts',(-0.763673465462726,-1.,-1.82131873145266));
#26844=CARTESIAN_POINT('Ctrl Pts',(-0.763673465462726,1.,-1.82131873145266));
#26845=CARTESIAN_POINT('Ctrl Pts',(-0.763132003836634,-1.,-1.8153211840553));
#26846=CARTESIAN_POINT('Ctrl Pts',(-0.763132003836634,1.,-1.8153211840553));
#26847=CARTESIAN_POINT('Ctrl Pts',(-0.762546129463938,-1.,-1.80938551463965));
#26848=CARTESIAN_POINT('Ctrl Pts',(-0.762546129463938,1.,-1.80938551463965));
#26849=CARTESIAN_POINT('Ctrl Pts',(-0.761915336443547,-1.,-1.80351583877342));
#26850=CARTESIAN_POINT('Ctrl Pts',(-0.761915336443547,1.,-1.80351583877342));
#26851=CARTESIAN_POINT('Ctrl Pts',(-0.761229695230558,-1.,-1.79768986997783));
#26852=CARTESIAN_POINT('Ctrl Pts',(-0.761229695230558,1.,-1.79768986997783));
#26853=CARTESIAN_POINT('Ctrl Pts',(-0.760469555880749,-1.,-1.7918581561088));
#26854=CARTESIAN_POINT('Ctrl Pts',(-0.760469555880749,1.,-1.7918581561088));
#26855=CARTESIAN_POINT('Ctrl Pts',(-0.759614401110189,-1.,-1.78596964884604));
#26856=CARTESIAN_POINT('Ctrl Pts',(-0.759614401110189,1.,-1.78596964884604));
#26857=CARTESIAN_POINT('Ctrl Pts',(-0.758650626677518,-1.,-1.77999411220945));
#26858=CARTESIAN_POINT('Ctrl Pts',(-0.758650626677518,1.,-1.77999411220945));
#26859=CARTESIAN_POINT('Ctrl Pts',(-0.757578264077029,-1.,-1.77394167108292));
#26860=CARTESIAN_POINT('Ctrl Pts',(-0.757578264077029,1.,-1.77394167108292));
#26861=CARTESIAN_POINT('Ctrl Pts',(-0.75642189602781,-1.,-1.76789396002998));
#26862=CARTESIAN_POINT('Ctrl Pts',(-0.75642189602781,1.,-1.76789396002998));
#26863=CARTESIAN_POINT('Ctrl Pts',(-0.755220979974461,-1.,-1.76197817240128));
#26864=CARTESIAN_POINT('Ctrl Pts',(-0.755220979974461,1.,-1.76197817240128));
#26865=CARTESIAN_POINT('Ctrl Pts',(-0.754009254027829,-1.,-1.75631083600019));
#26866=CARTESIAN_POINT('Ctrl Pts',(-0.754009254027829,1.,-1.75631083600019));
#26867=CARTESIAN_POINT('Ctrl Pts',(-0.752797683531314,-1.,-1.75095139468794));
#26868=CARTESIAN_POINT('Ctrl Pts',(-0.752797683531314,1.,-1.75095139468794));
#26869=CARTESIAN_POINT('Ctrl Pts',(-0.751555614164482,-1.,-1.74585086852502));
#26870=CARTESIAN_POINT('Ctrl Pts',(-0.751555614164482,1.,-1.74585086852502));
#26871=CARTESIAN_POINT('Ctrl Pts',(-0.750193435981249,-1.,-1.74080458267114));
#26872=CARTESIAN_POINT('Ctrl Pts',(-0.750193435981249,1.,-1.74080458267114));
#26873=CARTESIAN_POINT('Ctrl Pts',(-0.74858246295687,-1.,-1.7355035168033));
#26874=CARTESIAN_POINT('Ctrl Pts',(-0.74858246295687,1.,-1.7355035168033));
#26875=CARTESIAN_POINT('Ctrl Pts',(-0.746574710097752,-1.,-1.72958533647714));
#26876=CARTESIAN_POINT('Ctrl Pts',(-0.746574710097752,1.,-1.72958533647714));
#26877=CARTESIAN_POINT('Ctrl Pts',(-0.744021445433093,-1.,-1.72268229916769));
#26878=CARTESIAN_POINT('Ctrl Pts',(-0.744021445433093,1.,-1.72268229916769));
#26879=CARTESIAN_POINT('Ctrl Pts',(-0.74079516202821,-1.,-1.71447789751001));
#26880=CARTESIAN_POINT('Ctrl Pts',(-0.74079516202821,1.,-1.71447789751001));
#26881=CARTESIAN_POINT('Ctrl Pts',(-0.736799665716932,-1.,-1.70473309004249));
#26882=CARTESIAN_POINT('Ctrl Pts',(-0.736799665716932,1.,-1.70473309004249));
#26883=CARTESIAN_POINT('Ctrl Pts',(-0.731963238685357,-1.,-1.69326921972915));
#26884=CARTESIAN_POINT('Ctrl Pts',(-0.731963238685357,1.,-1.69326921972915));
#26885=CARTESIAN_POINT('Ctrl Pts',(-0.726235967982445,-1.,-1.67996158451922));
#26886=CARTESIAN_POINT('Ctrl Pts',(-0.726235967982445,1.,-1.67996158451922));
#26887=CARTESIAN_POINT('Ctrl Pts',(-0.71958543378795,-1.,-1.66472880551777));
#26888=CARTESIAN_POINT('Ctrl Pts',(-0.71958543378795,1.,-1.66472880551777));
#26889=CARTESIAN_POINT('Ctrl Pts',(-0.711993139340447,-1.,-1.64752408828442));
#26890=CARTESIAN_POINT('Ctrl Pts',(-0.711993139340447,1.,-1.64752408828442));
#26891=CARTESIAN_POINT('Ctrl Pts',(-0.705159151977294,-1.,-1.6321654166204));
#26892=CARTESIAN_POINT('Ctrl Pts',(-0.705159151977294,1.,-1.6321654166204));
#26893=CARTESIAN_POINT('Ctrl Pts',(-0.699605146398837,-1.,-1.61974673471117));
#26894=CARTESIAN_POINT('Ctrl Pts',(-0.699605146398837,1.,-1.61974673471117));
#26895=CARTESIAN_POINT('Ctrl Pts',(-0.69571209787897,-1.,-1.61106790957619));
#26896=CARTESIAN_POINT('Ctrl Pts',(-0.69571209787897,1.,-1.61106790957619));
#26897=CARTESIAN_POINT('Ctrl Pts',(-0.693717979106305,-1.,-1.60662857109684));
#26898=CARTESIAN_POINT('Ctrl Pts',(-0.693717979106305,1.,-1.60662857109684));
#26899=CARTESIAN_POINT('',(-0.745574324794401,1.,-2.0698113262342));
#26900=CARTESIAN_POINT('Ctrl Pts',(-0.745574324794401,1.,-2.0698113262342));
#26901=CARTESIAN_POINT('Ctrl Pts',(-0.745832791378367,1.,-2.06854248895728));
#26902=CARTESIAN_POINT('Ctrl Pts',(-0.7463458715442,1.,-2.06600523016815));
#26903=CARTESIAN_POINT('Ctrl Pts',(-0.747103932787919,1.,-2.06220058927826));
#26904=CARTESIAN_POINT('Ctrl Pts',(-0.748091554183802,1.,-2.05713023031006));
#26905=CARTESIAN_POINT('Ctrl Pts',(-0.749287468665046,1.,-2.05079645592154));
#26906=CARTESIAN_POINT('Ctrl Pts',(-0.750444657875576,1.,-2.04446689147979));
#26907=CARTESIAN_POINT('Ctrl Pts',(-0.751562963361115,1.,-2.03814160092099));
#26908=CARTESIAN_POINT('Ctrl Pts',(-0.752642180487211,1.,-2.03182068456221));
#26909=CARTESIAN_POINT('Ctrl Pts',(-0.753682061112768,1.,-2.02550428623313));
#26910=CARTESIAN_POINT('Ctrl Pts',(-0.754682330722816,1.,-2.01919259405809));
#26911=CARTESIAN_POINT('Ctrl Pts',(-0.755642704957865,1.,-2.01288584328084));
#26912=CARTESIAN_POINT('Ctrl Pts',(-0.75656290464667,1.,-2.0065843158773));
#26913=CARTESIAN_POINT('Ctrl Pts',(-0.757442676862724,1.,-2.00028834739178));
#26914=CARTESIAN_POINT('Ctrl Pts',(-0.758281796766761,1.,-1.99399831098817));
#26915=CARTESIAN_POINT('Ctrl Pts',(-0.759080037802488,1.,-1.98771456680874));
#26916=CARTESIAN_POINT('Ctrl Pts',(-0.75983714745219,1.,-1.98143741418172));
#26917=CARTESIAN_POINT('Ctrl Pts',(-0.760552825409757,1.,-1.97516705321494));
#26918=CARTESIAN_POINT('Ctrl Pts',(-0.76122669048382,1.,-1.96890351582499));
#26919=CARTESIAN_POINT('Ctrl Pts',(-0.761858300014423,1.,-1.96264672744186));
#26920=CARTESIAN_POINT('Ctrl Pts',(-0.762447203806179,1.,-1.95639665309869));
#26921=CARTESIAN_POINT('Ctrl Pts',(-0.762992990878769,1.,-1.95015342590024));
#26922=CARTESIAN_POINT('Ctrl Pts',(-0.763495333538629,1.,-1.9439174661764));
#26923=CARTESIAN_POINT('Ctrl Pts',(-0.763954049121458,1.,-1.93768964875886));
#26924=CARTESIAN_POINT('Ctrl Pts',(-0.764369010673941,1.,-1.93147105496382));
#26925=CARTESIAN_POINT('Ctrl Pts',(-0.764740025488211,1.,-1.92526263537048));
#26926=CARTESIAN_POINT('Ctrl Pts',(-0.765066729667088,1.,-1.91906491634196));
#26927=CARTESIAN_POINT('Ctrl Pts',(-0.765348465884722,1.,-1.91287765805169));
#26928=CARTESIAN_POINT('Ctrl Pts',(-0.765584196937919,1.,-1.90669961402356));
#26929=CARTESIAN_POINT('Ctrl Pts',(-0.765772772593386,1.,-1.90052930393596));
#26930=CARTESIAN_POINT('Ctrl Pts',(-0.765913193856978,1.,-1.89436577771388));
#26931=CARTESIAN_POINT('Ctrl Pts',(-0.766004837062091,1.,-1.88820926433409));
#26932=CARTESIAN_POINT('Ctrl Pts',(-0.766047794851865,1.,-1.88206215302561));
#26933=CARTESIAN_POINT('Ctrl Pts',(-0.766042837036744,1.,-1.87592888967883));
#26934=CARTESIAN_POINT('Ctrl Pts',(-0.765990708546091,1.,-1.86981398314341));
#26935=CARTESIAN_POINT('Ctrl Pts',(-0.765891519092547,1.,-1.86372027063312));
#26936=CARTESIAN_POINT('Ctrl Pts',(-0.765744212909318,1.,-1.85764741390394));
#26937=CARTESIAN_POINT('Ctrl Pts',(-0.765545710619062,1.,-1.85158945130063));
#26938=CARTESIAN_POINT('Ctrl Pts',(-0.765291664862029,1.,-1.84553698875924));
#26939=CARTESIAN_POINT('Ctrl Pts',(-0.764978057881737,1.,-1.83948181064835));
#26940=CARTESIAN_POINT('Ctrl Pts',(-0.764602549687853,1.,-1.83342077227142));
#26941=CARTESIAN_POINT('Ctrl Pts',(-0.764165902605995,1.,-1.82735991200065));
#26942=CARTESIAN_POINT('Ctrl Pts',(-0.763673465462726,1.,-1.82131873145266));
#26943=CARTESIAN_POINT('Ctrl Pts',(-0.763132003836634,1.,-1.8153211840553));
#26944=CARTESIAN_POINT('Ctrl Pts',(-0.762546129463938,1.,-1.80938551463965));
#26945=CARTESIAN_POINT('Ctrl Pts',(-0.761915336443547,1.,-1.80351583877342));
#26946=CARTESIAN_POINT('Ctrl Pts',(-0.761229695230558,1.,-1.79768986997783));
#26947=CARTESIAN_POINT('Ctrl Pts',(-0.760469555880749,1.,-1.7918581561088));
#26948=CARTESIAN_POINT('Ctrl Pts',(-0.759614401110189,1.,-1.78596964884604));
#26949=CARTESIAN_POINT('Ctrl Pts',(-0.758650626677518,1.,-1.77999411220945));
#26950=CARTESIAN_POINT('Ctrl Pts',(-0.757578264077029,1.,-1.77394167108292));
#26951=CARTESIAN_POINT('Ctrl Pts',(-0.75642189602781,1.,-1.76789396002998));
#26952=CARTESIAN_POINT('Ctrl Pts',(-0.755220979974461,1.,-1.76197817240128));
#26953=CARTESIAN_POINT('Ctrl Pts',(-0.754009254027829,1.,-1.75631083600019));
#26954=CARTESIAN_POINT('Ctrl Pts',(-0.752797683531314,1.,-1.75095139468794));
#26955=CARTESIAN_POINT('Ctrl Pts',(-0.751555614164482,1.,-1.74585086852502));
#26956=CARTESIAN_POINT('Ctrl Pts',(-0.750193435981249,1.,-1.74080458267114));
#26957=CARTESIAN_POINT('Ctrl Pts',(-0.74858246295687,1.,-1.7355035168033));
#26958=CARTESIAN_POINT('Ctrl Pts',(-0.746574710097752,1.,-1.72958533647714));
#26959=CARTESIAN_POINT('Ctrl Pts',(-0.744021445433093,1.,-1.72268229916769));
#26960=CARTESIAN_POINT('Ctrl Pts',(-0.74079516202821,1.,-1.71447789751001));
#26961=CARTESIAN_POINT('Ctrl Pts',(-0.736799665716932,1.,-1.70473309004249));
#26962=CARTESIAN_POINT('Ctrl Pts',(-0.731963238685357,1.,-1.69326921972915));
#26963=CARTESIAN_POINT('Ctrl Pts',(-0.726235967982445,1.,-1.67996158451922));
#26964=CARTESIAN_POINT('Ctrl Pts',(-0.71958543378795,1.,-1.66472880551777));
#26965=CARTESIAN_POINT('Ctrl Pts',(-0.711993139340447,1.,-1.64752408828442));
#26966=CARTESIAN_POINT('Ctrl Pts',(-0.705159151977294,1.,-1.6321654166204));
#26967=CARTESIAN_POINT('Ctrl Pts',(-0.699605146398837,1.,-1.61974673471117));
#26968=CARTESIAN_POINT('Ctrl Pts',(-0.69571209787897,1.,-1.61106790957619));
#26969=CARTESIAN_POINT('Ctrl Pts',(-0.693717979106305,1.,-1.60662857109684));
#26970=CARTESIAN_POINT('',(-0.745574324794401,0.,-2.0698113262342));
#26971=CARTESIAN_POINT('Origin',(-0.61342227326009,0.,-2.11275013067528));
#26972=CARTESIAN_POINT('',(-0.61342227326009,1.,-2.11275013067528));
#26973=CARTESIAN_POINT('',(-0.745574324794401,1.,-2.0698113262342));
#26974=CARTESIAN_POINT('',(-0.61342227326009,0.,-2.11275013067528));
#26975=CARTESIAN_POINT('Ctrl Pts',(-0.383122945602004,-1.,-1.7075470150345));
#26976=CARTESIAN_POINT('Ctrl Pts',(-0.383122945602004,1.,-1.7075470150345));
#26977=CARTESIAN_POINT('Ctrl Pts',(-0.384119047315542,-1.,-1.71231062891958));
#26978=CARTESIAN_POINT('Ctrl Pts',(-0.384119047315542,1.,-1.71231062891958));
#26979=CARTESIAN_POINT('Ctrl Pts',(-0.38607079032701,-1.,-1.72162022246158));
#26980=CARTESIAN_POINT('Ctrl Pts',(-0.38607079032701,1.,-1.72162022246158));
#26981=CARTESIAN_POINT('Ctrl Pts',(-0.388877023509191,-1.,-1.7349317097561));
#26982=CARTESIAN_POINT('Ctrl Pts',(-0.388877023509191,1.,-1.7349317097561));
#26983=CARTESIAN_POINT('Ctrl Pts',(-0.392375812294307,-1.,-1.75137405313962));
#26984=CARTESIAN_POINT('Ctrl Pts',(-0.392375812294307,1.,-1.75137405313962));
#26985=CARTESIAN_POINT('Ctrl Pts',(-0.39634619612042,-1.,-1.7697556004756));
#26986=CARTESIAN_POINT('Ctrl Pts',(-0.39634619612042,1.,-1.7697556004756));
#26987=CARTESIAN_POINT('Ctrl Pts',(-0.39991940378308,-1.,-1.78598826347533));
#26988=CARTESIAN_POINT('Ctrl Pts',(-0.39991940378308,1.,-1.78598826347533));
#26989=CARTESIAN_POINT('Ctrl Pts',(-0.403107976170441,-1.,-1.80012077176221));
#26990=CARTESIAN_POINT('Ctrl Pts',(-0.403107976170441,1.,-1.80012077176221));
#26991=CARTESIAN_POINT('Ctrl Pts',(-0.405933518411838,-1.,-1.81223801813988));
#26992=CARTESIAN_POINT('Ctrl Pts',(-0.405933518411838,1.,-1.81223801813988));
#26993=CARTESIAN_POINT('Ctrl Pts',(-0.408428948108533,-1.,-1.8224702267854));
#26994=CARTESIAN_POINT('Ctrl Pts',(-0.408428948108533,1.,-1.8224702267854));
#26995=CARTESIAN_POINT('Ctrl Pts',(-0.410641256301675,-1.,-1.83100408895216));
#26996=CARTESIAN_POINT('Ctrl Pts',(-0.410641256301675,1.,-1.83100408895216));
#26997=CARTESIAN_POINT('Ctrl Pts',(-0.412633125322162,-1.,-1.83808953475839));
#26998=CARTESIAN_POINT('Ctrl Pts',(-0.412633125322162,1.,-1.83808953475839));
#26999=CARTESIAN_POINT('Ctrl Pts',(-0.41448743825434,-1.,-1.8440575707371));
#27000=CARTESIAN_POINT('Ctrl Pts',(-0.41448743825434,1.,-1.8440575707371));
#27001=CARTESIAN_POINT('Ctrl Pts',(-0.416300022038864,-1.,-1.84929312929882));
#27002=CARTESIAN_POINT('Ctrl Pts',(-0.416300022038864,1.,-1.84929312929882));
#27003=CARTESIAN_POINT('Ctrl Pts',(-0.418164129143534,-1.,-1.85417632856234));
#27004=CARTESIAN_POINT('Ctrl Pts',(-0.418164129143534,1.,-1.85417632856234));
#27005=CARTESIAN_POINT('Ctrl Pts',(-0.420157287975619,-1.,-1.85903281096686));
#27006=CARTESIAN_POINT('Ctrl Pts',(-0.420157287975619,1.,-1.85903281096686));
#27007=CARTESIAN_POINT('Ctrl Pts',(-0.422327307418275,-1.,-1.86408083334028));
#27008=CARTESIAN_POINT('Ctrl Pts',(-0.422327307418275,1.,-1.86408083334028));
#27009=CARTESIAN_POINT('Ctrl Pts',(-0.424678177291359,-1.,-1.86937803944323));
#27010=CARTESIAN_POINT('Ctrl Pts',(-0.424678177291359,1.,-1.86937803944323));
#27011=CARTESIAN_POINT('Ctrl Pts',(-0.427183828519102,-1.,-1.87486989291484));
#27012=CARTESIAN_POINT('Ctrl Pts',(-0.427183828519102,1.,-1.87486989291484));
#27013=CARTESIAN_POINT('Ctrl Pts',(-0.429803062482344,-1.,-1.88044229001832));
#27014=CARTESIAN_POINT('Ctrl Pts',(-0.429803062482344,1.,-1.88044229001832));
#27015=CARTESIAN_POINT('Ctrl Pts',(-0.432493038548748,-1.,-1.88596913666793));
#27016=CARTESIAN_POINT('Ctrl Pts',(-0.432493038548748,1.,-1.88596913666793));
#27017=CARTESIAN_POINT('Ctrl Pts',(-0.435225660963383,-1.,-1.89136993975504));
#27018=CARTESIAN_POINT('Ctrl Pts',(-0.435225660963383,1.,-1.89136993975504));
#27019=CARTESIAN_POINT('Ctrl Pts',(-0.437995003948244,-1.,-1.89663648956466));
#27020=CARTESIAN_POINT('Ctrl Pts',(-0.437995003948244,1.,-1.89663648956466));
#27021=CARTESIAN_POINT('Ctrl Pts',(-0.440807833704038,-1.,-1.90180124389086));
#27022=CARTESIAN_POINT('Ctrl Pts',(-0.440807833704038,1.,-1.90180124389086));
#27023=CARTESIAN_POINT('Ctrl Pts',(-0.443677556849151,-1.,-1.90691756144898));
#27024=CARTESIAN_POINT('Ctrl Pts',(-0.443677556849151,1.,-1.90691756144898));
#27025=CARTESIAN_POINT('Ctrl Pts',(-0.446617343485711,-1.,-1.9120369998112));
#27026=CARTESIAN_POINT('Ctrl Pts',(-0.446617343485711,1.,-1.9120369998112));
#27027=CARTESIAN_POINT('Ctrl Pts',(-0.449632260106662,-1.,-1.91718342555755));
#27028=CARTESIAN_POINT('Ctrl Pts',(-0.449632260106662,1.,-1.91718342555755));
#27029=CARTESIAN_POINT('Ctrl Pts',(-0.452719478359432,-1.,-1.92235380648502));
#27030=CARTESIAN_POINT('Ctrl Pts',(-0.452719478359432,1.,-1.92235380648502));
#27031=CARTESIAN_POINT('Ctrl Pts',(-0.455872005174371,-1.,-1.92753067150476));
#27032=CARTESIAN_POINT('Ctrl Pts',(-0.455872005174371,1.,-1.92753067150476));
#27033=CARTESIAN_POINT('Ctrl Pts',(-0.459081234547926,-1.,-1.93269066517934));
#27034=CARTESIAN_POINT('Ctrl Pts',(-0.459081234547926,1.,-1.93269066517934));
#27035=CARTESIAN_POINT('Ctrl Pts',(-0.462340031009056,-1.,-1.93781486640821));
#27036=CARTESIAN_POINT('Ctrl Pts',(-0.462340031009056,1.,-1.93781486640821));
#27037=CARTESIAN_POINT('Ctrl Pts',(-0.46564546202603,-1.,-1.9428979419619));
#27038=CARTESIAN_POINT('Ctrl Pts',(-0.46564546202603,1.,-1.9428979419619));
#27039=CARTESIAN_POINT('Ctrl Pts',(-0.468997482913135,-1.,-1.94794381136514));
#27040=CARTESIAN_POINT('Ctrl Pts',(-0.468997482913135,1.,-1.94794381136514));
#27041=CARTESIAN_POINT('Ctrl Pts',(-0.472397672264072,-1.,-1.95296148278133));
#27042=CARTESIAN_POINT('Ctrl Pts',(-0.472397672264072,1.,-1.95296148278133));
#27043=CARTESIAN_POINT('Ctrl Pts',(-0.475848034683176,-1.,-1.95796111148177));
#27044=CARTESIAN_POINT('Ctrl Pts',(-0.475848034683176,1.,-1.95796111148177));
#27045=CARTESIAN_POINT('Ctrl Pts',(-0.479349583074855,-1.,-1.96294933055943));
#27046=CARTESIAN_POINT('Ctrl Pts',(-0.479349583074855,1.,-1.96294933055943));
#27047=CARTESIAN_POINT('Ctrl Pts',(-0.482901662120691,-1.,-1.96792703422362));
#27048=CARTESIAN_POINT('Ctrl Pts',(-0.482901662120691,1.,-1.96792703422362));
#27049=CARTESIAN_POINT('Ctrl Pts',(-0.486502692907659,-1.,-1.97289186263272));
#27050=CARTESIAN_POINT('Ctrl Pts',(-0.486502692907659,1.,-1.97289186263272));
#27051=CARTESIAN_POINT('Ctrl Pts',(-0.490150627860952,-1.,-1.97783973019229));
#27052=CARTESIAN_POINT('Ctrl Pts',(-0.490150627860952,1.,-1.97783973019229));
#27053=CARTESIAN_POINT('Ctrl Pts',(-0.493843476541495,-1.,-1.98276658761821));
#27054=CARTESIAN_POINT('Ctrl Pts',(-0.493843476541495,1.,-1.98276658761821));
#27055=CARTESIAN_POINT('Ctrl Pts',(-0.497579909545574,-1.,-1.98767044752932));
#27056=CARTESIAN_POINT('Ctrl Pts',(-0.497579909545574,1.,-1.98767044752932));
#27057=CARTESIAN_POINT('Ctrl Pts',(-0.501359287727146,-1.,-1.99255149126155));
#27058=CARTESIAN_POINT('Ctrl Pts',(-0.501359287727146,1.,-1.99255149126155));
#27059=CARTESIAN_POINT('Ctrl Pts',(-0.505181361323026,-1.,-1.99741107463572));
#27060=CARTESIAN_POINT('Ctrl Pts',(-0.505181361323026,1.,-1.99741107463572));
#27061=CARTESIAN_POINT('Ctrl Pts',(-0.509046069886157,-1.,-2.00225107134734));
#27062=CARTESIAN_POINT('Ctrl Pts',(-0.509046069886157,1.,-2.00225107134734));
#27063=CARTESIAN_POINT('Ctrl Pts',(-0.512953306961792,-1.,-2.00707309946949));
#27064=CARTESIAN_POINT('Ctrl Pts',(-0.512953306961792,1.,-2.00707309946949));
#27065=CARTESIAN_POINT('Ctrl Pts',(-0.516902681728687,-1.,-2.01187773939242));
#27066=CARTESIAN_POINT('Ctrl Pts',(-0.516902681728687,1.,-2.01187773939242));
#27067=CARTESIAN_POINT('Ctrl Pts',(-0.52089359039937,-1.,-2.01666477917286));
#27068=CARTESIAN_POINT('Ctrl Pts',(-0.52089359039937,1.,-2.01666477917286));
#27069=CARTESIAN_POINT('Ctrl Pts',(-0.524925318333476,-1.,-2.02143356304698));
#27070=CARTESIAN_POINT('Ctrl Pts',(-0.524925318333476,1.,-2.02143356304698));
#27071=CARTESIAN_POINT('Ctrl Pts',(-0.528997127241914,-1.,-2.0261832908329));
#27072=CARTESIAN_POINT('Ctrl Pts',(-0.528997127241914,1.,-2.0261832908329));
#27073=CARTESIAN_POINT('Ctrl Pts',(-0.533108355132977,-1.,-2.03091336214426));
#27074=CARTESIAN_POINT('Ctrl Pts',(-0.533108355132977,1.,-2.03091336214426));
#27075=CARTESIAN_POINT('Ctrl Pts',(-0.537258489833262,-1.,-2.03562362954037));
#27076=CARTESIAN_POINT('Ctrl Pts',(-0.537258489833262,1.,-2.03562362954037));
#27077=CARTESIAN_POINT('Ctrl Pts',(-0.541447120615659,-1.,-2.04031422690527));
#27078=CARTESIAN_POINT('Ctrl Pts',(-0.541447120615659,1.,-2.04031422690527));
#27079=CARTESIAN_POINT('Ctrl Pts',(-0.54567390381743,-1.,-2.04498544714588));
#27080=CARTESIAN_POINT('Ctrl Pts',(-0.54567390381743,1.,-2.04498544714588));
#27081=CARTESIAN_POINT('Ctrl Pts',(-0.549938525150295,-1.,-2.04963761077958));
#27082=CARTESIAN_POINT('Ctrl Pts',(-0.549938525150295,1.,-2.04963761077958));
#27083=CARTESIAN_POINT('Ctrl Pts',(-0.554240657463906,-1.,-2.05427091604413));
#27084=CARTESIAN_POINT('Ctrl Pts',(-0.554240657463906,1.,-2.05427091604413));
#27085=CARTESIAN_POINT('Ctrl Pts',(-0.558579940185151,-1.,-2.05888537756462));
#27086=CARTESIAN_POINT('Ctrl Pts',(-0.558579940185151,1.,-2.05888537756462));
#27087=CARTESIAN_POINT('Ctrl Pts',(-0.562955993082261,-1.,-2.06348090160589));
#27088=CARTESIAN_POINT('Ctrl Pts',(-0.562955993082261,1.,-2.06348090160589));
#27089=CARTESIAN_POINT('Ctrl Pts',(-0.567368421181087,-1.,-2.06805732997334));
#27090=CARTESIAN_POINT('Ctrl Pts',(-0.567368421181087,1.,-2.06805732997334));
#27091=CARTESIAN_POINT('Ctrl Pts',(-0.571816823242603,-1.,-2.07261449292824));
#27092=CARTESIAN_POINT('Ctrl Pts',(-0.571816823242603,1.,-2.07261449292824));
#27093=CARTESIAN_POINT('Ctrl Pts',(-0.576300797416844,-1.,-2.07715226767559));
#27094=CARTESIAN_POINT('Ctrl Pts',(-0.576300797416844,1.,-2.07715226767559));
#27095=CARTESIAN_POINT('Ctrl Pts',(-0.580819952108063,-1.,-2.08167059018418));
#27096=CARTESIAN_POINT('Ctrl Pts',(-0.580819952108063,1.,-2.08167059018418));
#27097=CARTESIAN_POINT('Ctrl Pts',(-0.585373918991617,-1.,-2.08616943727951));
#27098=CARTESIAN_POINT('Ctrl Pts',(-0.585373918991617,1.,-2.08616943727951));
#27099=CARTESIAN_POINT('Ctrl Pts',(-0.589962365403406,-1.,-2.09064881812129));
#27100=CARTESIAN_POINT('Ctrl Pts',(-0.589962365403406,1.,-2.09064881812129));
#27101=CARTESIAN_POINT('Ctrl Pts',(-0.594585006052162,-1.,-2.0951087622027));
#27102=CARTESIAN_POINT('Ctrl Pts',(-0.594585006052162,1.,-2.0951087622027));
#27103=CARTESIAN_POINT('Ctrl Pts',(-0.599241616420533,-1.,-2.0995493086477));
#27104=CARTESIAN_POINT('Ctrl Pts',(-0.599241616420533,1.,-2.0995493086477));
#27105=CARTESIAN_POINT('Ctrl Pts',(-0.60393203073603,-1.,-2.10397049886949));
#27106=CARTESIAN_POINT('Ctrl Pts',(-0.60393203073603,1.,-2.10397049886949));
#27107=CARTESIAN_POINT('Ctrl Pts',(-0.607711315454876,-1.,-2.1074919961518));
#27108=CARTESIAN_POINT('Ctrl Pts',(-0.607711315454876,1.,-2.1074919961518));
#27109=CARTESIAN_POINT('Ctrl Pts',(-0.610560911689899,-1.,-2.11012443807238));
#27110=CARTESIAN_POINT('Ctrl Pts',(-0.610560911689899,1.,-2.11012443807238));
#27111=CARTESIAN_POINT('Ctrl Pts',(-0.6124673655618,-1.,-2.11187554259986));
#27112=CARTESIAN_POINT('Ctrl Pts',(-0.6124673655618,1.,-2.11187554259986));
#27113=CARTESIAN_POINT('Ctrl Pts',(-0.61342227326009,-1.,-2.11275013067528));
#27114=CARTESIAN_POINT('Ctrl Pts',(-0.61342227326009,1.,-2.11275013067528));
#27115=CARTESIAN_POINT('',(-0.383122945602004,1.,-1.7075470150345));
#27116=CARTESIAN_POINT('Ctrl Pts',(-0.383122945602004,1.,-1.7075470150345));
#27117=CARTESIAN_POINT('Ctrl Pts',(-0.384119047315542,1.,-1.71231062891958));
#27118=CARTESIAN_POINT('Ctrl Pts',(-0.38607079032701,1.,-1.72162022246158));
#27119=CARTESIAN_POINT('Ctrl Pts',(-0.388877023509191,1.,-1.7349317097561));
#27120=CARTESIAN_POINT('Ctrl Pts',(-0.392375812294307,1.,-1.75137405313962));
#27121=CARTESIAN_POINT('Ctrl Pts',(-0.39634619612042,1.,-1.7697556004756));
#27122=CARTESIAN_POINT('Ctrl Pts',(-0.39991940378308,1.,-1.78598826347533));
#27123=CARTESIAN_POINT('Ctrl Pts',(-0.403107976170441,1.,-1.80012077176221));
#27124=CARTESIAN_POINT('Ctrl Pts',(-0.405933518411838,1.,-1.81223801813988));
#27125=CARTESIAN_POINT('Ctrl Pts',(-0.408428948108533,1.,-1.8224702267854));
#27126=CARTESIAN_POINT('Ctrl Pts',(-0.410641256301675,1.,-1.83100408895216));
#27127=CARTESIAN_POINT('Ctrl Pts',(-0.412633125322162,1.,-1.83808953475839));
#27128=CARTESIAN_POINT('Ctrl Pts',(-0.41448743825434,1.,-1.8440575707371));
#27129=CARTESIAN_POINT('Ctrl Pts',(-0.416300022038864,1.,-1.84929312929882));
#27130=CARTESIAN_POINT('Ctrl Pts',(-0.418164129143534,1.,-1.85417632856234));
#27131=CARTESIAN_POINT('Ctrl Pts',(-0.420157287975619,1.,-1.85903281096686));
#27132=CARTESIAN_POINT('Ctrl Pts',(-0.422327307418275,1.,-1.86408083334028));
#27133=CARTESIAN_POINT('Ctrl Pts',(-0.424678177291359,1.,-1.86937803944323));
#27134=CARTESIAN_POINT('Ctrl Pts',(-0.427183828519102,1.,-1.87486989291484));
#27135=CARTESIAN_POINT('Ctrl Pts',(-0.429803062482344,1.,-1.88044229001832));
#27136=CARTESIAN_POINT('Ctrl Pts',(-0.432493038548748,1.,-1.88596913666793));
#27137=CARTESIAN_POINT('Ctrl Pts',(-0.435225660963383,1.,-1.89136993975504));
#27138=CARTESIAN_POINT('Ctrl Pts',(-0.437995003948244,1.,-1.89663648956466));
#27139=CARTESIAN_POINT('Ctrl Pts',(-0.440807833704038,1.,-1.90180124389086));
#27140=CARTESIAN_POINT('Ctrl Pts',(-0.443677556849151,1.,-1.90691756144898));
#27141=CARTESIAN_POINT('Ctrl Pts',(-0.446617343485711,1.,-1.9120369998112));
#27142=CARTESIAN_POINT('Ctrl Pts',(-0.449632260106662,1.,-1.91718342555755));
#27143=CARTESIAN_POINT('Ctrl Pts',(-0.452719478359432,1.,-1.92235380648502));
#27144=CARTESIAN_POINT('Ctrl Pts',(-0.455872005174371,1.,-1.92753067150476));
#27145=CARTESIAN_POINT('Ctrl Pts',(-0.459081234547926,1.,-1.93269066517934));
#27146=CARTESIAN_POINT('Ctrl Pts',(-0.462340031009056,1.,-1.93781486640821));
#27147=CARTESIAN_POINT('Ctrl Pts',(-0.46564546202603,1.,-1.9428979419619));
#27148=CARTESIAN_POINT('Ctrl Pts',(-0.468997482913135,1.,-1.94794381136514));
#27149=CARTESIAN_POINT('Ctrl Pts',(-0.472397672264072,1.,-1.95296148278133));
#27150=CARTESIAN_POINT('Ctrl Pts',(-0.475848034683176,1.,-1.95796111148177));
#27151=CARTESIAN_POINT('Ctrl Pts',(-0.479349583074855,1.,-1.96294933055943));
#27152=CARTESIAN_POINT('Ctrl Pts',(-0.482901662120691,1.,-1.96792703422362));
#27153=CARTESIAN_POINT('Ctrl Pts',(-0.486502692907659,1.,-1.97289186263272));
#27154=CARTESIAN_POINT('Ctrl Pts',(-0.490150627860952,1.,-1.97783973019229));
#27155=CARTESIAN_POINT('Ctrl Pts',(-0.493843476541495,1.,-1.98276658761821));
#27156=CARTESIAN_POINT('Ctrl Pts',(-0.497579909545574,1.,-1.98767044752932));
#27157=CARTESIAN_POINT('Ctrl Pts',(-0.501359287727146,1.,-1.99255149126155));
#27158=CARTESIAN_POINT('Ctrl Pts',(-0.505181361323026,1.,-1.99741107463572));
#27159=CARTESIAN_POINT('Ctrl Pts',(-0.509046069886157,1.,-2.00225107134734));
#27160=CARTESIAN_POINT('Ctrl Pts',(-0.512953306961792,1.,-2.00707309946949));
#27161=CARTESIAN_POINT('Ctrl Pts',(-0.516902681728687,1.,-2.01187773939242));
#27162=CARTESIAN_POINT('Ctrl Pts',(-0.52089359039937,1.,-2.01666477917286));
#27163=CARTESIAN_POINT('Ctrl Pts',(-0.524925318333476,1.,-2.02143356304698));
#27164=CARTESIAN_POINT('Ctrl Pts',(-0.528997127241914,1.,-2.0261832908329));
#27165=CARTESIAN_POINT('Ctrl Pts',(-0.533108355132977,1.,-2.03091336214426));
#27166=CARTESIAN_POINT('Ctrl Pts',(-0.537258489833262,1.,-2.03562362954037));
#27167=CARTESIAN_POINT('Ctrl Pts',(-0.541447120615659,1.,-2.04031422690527));
#27168=CARTESIAN_POINT('Ctrl Pts',(-0.54567390381743,1.,-2.04498544714588));
#27169=CARTESIAN_POINT('Ctrl Pts',(-0.549938525150295,1.,-2.04963761077958));
#27170=CARTESIAN_POINT('Ctrl Pts',(-0.554240657463906,1.,-2.05427091604413));
#27171=CARTESIAN_POINT('Ctrl Pts',(-0.558579940185151,1.,-2.05888537756462));
#27172=CARTESIAN_POINT('Ctrl Pts',(-0.562955993082261,1.,-2.06348090160589));
#27173=CARTESIAN_POINT('Ctrl Pts',(-0.567368421181087,1.,-2.06805732997334));
#27174=CARTESIAN_POINT('Ctrl Pts',(-0.571816823242603,1.,-2.07261449292824));
#27175=CARTESIAN_POINT('Ctrl Pts',(-0.576300797416844,1.,-2.07715226767559));
#27176=CARTESIAN_POINT('Ctrl Pts',(-0.580819952108063,1.,-2.08167059018418));
#27177=CARTESIAN_POINT('Ctrl Pts',(-0.585373918991617,1.,-2.08616943727951));
#27178=CARTESIAN_POINT('Ctrl Pts',(-0.589962365403406,1.,-2.09064881812129));
#27179=CARTESIAN_POINT('Ctrl Pts',(-0.594585006052162,1.,-2.0951087622027));
#27180=CARTESIAN_POINT('Ctrl Pts',(-0.599241616420533,1.,-2.0995493086477));
#27181=CARTESIAN_POINT('Ctrl Pts',(-0.60393203073603,1.,-2.10397049886949));
#27182=CARTESIAN_POINT('Ctrl Pts',(-0.607711315454876,1.,-2.1074919961518));
#27183=CARTESIAN_POINT('Ctrl Pts',(-0.610560911689899,1.,-2.11012443807238));
#27184=CARTESIAN_POINT('Ctrl Pts',(-0.6124673655618,1.,-2.11187554259986));
#27185=CARTESIAN_POINT('Ctrl Pts',(-0.61342227326009,1.,-2.11275013067528));
#27186=CARTESIAN_POINT('',(-0.383122945602003,0.,-1.7075470150345));
#27187=CARTESIAN_POINT('Origin',(0.,0.,0.));
#27188=CARTESIAN_POINT('',(-0.163289472382896,1.,-1.74236521665491));
#27189=CARTESIAN_POINT('Origin',(0.,1.,0.));
#27190=CARTESIAN_POINT('',(-0.163289472382896,0.,-1.74236521665491));
#27191=CARTESIAN_POINT('Ctrl Pts',(-0.0694764450219581,-1.,-2.19890268624765));
#27192=CARTESIAN_POINT('Ctrl Pts',(-0.0694764450219581,1.,-2.19890268624765));
#27193=CARTESIAN_POINT('Ctrl Pts',(-0.070114353632549,-1.,-2.19777582085423));
#27194=CARTESIAN_POINT('Ctrl Pts',(-0.070114353632549,1.,-2.19777582085423));
#27195=CARTESIAN_POINT('Ctrl Pts',(-0.0713863779526154,-1.,-2.19552129484002));
#27196=CARTESIAN_POINT('Ctrl Pts',(-0.0713863779526154,1.,-2.19552129484002));
#27197=CARTESIAN_POINT('Ctrl Pts',(-0.0732830357306725,-1.,-2.19213712013662));
#27198=CARTESIAN_POINT('Ctrl Pts',(-0.0732830357306725,1.,-2.19213712013662));
#27199=CARTESIAN_POINT('Ctrl Pts',(-0.0757891465836148,-1.,-2.1876201139953));
#27200=CARTESIAN_POINT('Ctrl Pts',(-0.0757891465836148,1.,-2.1876201139953));
#27201=CARTESIAN_POINT('Ctrl Pts',(-0.0788837727685243,-1.,-2.18196589448887));
#27202=CARTESIAN_POINT('Ctrl Pts',(-0.0788837727685243,1.,-2.18196589448887));
#27203=CARTESIAN_POINT('Ctrl Pts',(-0.0819402680872765,-1.,-2.176303712113));
#27204=CARTESIAN_POINT('Ctrl Pts',(-0.0819402680872765,1.,-2.176303712113));
#27205=CARTESIAN_POINT('Ctrl Pts',(-0.0849584620835372,-1.,-2.17063357870952));
#27206=CARTESIAN_POINT('Ctrl Pts',(-0.0849584620835372,1.,-2.17063357870952));
#27207=CARTESIAN_POINT('Ctrl Pts',(-0.0879381291386923,-1.,-2.16495552645014));
#27208=CARTESIAN_POINT('Ctrl Pts',(-0.0879381291386923,1.,-2.16495552645014));
#27209=CARTESIAN_POINT('Ctrl Pts',(-0.0908789888107265,-1.,-2.15926961544516));
#27210=CARTESIAN_POINT('Ctrl Pts',(-0.0908789888107265,1.,-2.15926961544516));
#27211=CARTESIAN_POINT('Ctrl Pts',(-0.0937807218867643,-1.,-2.1535759397817));
#27212=CARTESIAN_POINT('Ctrl Pts',(-0.0937807218867643,1.,-2.1535759397817));
#27213=CARTESIAN_POINT('Ctrl Pts',(-0.0966429852305459,-1.,-2.14787463531795));
#27214=CARTESIAN_POINT('Ctrl Pts',(-0.0966429852305459,1.,-2.14787463531795));
#27215=CARTESIAN_POINT('Ctrl Pts',(-0.0994654261990915,-1.,-2.14216588396025));
#27216=CARTESIAN_POINT('Ctrl Pts',(-0.0994654261990915,1.,-2.14216588396025));
#27217=CARTESIAN_POINT('Ctrl Pts',(-0.1022477005561,-1.,-2.13644992667165));
#27218=CARTESIAN_POINT('Ctrl Pts',(-0.1022477005561,1.,-2.13644992667165));
#27219=CARTESIAN_POINT('Ctrl Pts',(-0.104989479152739,-1.,-2.13072704887293));
#27220=CARTESIAN_POINT('Ctrl Pts',(-0.104989479152739,1.,-2.13072704887293));
#27221=CARTESIAN_POINT('Ctrl Pts',(-0.10769043523109,-1.,-2.12499752307));
#27222=CARTESIAN_POINT('Ctrl Pts',(-0.10769043523109,1.,-2.12499752307));
#27223=CARTESIAN_POINT('Ctrl Pts',(-0.110350236135025,-1.,-2.11926155590865));
#27224=CARTESIAN_POINT('Ctrl Pts',(-0.110350236135025,1.,-2.11926155590865));
#27225=CARTESIAN_POINT('Ctrl Pts',(-0.112968534419737,-1.,-2.11351924490306));
#27226=CARTESIAN_POINT('Ctrl Pts',(-0.112968534419737,1.,-2.11351924490306));
#27227=CARTESIAN_POINT('Ctrl Pts',(-0.115544957687926,-1.,-2.10777050261309));
#27228=CARTESIAN_POINT('Ctrl Pts',(-0.115544957687926,1.,-2.10777050261309));
#27229=CARTESIAN_POINT('Ctrl Pts',(-0.118079107988355,-1.,-2.102015121329));
#27230=CARTESIAN_POINT('Ctrl Pts',(-0.118079107988355,1.,-2.102015121329));
#27231=CARTESIAN_POINT('Ctrl Pts',(-0.120570567965122,-1.,-2.0962529286773));
#27232=CARTESIAN_POINT('Ctrl Pts',(-0.120570567965122,1.,-2.0962529286773));
#27233=CARTESIAN_POINT('Ctrl Pts',(-0.123018905621083,-1.,-2.09048392424825));
#27234=CARTESIAN_POINT('Ctrl Pts',(-0.123018905621083,1.,-2.09048392424825));
#27235=CARTESIAN_POINT('Ctrl Pts',(-0.125423679412061,-1.,-2.08470840653643));
#27236=CARTESIAN_POINT('Ctrl Pts',(-0.125423679412061,1.,-2.08470840653643));
#27237=CARTESIAN_POINT('Ctrl Pts',(-0.12778444527612,-1.,-2.07892715110987));
#27238=CARTESIAN_POINT('Ctrl Pts',(-0.12778444527612,1.,-2.07892715110987));
#27239=CARTESIAN_POINT('Ctrl Pts',(-0.130100748328403,-1.,-2.07314114713063));
#27240=CARTESIAN_POINT('Ctrl Pts',(-0.130100748328403,1.,-2.07314114713063));
#27241=CARTESIAN_POINT('Ctrl Pts',(-0.13237211154771,-1.,-2.06735123910326));
#27242=CARTESIAN_POINT('Ctrl Pts',(-0.13237211154771,1.,-2.06735123910326));
#27243=CARTESIAN_POINT('Ctrl Pts',(-0.134598026192106,-1.,-2.06155781517842));
#27244=CARTESIAN_POINT('Ctrl Pts',(-0.134598026192106,1.,-2.06155781517842));
#27245=CARTESIAN_POINT('Ctrl Pts',(-0.136777941218044,-1.,-2.05576044414264));
#27246=CARTESIAN_POINT('Ctrl Pts',(-0.136777941218044,1.,-2.05576044414264));
#27247=CARTESIAN_POINT('Ctrl Pts',(-0.138911255368966,-1.,-2.04995762001328));
#27248=CARTESIAN_POINT('Ctrl Pts',(-0.138911255368966,1.,-2.04995762001328));
#27249=CARTESIAN_POINT('Ctrl Pts',(-0.140997332152546,-1.,-2.04414757947916));
#27250=CARTESIAN_POINT('Ctrl Pts',(-0.140997332152546,1.,-2.04414757947916));
#27251=CARTESIAN_POINT('Ctrl Pts',(-0.143035515058209,-1.,-2.03832911025912));
#27252=CARTESIAN_POINT('Ctrl Pts',(-0.143035515058209,1.,-2.03832911025912));
#27253=CARTESIAN_POINT('Ctrl Pts',(-0.145025140186057,-1.,-2.03250223739942));
#27254=CARTESIAN_POINT('Ctrl Pts',(-0.145025140186057,1.,-2.03250223739942));
#27255=CARTESIAN_POINT('Ctrl Pts',(-0.146965557332583,-1.,-2.02666926182017));
#27256=CARTESIAN_POINT('Ctrl Pts',(-0.146965557332583,1.,-2.02666926182017));
#27257=CARTESIAN_POINT('Ctrl Pts',(-0.148856124775337,-1.,-2.02083464969894));
#27258=CARTESIAN_POINT('Ctrl Pts',(-0.148856124775337,1.,-2.02083464969894));
#27259=CARTESIAN_POINT('Ctrl Pts',(-0.150696157673078,-1.,-2.01500291940238));
#27260=CARTESIAN_POINT('Ctrl Pts',(-0.150696157673078,1.,-2.01500291940238));
#27261=CARTESIAN_POINT('Ctrl Pts',(-0.15248488362145,-1.,-2.00917680318424));
#27262=CARTESIAN_POINT('Ctrl Pts',(-0.15248488362145,1.,-2.00917680318424));
#27263=CARTESIAN_POINT('Ctrl Pts',(-0.154221403049722,-1.,-2.00335565310543));
#27264=CARTESIAN_POINT('Ctrl Pts',(-0.154221403049722,1.,-2.00335565310543));
#27265=CARTESIAN_POINT('Ctrl Pts',(-0.155904629548783,-1.,-1.99753284771497));
#27266=CARTESIAN_POINT('Ctrl Pts',(-0.155904629548783,1.,-1.99753284771497));
#27267=CARTESIAN_POINT('Ctrl Pts',(-0.157533331459227,-1.,-1.99169810931908));
#27268=CARTESIAN_POINT('Ctrl Pts',(-0.157533331459227,1.,-1.99169810931908));
#27269=CARTESIAN_POINT('Ctrl Pts',(-0.159106226437299,-1.,-1.98584238283292));
#27270=CARTESIAN_POINT('Ctrl Pts',(-0.159106226437299,1.,-1.98584238283292));
#27271=CARTESIAN_POINT('Ctrl Pts',(-0.160622060784611,-1.,-1.97996195437559));
#27272=CARTESIAN_POINT('Ctrl Pts',(-0.160622060784611,1.,-1.97996195437559));
#27273=CARTESIAN_POINT('Ctrl Pts',(-0.162079693556289,-1.,-1.97406280235188));
#27274=CARTESIAN_POINT('Ctrl Pts',(-0.162079693556289,1.,-1.97406280235188));
#27275=CARTESIAN_POINT('Ctrl Pts',(-0.163478185457734,-1.,-1.96816512677967));
#27276=CARTESIAN_POINT('Ctrl Pts',(-0.163478185457734,1.,-1.96816512677967));
#27277=CARTESIAN_POINT('Ctrl Pts',(-0.164816568920269,-1.,-1.96229379940136));
#27278=CARTESIAN_POINT('Ctrl Pts',(-0.164816568920269,1.,-1.96229379940136));
#27279=CARTESIAN_POINT('Ctrl Pts',(-0.166093592002812,-1.,-1.9564675971873));
#27280=CARTESIAN_POINT('Ctrl Pts',(-0.166093592002812,1.,-1.9564675971873));
#27281=CARTESIAN_POINT('Ctrl Pts',(-0.167307501784475,-1.,-1.95069027794294));
#27282=CARTESIAN_POINT('Ctrl Pts',(-0.167307501784475,1.,-1.95069027794294));
#27283=CARTESIAN_POINT('Ctrl Pts',(-0.168455741607556,-1.,-1.94493757756931));
#27284=CARTESIAN_POINT('Ctrl Pts',(-0.168455741607556,1.,-1.94493757756931));
#27285=CARTESIAN_POINT('Ctrl Pts',(-0.169534904817491,-1.,-1.93915639211581));
#27286=CARTESIAN_POINT('Ctrl Pts',(-0.169534904817491,1.,-1.93915639211581));
#27287=CARTESIAN_POINT('Ctrl Pts',(-0.170541253116202,-1.,-1.93329183155539));
#27288=CARTESIAN_POINT('Ctrl Pts',(-0.170541253116202,1.,-1.93329183155539));
#27289=CARTESIAN_POINT('Ctrl Pts',(-0.171471191532988,-1.,-1.92731093582036));
#27290=CARTESIAN_POINT('Ctrl Pts',(-0.171471191532988,1.,-1.92731093582036));
#27291=CARTESIAN_POINT('Ctrl Pts',(-0.172321621259514,-1.,-1.9212233439798));
#27292=CARTESIAN_POINT('Ctrl Pts',(-0.172321621259514,1.,-1.9212233439798));
#27293=CARTESIAN_POINT('Ctrl Pts',(-0.173090695383496,-1.,-1.91511429159527));
#27294=CARTESIAN_POINT('Ctrl Pts',(-0.173090695383496,1.,-1.91511429159527));
#27295=CARTESIAN_POINT('Ctrl Pts',(-0.173776635257817,-1.,-1.90911693975267));
#27296=CARTESIAN_POINT('Ctrl Pts',(-0.173776635257817,1.,-1.90911693975267));
#27297=CARTESIAN_POINT('Ctrl Pts',(-0.174375518661085,-1.,-1.90335253862834));
#27298=CARTESIAN_POINT('Ctrl Pts',(-0.174375518661085,1.,-1.90335253862834));
#27299=CARTESIAN_POINT('Ctrl Pts',(-0.174879405091263,-1.,-1.89788101117132));
#27300=CARTESIAN_POINT('Ctrl Pts',(-0.174879405091263,1.,-1.89788101117132));
#27301=CARTESIAN_POINT('Ctrl Pts',(-0.175274276190844,-1.,-1.892646301985));
#27302=CARTESIAN_POINT('Ctrl Pts',(-0.175274276190844,1.,-1.892646301985));
#27303=CARTESIAN_POINT('Ctrl Pts',(-0.175538155840648,-1.,-1.88742606273259));
#27304=CARTESIAN_POINT('Ctrl Pts',(-0.175538155840648,1.,-1.88742606273259));
#27305=CARTESIAN_POINT('Ctrl Pts',(-0.175644148889699,-1.,-1.88188663145367));
#27306=CARTESIAN_POINT('Ctrl Pts',(-0.175644148889699,1.,-1.88188663145367));
#27307=CARTESIAN_POINT('Ctrl Pts',(-0.175563480746485,-1.,-1.87563767773588));
#27308=CARTESIAN_POINT('Ctrl Pts',(-0.175563480746485,1.,-1.87563767773588));
#27309=CARTESIAN_POINT('Ctrl Pts',(-0.175268337590758,-1.,-1.86828349694799));
#27310=CARTESIAN_POINT('Ctrl Pts',(-0.175268337590758,1.,-1.86828349694799));
#27311=CARTESIAN_POINT('Ctrl Pts',(-0.17473525927603,-1.,-1.85948367088837));
#27312=CARTESIAN_POINT('Ctrl Pts',(-0.17473525927603,1.,-1.85948367088837));
#27313=CARTESIAN_POINT('Ctrl Pts',(-0.173946627587731,-1.,-1.8489811319852));
#27314=CARTESIAN_POINT('Ctrl Pts',(-0.173946627587731,1.,-1.8489811319852));
#27315=CARTESIAN_POINT('Ctrl Pts',(-0.1728894428919,-1.,-1.83658380527692));
#27316=CARTESIAN_POINT('Ctrl Pts',(-0.1728894428919,1.,-1.83658380527692));
#27317=CARTESIAN_POINT('Ctrl Pts',(-0.171554770204119,-1.,-1.82215766811545));
#27318=CARTESIAN_POINT('Ctrl Pts',(-0.171554770204119,1.,-1.82215766811545));
#27319=CARTESIAN_POINT('Ctrl Pts',(-0.169936923904608,-1.,-1.80561530629706));
#27320=CARTESIAN_POINT('Ctrl Pts',(-0.169936923904608,1.,-1.80561530629706));
#27321=CARTESIAN_POINT('Ctrl Pts',(-0.168032772805197,-1.,-1.7869064998507));
#27322=CARTESIAN_POINT('Ctrl Pts',(-0.168032772805197,1.,-1.7869064998507));
#27323=CARTESIAN_POINT('Ctrl Pts',(-0.1662793551464,-1.,-1.77018771684844));
#27324=CARTESIAN_POINT('Ctrl Pts',(-0.1662793551464,1.,-1.77018771684844));
#27325=CARTESIAN_POINT('Ctrl Pts',(-0.164834765707158,-1.,-1.75666056638427));
#27326=CARTESIAN_POINT('Ctrl Pts',(-0.164834765707158,1.,-1.75666056638427));
#27327=CARTESIAN_POINT('Ctrl Pts',(-0.163814161002002,-1.,-1.7472034950333));
#27328=CARTESIAN_POINT('Ctrl Pts',(-0.163814161002002,1.,-1.7472034950333));
#27329=CARTESIAN_POINT('Ctrl Pts',(-0.163289472382896,-1.,-1.74236521665491));
#27330=CARTESIAN_POINT('Ctrl Pts',(-0.163289472382896,1.,-1.74236521665491));
#27331=CARTESIAN_POINT('',(-0.0694764450219581,1.,-2.19890268624765));
#27332=CARTESIAN_POINT('Ctrl Pts',(-0.0694764450219581,1.,-2.19890268624765));
#27333=CARTESIAN_POINT('Ctrl Pts',(-0.070114353632549,1.,-2.19777582085423));
#27334=CARTESIAN_POINT('Ctrl Pts',(-0.0713863779526154,1.,-2.19552129484002));
#27335=CARTESIAN_POINT('Ctrl Pts',(-0.0732830357306725,1.,-2.19213712013662));
#27336=CARTESIAN_POINT('Ctrl Pts',(-0.0757891465836148,1.,-2.1876201139953));
#27337=CARTESIAN_POINT('Ctrl Pts',(-0.0788837727685243,1.,-2.18196589448887));
#27338=CARTESIAN_POINT('Ctrl Pts',(-0.0819402680872765,1.,-2.176303712113));
#27339=CARTESIAN_POINT('Ctrl Pts',(-0.0849584620835372,1.,-2.17063357870952));
#27340=CARTESIAN_POINT('Ctrl Pts',(-0.0879381291386923,1.,-2.16495552645014));
#27341=CARTESIAN_POINT('Ctrl Pts',(-0.0908789888107265,1.,-2.15926961544516));
#27342=CARTESIAN_POINT('Ctrl Pts',(-0.0937807218867643,1.,-2.1535759397817));
#27343=CARTESIAN_POINT('Ctrl Pts',(-0.0966429852305459,1.,-2.14787463531795));
#27344=CARTESIAN_POINT('Ctrl Pts',(-0.0994654261990915,1.,-2.14216588396025));
#27345=CARTESIAN_POINT('Ctrl Pts',(-0.1022477005561,1.,-2.13644992667165));
#27346=CARTESIAN_POINT('Ctrl Pts',(-0.104989479152739,1.,-2.13072704887293));
#27347=CARTESIAN_POINT('Ctrl Pts',(-0.10769043523109,1.,-2.12499752307));
#27348=CARTESIAN_POINT('Ctrl Pts',(-0.110350236135025,1.,-2.11926155590865));
#27349=CARTESIAN_POINT('Ctrl Pts',(-0.112968534419737,1.,-2.11351924490306));
#27350=CARTESIAN_POINT('Ctrl Pts',(-0.115544957687926,1.,-2.10777050261309));
#27351=CARTESIAN_POINT('Ctrl Pts',(-0.118079107988355,1.,-2.102015121329));
#27352=CARTESIAN_POINT('Ctrl Pts',(-0.120570567965122,1.,-2.0962529286773));
#27353=CARTESIAN_POINT('Ctrl Pts',(-0.123018905621083,1.,-2.09048392424825));
#27354=CARTESIAN_POINT('Ctrl Pts',(-0.125423679412061,1.,-2.08470840653643));
#27355=CARTESIAN_POINT('Ctrl Pts',(-0.12778444527612,1.,-2.07892715110987));
#27356=CARTESIAN_POINT('Ctrl Pts',(-0.130100748328403,1.,-2.07314114713063));
#27357=CARTESIAN_POINT('Ctrl Pts',(-0.13237211154771,1.,-2.06735123910326));
#27358=CARTESIAN_POINT('Ctrl Pts',(-0.134598026192106,1.,-2.06155781517842));
#27359=CARTESIAN_POINT('Ctrl Pts',(-0.136777941218044,1.,-2.05576044414264));
#27360=CARTESIAN_POINT('Ctrl Pts',(-0.138911255368966,1.,-2.04995762001328));
#27361=CARTESIAN_POINT('Ctrl Pts',(-0.140997332152546,1.,-2.04414757947916));
#27362=CARTESIAN_POINT('Ctrl Pts',(-0.143035515058209,1.,-2.03832911025912));
#27363=CARTESIAN_POINT('Ctrl Pts',(-0.145025140186057,1.,-2.03250223739942));
#27364=CARTESIAN_POINT('Ctrl Pts',(-0.146965557332583,1.,-2.02666926182017));
#27365=CARTESIAN_POINT('Ctrl Pts',(-0.148856124775337,1.,-2.02083464969894));
#27366=CARTESIAN_POINT('Ctrl Pts',(-0.150696157673078,1.,-2.01500291940238));
#27367=CARTESIAN_POINT('Ctrl Pts',(-0.15248488362145,1.,-2.00917680318424));
#27368=CARTESIAN_POINT('Ctrl Pts',(-0.154221403049722,1.,-2.00335565310543));
#27369=CARTESIAN_POINT('Ctrl Pts',(-0.155904629548783,1.,-1.99753284771497));
#27370=CARTESIAN_POINT('Ctrl Pts',(-0.157533331459227,1.,-1.99169810931908));
#27371=CARTESIAN_POINT('Ctrl Pts',(-0.159106226437299,1.,-1.98584238283292));
#27372=CARTESIAN_POINT('Ctrl Pts',(-0.160622060784611,1.,-1.97996195437559));
#27373=CARTESIAN_POINT('Ctrl Pts',(-0.162079693556289,1.,-1.97406280235188));
#27374=CARTESIAN_POINT('Ctrl Pts',(-0.163478185457734,1.,-1.96816512677967));
#27375=CARTESIAN_POINT('Ctrl Pts',(-0.164816568920269,1.,-1.96229379940136));
#27376=CARTESIAN_POINT('Ctrl Pts',(-0.166093592002812,1.,-1.9564675971873));
#27377=CARTESIAN_POINT('Ctrl Pts',(-0.167307501784475,1.,-1.95069027794294));
#27378=CARTESIAN_POINT('Ctrl Pts',(-0.168455741607556,1.,-1.94493757756931));
#27379=CARTESIAN_POINT('Ctrl Pts',(-0.169534904817491,1.,-1.93915639211581));
#27380=CARTESIAN_POINT('Ctrl Pts',(-0.170541253116202,1.,-1.93329183155539));
#27381=CARTESIAN_POINT('Ctrl Pts',(-0.171471191532988,1.,-1.92731093582036));
#27382=CARTESIAN_POINT('Ctrl Pts',(-0.172321621259514,1.,-1.9212233439798));
#27383=CARTESIAN_POINT('Ctrl Pts',(-0.173090695383496,1.,-1.91511429159527));
#27384=CARTESIAN_POINT('Ctrl Pts',(-0.173776635257817,1.,-1.90911693975267));
#27385=CARTESIAN_POINT('Ctrl Pts',(-0.174375518661085,1.,-1.90335253862834));
#27386=CARTESIAN_POINT('Ctrl Pts',(-0.174879405091263,1.,-1.89788101117132));
#27387=CARTESIAN_POINT('Ctrl Pts',(-0.175274276190844,1.,-1.892646301985));
#27388=CARTESIAN_POINT('Ctrl Pts',(-0.175538155840648,1.,-1.88742606273259));
#27389=CARTESIAN_POINT('Ctrl Pts',(-0.175644148889699,1.,-1.88188663145367));
#27390=CARTESIAN_POINT('Ctrl Pts',(-0.175563480746485,1.,-1.87563767773588));
#27391=CARTESIAN_POINT('Ctrl Pts',(-0.175268337590758,1.,-1.86828349694799));
#27392=CARTESIAN_POINT('Ctrl Pts',(-0.17473525927603,1.,-1.85948367088837));
#27393=CARTESIAN_POINT('Ctrl Pts',(-0.173946627587731,1.,-1.8489811319852));
#27394=CARTESIAN_POINT('Ctrl Pts',(-0.1728894428919,1.,-1.83658380527692));
#27395=CARTESIAN_POINT('Ctrl Pts',(-0.171554770204119,1.,-1.82215766811545));
#27396=CARTESIAN_POINT('Ctrl Pts',(-0.169936923904608,1.,-1.80561530629706));
#27397=CARTESIAN_POINT('Ctrl Pts',(-0.168032772805197,1.,-1.7869064998507));
#27398=CARTESIAN_POINT('Ctrl Pts',(-0.1662793551464,1.,-1.77018771684844));
#27399=CARTESIAN_POINT('Ctrl Pts',(-0.164834765707158,1.,-1.75666056638427));
#27400=CARTESIAN_POINT('Ctrl Pts',(-0.163814161002002,1.,-1.7472034950333));
#27401=CARTESIAN_POINT('Ctrl Pts',(-0.163289472382896,1.,-1.74236521665491));
#27402=CARTESIAN_POINT('',(-0.0694764450219581,0.,-2.19890268624765));
#27403=CARTESIAN_POINT('Origin',(0.0694764450219584,0.,-2.19890268624765));
#27404=CARTESIAN_POINT('',(0.0694764450219584,1.,-2.19890268624765));
#27405=CARTESIAN_POINT('',(-0.0694764450219581,1.,-2.19890268624765));
#27406=CARTESIAN_POINT('',(0.0694764450219584,0.,-2.19890268624765));
#27407=CARTESIAN_POINT('Ctrl Pts',(0.163289472382896,-1.,-1.74236521665491));
#27408=CARTESIAN_POINT('Ctrl Pts',(0.163289472382896,1.,-1.74236521665491));
#27409=CARTESIAN_POINT('Ctrl Pts',(0.163814161002474,-1.,-1.74720349503904));
#27410=CARTESIAN_POINT('Ctrl Pts',(0.163814161002474,1.,-1.74720349503904));
#27411=CARTESIAN_POINT('Ctrl Pts',(0.164834765708484,-1.,-1.75666056640041));
#27412=CARTESIAN_POINT('Ctrl Pts',(0.164834765708484,1.,-1.75666056640041));
#27413=CARTESIAN_POINT('Ctrl Pts',(0.166279355148738,-1.,-1.77018771687692));
#27414=CARTESIAN_POINT('Ctrl Pts',(0.166279355148738,1.,-1.77018771687692));
#27415=CARTESIAN_POINT('Ctrl Pts',(0.16803277280837,-1.,-1.78690649988931));
#27416=CARTESIAN_POINT('Ctrl Pts',(0.16803277280837,1.,-1.78690649988931));
#27417=CARTESIAN_POINT('Ctrl Pts',(0.169936923908078,-1.,-1.80561530633924));
#27418=CARTESIAN_POINT('Ctrl Pts',(0.169936923908078,1.,-1.80561530633924));
#27419=CARTESIAN_POINT('Ctrl Pts',(0.171554770207306,-1.,-1.82215766815414));
#27420=CARTESIAN_POINT('Ctrl Pts',(0.171554770207306,1.,-1.82215766815414));
#27421=CARTESIAN_POINT('Ctrl Pts',(0.17288944289442,-1.,-1.83658380530747));
#27422=CARTESIAN_POINT('Ctrl Pts',(0.17288944289442,1.,-1.83658380530747));
#27423=CARTESIAN_POINT('Ctrl Pts',(0.173946627589401,-1.,-1.84898113200543));
#27424=CARTESIAN_POINT('Ctrl Pts',(0.173946627589401,1.,-1.84898113200543));
#27425=CARTESIAN_POINT('Ctrl Pts',(0.174735259276856,-1.,-1.85948367089838));
#27426=CARTESIAN_POINT('Ctrl Pts',(0.174735259276856,1.,-1.85948367089838));
#27427=CARTESIAN_POINT('Ctrl Pts',(0.175268337590901,-1.,-1.86828349694972));
#27428=CARTESIAN_POINT('Ctrl Pts',(0.175268337590901,1.,-1.86828349694972));
#27429=CARTESIAN_POINT('Ctrl Pts',(0.175563480746205,-1.,-1.87563767773249));
#27430=CARTESIAN_POINT('Ctrl Pts',(0.175563480746205,1.,-1.87563767773249));
#27431=CARTESIAN_POINT('Ctrl Pts',(0.175644148889271,-1.,-1.88188663144846));
#27432=CARTESIAN_POINT('Ctrl Pts',(0.175644148889271,1.,-1.88188663144846));
#27433=CARTESIAN_POINT('Ctrl Pts',(0.175538155840286,-1.,-1.88742606272818));
#27434=CARTESIAN_POINT('Ctrl Pts',(0.175538155840286,1.,-1.88742606272818));
#27435=CARTESIAN_POINT('Ctrl Pts',(0.175274276190664,-1.,-1.89264630198279));
#27436=CARTESIAN_POINT('Ctrl Pts',(0.175274276190664,1.,-1.89264630198279));
#27437=CARTESIAN_POINT('Ctrl Pts',(0.174879405091277,-1.,-1.89788101117148));
#27438=CARTESIAN_POINT('Ctrl Pts',(0.174879405091277,1.,-1.89788101117148));
#27439=CARTESIAN_POINT('Ctrl Pts',(0.174375518661222,-1.,-1.90335253863003));
#27440=CARTESIAN_POINT('Ctrl Pts',(0.174375518661222,1.,-1.90335253863003));
#27441=CARTESIAN_POINT('Ctrl Pts',(0.173776635257984,-1.,-1.90911693975475));
#27442=CARTESIAN_POINT('Ctrl Pts',(0.173776635257984,1.,-1.90911693975475));
#27443=CARTESIAN_POINT('Ctrl Pts',(0.173090695383619,-1.,-1.91511429159681));
#27444=CARTESIAN_POINT('Ctrl Pts',(0.173090695383619,1.,-1.91511429159681));
#27445=CARTESIAN_POINT('Ctrl Pts',(0.172321621259557,-1.,-1.92122334398034));
#27446=CARTESIAN_POINT('Ctrl Pts',(0.172321621259557,1.,-1.92122334398034));
#27447=CARTESIAN_POINT('Ctrl Pts',(0.17147119153296,-1.,-1.92731093582));
#27448=CARTESIAN_POINT('Ctrl Pts',(0.17147119153296,1.,-1.92731093582));
#27449=CARTESIAN_POINT('Ctrl Pts',(0.170541253116136,-1.,-1.93329183155455));
#27450=CARTESIAN_POINT('Ctrl Pts',(0.170541253116136,1.,-1.93329183155455));
#27451=CARTESIAN_POINT('Ctrl Pts',(0.169534904817425,-1.,-1.93915639211497));
#27452=CARTESIAN_POINT('Ctrl Pts',(0.169534904817425,1.,-1.93915639211497));
#27453=CARTESIAN_POINT('Ctrl Pts',(0.168455741607516,-1.,-1.94493757756879));
#27454=CARTESIAN_POINT('Ctrl Pts',(0.168455741607516,1.,-1.94493757756879));
#27455=CARTESIAN_POINT('Ctrl Pts',(0.167307501784469,-1.,-1.95069027794286));
#27456=CARTESIAN_POINT('Ctrl Pts',(0.167307501784469,1.,-1.95069027794286));
#27457=CARTESIAN_POINT('Ctrl Pts',(0.166093592002833,-1.,-1.95646759718755));
#27458=CARTESIAN_POINT('Ctrl Pts',(0.166093592002833,1.,-1.95646759718755));
#27459=CARTESIAN_POINT('Ctrl Pts',(0.1648165689203,-1.,-1.96229379940174));
#27460=CARTESIAN_POINT('Ctrl Pts',(0.1648165689203,1.,-1.96229379940174));
#27461=CARTESIAN_POINT('Ctrl Pts',(0.16347818545776,-1.,-1.96816512678));
#27462=CARTESIAN_POINT('Ctrl Pts',(0.16347818545776,1.,-1.96816512678));
#27463=CARTESIAN_POINT('Ctrl Pts',(0.162079693556302,-1.,-1.97406280235204));
#27464=CARTESIAN_POINT('Ctrl Pts',(0.162079693556302,1.,-1.97406280235204));
#27465=CARTESIAN_POINT('Ctrl Pts',(0.16062206078461,-1.,-1.97996195437557));
#27466=CARTESIAN_POINT('Ctrl Pts',(0.16062206078461,1.,-1.97996195437557));
#27467=CARTESIAN_POINT('Ctrl Pts',(0.159106226437288,-1.,-1.98584238283279));
#27468=CARTESIAN_POINT('Ctrl Pts',(0.159106226437288,1.,-1.98584238283279));
#27469=CARTESIAN_POINT('Ctrl Pts',(0.157533331459215,-1.,-1.99169810931893));
#27470=CARTESIAN_POINT('Ctrl Pts',(0.157533331459215,1.,-1.99169810931893));
#27471=CARTESIAN_POINT('Ctrl Pts',(0.155904629548774,-1.,-1.99753284771487));
#27472=CARTESIAN_POINT('Ctrl Pts',(0.155904629548774,1.,-1.99753284771487));
#27473=CARTESIAN_POINT('Ctrl Pts',(0.154221403049719,-1.,-2.00335565310539));
#27474=CARTESIAN_POINT('Ctrl Pts',(0.154221403049719,1.,-2.00335565310539));
#27475=CARTESIAN_POINT('Ctrl Pts',(0.152484883621452,-1.,-2.00917680318426));
#27476=CARTESIAN_POINT('Ctrl Pts',(0.152484883621452,1.,-2.00917680318426));
#27477=CARTESIAN_POINT('Ctrl Pts',(0.150696157673084,-1.,-2.01500291940243));
#27478=CARTESIAN_POINT('Ctrl Pts',(0.150696157673084,1.,-2.01500291940243));
#27479=CARTESIAN_POINT('Ctrl Pts',(0.148856124775343,-1.,-2.02083464969897));
#27480=CARTESIAN_POINT('Ctrl Pts',(0.148856124775343,1.,-2.02083464969897));
#27481=CARTESIAN_POINT('Ctrl Pts',(0.146965557332586,-1.,-2.02666926182017));
#27482=CARTESIAN_POINT('Ctrl Pts',(0.146965557332586,1.,-2.02666926182017));
#27483=CARTESIAN_POINT('Ctrl Pts',(0.145025140186058,-1.,-2.03250223739941));
#27484=CARTESIAN_POINT('Ctrl Pts',(0.145025140186058,1.,-2.03250223739941));
#27485=CARTESIAN_POINT('Ctrl Pts',(0.143035515058208,-1.,-2.03832911025913));
#27486=CARTESIAN_POINT('Ctrl Pts',(0.143035515058208,1.,-2.03832911025913));
#27487=CARTESIAN_POINT('Ctrl Pts',(0.140997332152545,-1.,-2.04414757947919));
#27488=CARTESIAN_POINT('Ctrl Pts',(0.140997332152545,1.,-2.04414757947919));
#27489=CARTESIAN_POINT('Ctrl Pts',(0.138911255368966,-1.,-2.04995762001333));
#27490=CARTESIAN_POINT('Ctrl Pts',(0.138911255368966,1.,-2.04995762001333));
#27491=CARTESIAN_POINT('Ctrl Pts',(0.136777941218044,-1.,-2.0557604441427));
#27492=CARTESIAN_POINT('Ctrl Pts',(0.136777941218044,1.,-2.0557604441427));
#27493=CARTESIAN_POINT('Ctrl Pts',(0.134598026192107,-1.,-2.06155781517844));
#27494=CARTESIAN_POINT('Ctrl Pts',(0.134598026192107,1.,-2.06155781517844));
#27495=CARTESIAN_POINT('Ctrl Pts',(0.13237211154771,-1.,-2.06735123910319));
#27496=CARTESIAN_POINT('Ctrl Pts',(0.13237211154771,1.,-2.06735123910319));
#27497=CARTESIAN_POINT('Ctrl Pts',(0.1301007483284,-1.,-2.07314114713047));
#27498=CARTESIAN_POINT('Ctrl Pts',(0.1301007483284,1.,-2.07314114713047));
#27499=CARTESIAN_POINT('Ctrl Pts',(0.127784445276116,-1.,-2.07892715110967));
#27500=CARTESIAN_POINT('Ctrl Pts',(0.127784445276116,1.,-2.07892715110967));
#27501=CARTESIAN_POINT('Ctrl Pts',(0.125423679412058,-1.,-2.08470840653628));
#27502=CARTESIAN_POINT('Ctrl Pts',(0.125423679412058,1.,-2.08470840653628));
#27503=CARTESIAN_POINT('Ctrl Pts',(0.123018905621083,-1.,-2.09048392424826));
#27504=CARTESIAN_POINT('Ctrl Pts',(0.123018905621083,1.,-2.09048392424826));
#27505=CARTESIAN_POINT('Ctrl Pts',(0.120570567965129,-1.,-2.09625292867756));
#27506=CARTESIAN_POINT('Ctrl Pts',(0.120570567965129,1.,-2.09625292867756));
#27507=CARTESIAN_POINT('Ctrl Pts',(0.118079107988368,-1.,-2.10201512132945));
#27508=CARTESIAN_POINT('Ctrl Pts',(0.118079107988368,1.,-2.10201512132945));
#27509=CARTESIAN_POINT('Ctrl Pts',(0.11554495768794,-1.,-2.10777050261359));
#27510=CARTESIAN_POINT('Ctrl Pts',(0.11554495768794,1.,-2.10777050261359));
#27511=CARTESIAN_POINT('Ctrl Pts',(0.112968534419746,-1.,-2.11351924490335));
#27512=CARTESIAN_POINT('Ctrl Pts',(0.112968534419746,1.,-2.11351924490335));
#27513=CARTESIAN_POINT('Ctrl Pts',(0.11035023613502,-1.,-2.11926155590849));
#27514=CARTESIAN_POINT('Ctrl Pts',(0.11035023613502,1.,-2.11926155590849));
#27515=CARTESIAN_POINT('Ctrl Pts',(0.107690435231068,-1.,-2.12499752306927));
#27516=CARTESIAN_POINT('Ctrl Pts',(0.107690435231068,1.,-2.12499752306927));
#27517=CARTESIAN_POINT('Ctrl Pts',(0.104989479152703,-1.,-2.1307270488718));
#27518=CARTESIAN_POINT('Ctrl Pts',(0.104989479152703,1.,-2.1307270488718));
#27519=CARTESIAN_POINT('Ctrl Pts',(0.102247700556064,-1.,-2.13644992667052));
#27520=CARTESIAN_POINT('Ctrl Pts',(0.102247700556064,1.,-2.13644992667052));
#27521=CARTESIAN_POINT('Ctrl Pts',(0.0994654261990743,-1.,-2.14216588395974));
#27522=CARTESIAN_POINT('Ctrl Pts',(0.0994654261990743,1.,-2.14216588395974));
#27523=CARTESIAN_POINT('Ctrl Pts',(0.0966429852305689,-1.,-2.14787463531864));
#27524=CARTESIAN_POINT('Ctrl Pts',(0.0966429852305689,1.,-2.14787463531864));
#27525=CARTESIAN_POINT('Ctrl Pts',(0.0937807218868345,-1.,-2.15357593978377));
#27526=CARTESIAN_POINT('Ctrl Pts',(0.0937807218868345,1.,-2.15357593978377));
#27527=CARTESIAN_POINT('Ctrl Pts',(0.0908789888108266,-1.,-2.15926961544808));
#27528=CARTESIAN_POINT('Ctrl Pts',(0.0908789888108266,1.,-2.15926961544808));
#27529=CARTESIAN_POINT('Ctrl Pts',(0.0879381291387823,-1.,-2.16495552645275));
#27530=CARTESIAN_POINT('Ctrl Pts',(0.0879381291387823,1.,-2.16495552645275));
#27531=CARTESIAN_POINT('Ctrl Pts',(0.0849584620835643,-1.,-2.17063357871031));
#27532=CARTESIAN_POINT('Ctrl Pts',(0.0849584620835643,1.,-2.17063357871031));
#27533=CARTESIAN_POINT('Ctrl Pts',(0.0819402680871939,-1.,-2.1763037121106));
#27534=CARTESIAN_POINT('Ctrl Pts',(0.0819402680871939,1.,-2.1763037121106));
#27535=CARTESIAN_POINT('Ctrl Pts',(0.0788837727683228,-1.,-2.18196589448304));
#27536=CARTESIAN_POINT('Ctrl Pts',(0.0788837727683228,1.,-2.18196589448304));
#27537=CARTESIAN_POINT('Ctrl Pts',(0.0757891465833411,-1.,-2.1876201139874));
#27538=CARTESIAN_POINT('Ctrl Pts',(0.0757891465833411,1.,-2.1876201139874));
#27539=CARTESIAN_POINT('Ctrl Pts',(0.0732830357304276,-1.,-2.19213712012956));
#27540=CARTESIAN_POINT('Ctrl Pts',(0.0732830357304276,1.,-2.19213712012956));
#27541=CARTESIAN_POINT('Ctrl Pts',(0.0713863779524627,-1.,-2.19552129483562));
#27542=CARTESIAN_POINT('Ctrl Pts',(0.0713863779524627,1.,-2.19552129483562));
#27543=CARTESIAN_POINT('Ctrl Pts',(0.0701143536324926,-1.,-2.19777582085261));
#27544=CARTESIAN_POINT('Ctrl Pts',(0.0701143536324926,1.,-2.19777582085261));
#27545=CARTESIAN_POINT('Ctrl Pts',(0.0694764450219584,-1.,-2.19890268624765));
#27546=CARTESIAN_POINT('Ctrl Pts',(0.0694764450219584,1.,-2.19890268624765));
#27547=CARTESIAN_POINT('',(0.163289472382896,1.,-1.74236521665491));
#27548=CARTESIAN_POINT('Ctrl Pts',(0.163289472382896,1.,-1.74236521665491));
#27549=CARTESIAN_POINT('Ctrl Pts',(0.163814161002474,1.,-1.74720349503904));
#27550=CARTESIAN_POINT('Ctrl Pts',(0.164834765708484,1.,-1.75666056640041));
#27551=CARTESIAN_POINT('Ctrl Pts',(0.166279355148738,1.,-1.77018771687692));
#27552=CARTESIAN_POINT('Ctrl Pts',(0.16803277280837,1.,-1.78690649988931));
#27553=CARTESIAN_POINT('Ctrl Pts',(0.169936923908078,1.,-1.80561530633924));
#27554=CARTESIAN_POINT('Ctrl Pts',(0.171554770207306,1.,-1.82215766815414));
#27555=CARTESIAN_POINT('Ctrl Pts',(0.17288944289442,1.,-1.83658380530747));
#27556=CARTESIAN_POINT('Ctrl Pts',(0.173946627589401,1.,-1.84898113200543));
#27557=CARTESIAN_POINT('Ctrl Pts',(0.174735259276856,1.,-1.85948367089838));
#27558=CARTESIAN_POINT('Ctrl Pts',(0.175268337590901,1.,-1.86828349694972));
#27559=CARTESIAN_POINT('Ctrl Pts',(0.175563480746205,1.,-1.87563767773249));
#27560=CARTESIAN_POINT('Ctrl Pts',(0.175644148889271,1.,-1.88188663144846));
#27561=CARTESIAN_POINT('Ctrl Pts',(0.175538155840286,1.,-1.88742606272818));
#27562=CARTESIAN_POINT('Ctrl Pts',(0.175274276190664,1.,-1.89264630198279));
#27563=CARTESIAN_POINT('Ctrl Pts',(0.174879405091277,1.,-1.89788101117148));
#27564=CARTESIAN_POINT('Ctrl Pts',(0.174375518661222,1.,-1.90335253863003));
#27565=CARTESIAN_POINT('Ctrl Pts',(0.173776635257984,1.,-1.90911693975475));
#27566=CARTESIAN_POINT('Ctrl Pts',(0.173090695383619,1.,-1.91511429159681));
#27567=CARTESIAN_POINT('Ctrl Pts',(0.172321621259557,1.,-1.92122334398034));
#27568=CARTESIAN_POINT('Ctrl Pts',(0.17147119153296,1.,-1.92731093582));
#27569=CARTESIAN_POINT('Ctrl Pts',(0.170541253116136,1.,-1.93329183155455));
#27570=CARTESIAN_POINT('Ctrl Pts',(0.169534904817425,1.,-1.93915639211497));
#27571=CARTESIAN_POINT('Ctrl Pts',(0.168455741607516,1.,-1.94493757756879));
#27572=CARTESIAN_POINT('Ctrl Pts',(0.167307501784469,1.,-1.95069027794286));
#27573=CARTESIAN_POINT('Ctrl Pts',(0.166093592002833,1.,-1.95646759718755));
#27574=CARTESIAN_POINT('Ctrl Pts',(0.1648165689203,1.,-1.96229379940174));
#27575=CARTESIAN_POINT('Ctrl Pts',(0.16347818545776,1.,-1.96816512678));
#27576=CARTESIAN_POINT('Ctrl Pts',(0.162079693556302,1.,-1.97406280235204));
#27577=CARTESIAN_POINT('Ctrl Pts',(0.16062206078461,1.,-1.97996195437557));
#27578=CARTESIAN_POINT('Ctrl Pts',(0.159106226437288,1.,-1.98584238283279));
#27579=CARTESIAN_POINT('Ctrl Pts',(0.157533331459215,1.,-1.99169810931893));
#27580=CARTESIAN_POINT('Ctrl Pts',(0.155904629548774,1.,-1.99753284771487));
#27581=CARTESIAN_POINT('Ctrl Pts',(0.154221403049719,1.,-2.00335565310539));
#27582=CARTESIAN_POINT('Ctrl Pts',(0.152484883621452,1.,-2.00917680318426));
#27583=CARTESIAN_POINT('Ctrl Pts',(0.150696157673084,1.,-2.01500291940243));
#27584=CARTESIAN_POINT('Ctrl Pts',(0.148856124775343,1.,-2.02083464969897));
#27585=CARTESIAN_POINT('Ctrl Pts',(0.146965557332586,1.,-2.02666926182017));
#27586=CARTESIAN_POINT('Ctrl Pts',(0.145025140186058,1.,-2.03250223739941));
#27587=CARTESIAN_POINT('Ctrl Pts',(0.143035515058208,1.,-2.03832911025913));
#27588=CARTESIAN_POINT('Ctrl Pts',(0.140997332152545,1.,-2.04414757947919));
#27589=CARTESIAN_POINT('Ctrl Pts',(0.138911255368966,1.,-2.04995762001333));
#27590=CARTESIAN_POINT('Ctrl Pts',(0.136777941218044,1.,-2.0557604441427));
#27591=CARTESIAN_POINT('Ctrl Pts',(0.134598026192107,1.,-2.06155781517844));
#27592=CARTESIAN_POINT('Ctrl Pts',(0.13237211154771,1.,-2.06735123910319));
#27593=CARTESIAN_POINT('Ctrl Pts',(0.1301007483284,1.,-2.07314114713047));
#27594=CARTESIAN_POINT('Ctrl Pts',(0.127784445276116,1.,-2.07892715110967));
#27595=CARTESIAN_POINT('Ctrl Pts',(0.125423679412058,1.,-2.08470840653628));
#27596=CARTESIAN_POINT('Ctrl Pts',(0.123018905621083,1.,-2.09048392424826));
#27597=CARTESIAN_POINT('Ctrl Pts',(0.120570567965129,1.,-2.09625292867756));
#27598=CARTESIAN_POINT('Ctrl Pts',(0.118079107988368,1.,-2.10201512132945));
#27599=CARTESIAN_POINT('Ctrl Pts',(0.11554495768794,1.,-2.10777050261359));
#27600=CARTESIAN_POINT('Ctrl Pts',(0.112968534419746,1.,-2.11351924490335));
#27601=CARTESIAN_POINT('Ctrl Pts',(0.11035023613502,1.,-2.11926155590849));
#27602=CARTESIAN_POINT('Ctrl Pts',(0.107690435231068,1.,-2.12499752306927));
#27603=CARTESIAN_POINT('Ctrl Pts',(0.104989479152703,1.,-2.1307270488718));
#27604=CARTESIAN_POINT('Ctrl Pts',(0.102247700556064,1.,-2.13644992667052));
#27605=CARTESIAN_POINT('Ctrl Pts',(0.0994654261990743,1.,-2.14216588395974));
#27606=CARTESIAN_POINT('Ctrl Pts',(0.0966429852305689,1.,-2.14787463531864));
#27607=CARTESIAN_POINT('Ctrl Pts',(0.0937807218868345,1.,-2.15357593978377));
#27608=CARTESIAN_POINT('Ctrl Pts',(0.0908789888108266,1.,-2.15926961544808));
#27609=CARTESIAN_POINT('Ctrl Pts',(0.0879381291387823,1.,-2.16495552645275));
#27610=CARTESIAN_POINT('Ctrl Pts',(0.0849584620835643,1.,-2.17063357871031));
#27611=CARTESIAN_POINT('Ctrl Pts',(0.0819402680871939,1.,-2.1763037121106));
#27612=CARTESIAN_POINT('Ctrl Pts',(0.0788837727683228,1.,-2.18196589448304));
#27613=CARTESIAN_POINT('Ctrl Pts',(0.0757891465833411,1.,-2.1876201139874));
#27614=CARTESIAN_POINT('Ctrl Pts',(0.0732830357304276,1.,-2.19213712012956));
#27615=CARTESIAN_POINT('Ctrl Pts',(0.0713863779524627,1.,-2.19552129483562));
#27616=CARTESIAN_POINT('Ctrl Pts',(0.0701143536324926,1.,-2.19777582085261));
#27617=CARTESIAN_POINT('Ctrl Pts',(0.0694764450219584,1.,-2.19890268624765));
#27618=CARTESIAN_POINT('',(0.163289472382896,0.,-1.74236521665491));
#27619=CARTESIAN_POINT('Origin',(0.,0.,0.));
#27620=CARTESIAN_POINT('',(0.383122945602004,1.,-1.7075470150345));
#27621=CARTESIAN_POINT('Origin',(0.,1.,0.));
#27622=CARTESIAN_POINT('',(0.383122945602004,0.,-1.7075470150345));
#27623=CARTESIAN_POINT('Ctrl Pts',(0.61342227326009,-1.,-2.11275013067528));
#27624=CARTESIAN_POINT('Ctrl Pts',(0.61342227326009,1.,-2.11275013067528));
#27625=CARTESIAN_POINT('Ctrl Pts',(0.61246736556225,-1.,-2.11187554260142));
#27626=CARTESIAN_POINT('Ctrl Pts',(0.61246736556225,1.,-2.11187554260142));
#27627=CARTESIAN_POINT('Ctrl Pts',(0.610560911691113,-1.,-2.11012443807661));
#27628=CARTESIAN_POINT('Ctrl Pts',(0.610560911691113,1.,-2.11012443807661));
#27629=CARTESIAN_POINT('Ctrl Pts',(0.607711315456826,-1.,-2.10749199615859));
#27630=CARTESIAN_POINT('Ctrl Pts',(0.607711315456826,1.,-2.10749199615859));
#27631=CARTESIAN_POINT('Ctrl Pts',(0.603932030738212,-1.,-2.10397049887709));
#27632=CARTESIAN_POINT('Ctrl Pts',(0.603932030738212,1.,-2.10397049887709));
#27633=CARTESIAN_POINT('Ctrl Pts',(0.599241616422144,-1.,-2.09954930865331));
#27634=CARTESIAN_POINT('Ctrl Pts',(0.599241616422144,1.,-2.09954930865331));
#27635=CARTESIAN_POINT('Ctrl Pts',(0.594585006052823,-1.,-2.09510876220501));
#27636=CARTESIAN_POINT('Ctrl Pts',(0.594585006052823,1.,-2.09510876220501));
#27637=CARTESIAN_POINT('Ctrl Pts',(0.589962365403189,-1.,-2.09064881812053));
#27638=CARTESIAN_POINT('Ctrl Pts',(0.589962365403189,1.,-2.09064881812053));
#27639=CARTESIAN_POINT('Ctrl Pts',(0.585373918990895,-1.,-2.086169437277));
#27640=CARTESIAN_POINT('Ctrl Pts',(0.585373918990895,1.,-2.086169437277));
#27641=CARTESIAN_POINT('Ctrl Pts',(0.580819952107256,-1.,-2.08167059018138));
#27642=CARTESIAN_POINT('Ctrl Pts',(0.580819952107256,1.,-2.08167059018138));
#27643=CARTESIAN_POINT('Ctrl Pts',(0.576300797416274,-1.,-2.07715226767361));
#27644=CARTESIAN_POINT('Ctrl Pts',(0.576300797416274,1.,-2.07715226767361));
#27645=CARTESIAN_POINT('Ctrl Pts',(0.571816823242411,-1.,-2.07261449292758));
#27646=CARTESIAN_POINT('Ctrl Pts',(0.571816823242411,1.,-2.07261449292758));
#27647=CARTESIAN_POINT('Ctrl Pts',(0.567368421181229,-1.,-2.06805732997383));
#27648=CARTESIAN_POINT('Ctrl Pts',(0.567368421181229,1.,-2.06805732997383));
#27649=CARTESIAN_POINT('Ctrl Pts',(0.562955993082574,-1.,-2.06348090160697));
#27650=CARTESIAN_POINT('Ctrl Pts',(0.562955993082574,1.,-2.06348090160697));
#27651=CARTESIAN_POINT('Ctrl Pts',(0.558579940185467,-1.,-2.05888537756571));
#27652=CARTESIAN_POINT('Ctrl Pts',(0.558579940185467,1.,-2.05888537756571));
#27653=CARTESIAN_POINT('Ctrl Pts',(0.554240657464109,-1.,-2.05427091604482));
#27654=CARTESIAN_POINT('Ctrl Pts',(0.554240657464109,1.,-2.05427091604482));
#27655=CARTESIAN_POINT('Ctrl Pts',(0.549938525150342,-1.,-2.04963761077974));
#27656=CARTESIAN_POINT('Ctrl Pts',(0.549938525150342,1.,-2.04963761077974));
#27657=CARTESIAN_POINT('Ctrl Pts',(0.545673903817348,-1.,-2.0449854471456));
#27658=CARTESIAN_POINT('Ctrl Pts',(0.545673903817348,1.,-2.0449854471456));
#27659=CARTESIAN_POINT('Ctrl Pts',(0.54144712061552,-1.,-2.0403142269048));
#27660=CARTESIAN_POINT('Ctrl Pts',(0.54144712061552,1.,-2.0403142269048));
#27661=CARTESIAN_POINT('Ctrl Pts',(0.537258489833134,-1.,-2.03562362953993));
#27662=CARTESIAN_POINT('Ctrl Pts',(0.537258489833134,1.,-2.03562362953993));
#27663=CARTESIAN_POINT('Ctrl Pts',(0.533108355132905,-1.,-2.03091336214401));
#27664=CARTESIAN_POINT('Ctrl Pts',(0.533108355132905,1.,-2.03091336214401));
#27665=CARTESIAN_POINT('Ctrl Pts',(0.52899712724191,-1.,-2.02618329083289));
#27666=CARTESIAN_POINT('Ctrl Pts',(0.52899712724191,1.,-2.02618329083289));
#27667=CARTESIAN_POINT('Ctrl Pts',(0.524925318333518,-1.,-2.02143356304712));
#27668=CARTESIAN_POINT('Ctrl Pts',(0.524925318333518,1.,-2.02143356304712));
#27669=CARTESIAN_POINT('Ctrl Pts',(0.520893590399428,-1.,-2.01666477917306));
#27670=CARTESIAN_POINT('Ctrl Pts',(0.520893590399428,1.,-2.01666477917306));
#27671=CARTESIAN_POINT('Ctrl Pts',(0.516902681728733,-1.,-2.01187773939257));
#27672=CARTESIAN_POINT('Ctrl Pts',(0.516902681728733,1.,-2.01187773939257));
#27673=CARTESIAN_POINT('Ctrl Pts',(0.512953306961813,-1.,-2.00707309946955));
#27674=CARTESIAN_POINT('Ctrl Pts',(0.512953306961813,1.,-2.00707309946955));
#27675=CARTESIAN_POINT('Ctrl Pts',(0.509046069886152,-1.,-2.00225107134733));
#27676=CARTESIAN_POINT('Ctrl Pts',(0.509046069886152,1.,-2.00225107134733));
#27677=CARTESIAN_POINT('Ctrl Pts',(0.505181361323011,-1.,-1.99741107463567));
#27678=CARTESIAN_POINT('Ctrl Pts',(0.505181361323011,1.,-1.99741107463567));
#27679=CARTESIAN_POINT('Ctrl Pts',(0.501359287727129,-1.,-1.9925514912615));
#27680=CARTESIAN_POINT('Ctrl Pts',(0.501359287727129,1.,-1.9925514912615));
#27681=CARTESIAN_POINT('Ctrl Pts',(0.497579909545564,-1.,-1.98767044752929));
#27682=CARTESIAN_POINT('Ctrl Pts',(0.497579909545564,1.,-1.98767044752929));
#27683=CARTESIAN_POINT('Ctrl Pts',(0.493843476541492,-1.,-1.9827665876182));
#27684=CARTESIAN_POINT('Ctrl Pts',(0.493843476541492,1.,-1.9827665876182));
#27685=CARTESIAN_POINT('Ctrl Pts',(0.490150627860955,-1.,-1.97783973019229));
#27686=CARTESIAN_POINT('Ctrl Pts',(0.490150627860955,1.,-1.97783973019229));
#27687=CARTESIAN_POINT('Ctrl Pts',(0.486502692907661,-1.,-1.97289186263272));
#27688=CARTESIAN_POINT('Ctrl Pts',(0.486502692907661,1.,-1.97289186263272));
#27689=CARTESIAN_POINT('Ctrl Pts',(0.482901662120686,-1.,-1.96792703422358));
#27690=CARTESIAN_POINT('Ctrl Pts',(0.482901662120686,1.,-1.96792703422358));
#27691=CARTESIAN_POINT('Ctrl Pts',(0.479349583074846,-1.,-1.96294933055938));
#27692=CARTESIAN_POINT('Ctrl Pts',(0.479349583074846,1.,-1.96294933055938));
#27693=CARTESIAN_POINT('Ctrl Pts',(0.475848034683171,-1.,-1.95796111148175));
#27694=CARTESIAN_POINT('Ctrl Pts',(0.475848034683171,1.,-1.95796111148175));
#27695=CARTESIAN_POINT('Ctrl Pts',(0.472397672264079,-1.,-1.95296148278136));
#27696=CARTESIAN_POINT('Ctrl Pts',(0.472397672264079,1.,-1.95296148278136));
#27697=CARTESIAN_POINT('Ctrl Pts',(0.468997482913158,-1.,-1.94794381136524));
#27698=CARTESIAN_POINT('Ctrl Pts',(0.468997482913158,1.,-1.94794381136524));
#27699=CARTESIAN_POINT('Ctrl Pts',(0.465645462026064,-1.,-1.94289794196205));
#27700=CARTESIAN_POINT('Ctrl Pts',(0.465645462026064,1.,-1.94289794196205));
#27701=CARTESIAN_POINT('Ctrl Pts',(0.462340031009087,-1.,-1.93781486640834));
#27702=CARTESIAN_POINT('Ctrl Pts',(0.462340031009087,1.,-1.93781486640834));
#27703=CARTESIAN_POINT('Ctrl Pts',(0.459081234547931,-1.,-1.93269066517936));
#27704=CARTESIAN_POINT('Ctrl Pts',(0.459081234547931,1.,-1.93269066517936));
#27705=CARTESIAN_POINT('Ctrl Pts',(0.455872005174335,-1.,-1.92753067150461));
#27706=CARTESIAN_POINT('Ctrl Pts',(0.455872005174335,1.,-1.92753067150461));
#27707=CARTESIAN_POINT('Ctrl Pts',(0.452719478359356,-1.,-1.9223538064847));
#27708=CARTESIAN_POINT('Ctrl Pts',(0.452719478359356,1.,-1.9223538064847));
#27709=CARTESIAN_POINT('Ctrl Pts',(0.449632260106572,-1.,-1.91718342555717));
#27710=CARTESIAN_POINT('Ctrl Pts',(0.449632260106572,1.,-1.91718342555717));
#27711=CARTESIAN_POINT('Ctrl Pts',(0.446617343485651,-1.,-1.91203699981095));
#27712=CARTESIAN_POINT('Ctrl Pts',(0.446617343485651,1.,-1.91203699981095));
#27713=CARTESIAN_POINT('Ctrl Pts',(0.44367755684917,-1.,-1.90691756144906));
#27714=CARTESIAN_POINT('Ctrl Pts',(0.44367755684917,1.,-1.90691756144906));
#27715=CARTESIAN_POINT('Ctrl Pts',(0.44080783370416,-1.,-1.90180124389137));
#27716=CARTESIAN_POINT('Ctrl Pts',(0.44080783370416,1.,-1.90180124389137));
#27717=CARTESIAN_POINT('Ctrl Pts',(0.437995003948443,-1.,-1.89663648956549));
#27718=CARTESIAN_POINT('Ctrl Pts',(0.437995003948443,1.,-1.89663648956549));
#27719=CARTESIAN_POINT('Ctrl Pts',(0.43522566096358,-1.,-1.89136993975585));
#27720=CARTESIAN_POINT('Ctrl Pts',(0.43522566096358,1.,-1.89136993975585));
#27721=CARTESIAN_POINT('Ctrl Pts',(0.432493038548833,-1.,-1.88596913666828));
#27722=CARTESIAN_POINT('Ctrl Pts',(0.432493038548833,1.,-1.88596913666828));
#27723=CARTESIAN_POINT('Ctrl Pts',(0.429803062482217,-1.,-1.88044229001779));
#27724=CARTESIAN_POINT('Ctrl Pts',(0.429803062482217,1.,-1.88044229001779));
#27725=CARTESIAN_POINT('Ctrl Pts',(0.427183828518743,-1.,-1.87486989291334));
#27726=CARTESIAN_POINT('Ctrl Pts',(0.427183828518743,1.,-1.87486989291334));
#27727=CARTESIAN_POINT('Ctrl Pts',(0.424678177290876,-1.,-1.8693780394412));
#27728=CARTESIAN_POINT('Ctrl Pts',(0.424678177290876,1.,-1.8693780394412));
#27729=CARTESIAN_POINT('Ctrl Pts',(0.422327307417884,-1.,-1.86408083333863));
#27730=CARTESIAN_POINT('Ctrl Pts',(0.422327307417884,1.,-1.86408083333863));
#27731=CARTESIAN_POINT('Ctrl Pts',(0.420157287975583,-1.,-1.8590328109667));
#27732=CARTESIAN_POINT('Ctrl Pts',(0.420157287975583,1.,-1.8590328109667));
#27733=CARTESIAN_POINT('Ctrl Pts',(0.418164129144045,-1.,-1.8541763285645));
#27734=CARTESIAN_POINT('Ctrl Pts',(0.418164129144045,1.,-1.8541763285645));
#27735=CARTESIAN_POINT('Ctrl Pts',(0.416300022039885,-1.,-1.84929312930314));
#27736=CARTESIAN_POINT('Ctrl Pts',(0.416300022039885,1.,-1.84929312930314));
#27737=CARTESIAN_POINT('Ctrl Pts',(0.414487438255542,-1.,-1.84405757074218));
#27738=CARTESIAN_POINT('Ctrl Pts',(0.414487438255542,1.,-1.84405757074218));
#27739=CARTESIAN_POINT('Ctrl Pts',(0.412633125322945,-1.,-1.8380895347617));
#27740=CARTESIAN_POINT('Ctrl Pts',(0.412633125322945,1.,-1.8380895347617));
#27741=CARTESIAN_POINT('Ctrl Pts',(0.410641256301276,-1.,-1.83100408895047));
#27742=CARTESIAN_POINT('Ctrl Pts',(0.410641256301276,1.,-1.83100408895047));
#27743=CARTESIAN_POINT('Ctrl Pts',(0.408428948106227,-1.,-1.82247022677562));
#27744=CARTESIAN_POINT('Ctrl Pts',(0.408428948106227,1.,-1.82247022677562));
#27745=CARTESIAN_POINT('Ctrl Pts',(0.405933518407175,-1.,-1.81223801812013));
#27746=CARTESIAN_POINT('Ctrl Pts',(0.405933518407175,1.,-1.81223801812013));
#27747=CARTESIAN_POINT('Ctrl Pts',(0.403107976163396,-1.,-1.80012077173238));
#27748=CARTESIAN_POINT('Ctrl Pts',(0.403107976163396,1.,-1.80012077173238));
#27749=CARTESIAN_POINT('Ctrl Pts',(0.399919403774155,-1.,-1.78598826343754));
#27750=CARTESIAN_POINT('Ctrl Pts',(0.399919403774155,1.,-1.78598826343754));
#27751=CARTESIAN_POINT('Ctrl Pts',(0.396346196110688,-1.,-1.76975560043442));
#27752=CARTESIAN_POINT('Ctrl Pts',(0.396346196110688,1.,-1.76975560043442));
#27753=CARTESIAN_POINT('Ctrl Pts',(0.392375812285395,-1.,-1.75137405310193));
#27754=CARTESIAN_POINT('Ctrl Pts',(0.392375812285395,1.,-1.75137405310193));
#27755=CARTESIAN_POINT('Ctrl Pts',(0.388877023502615,-1.,-1.73493170972829));
#27756=CARTESIAN_POINT('Ctrl Pts',(0.388877023502615,1.,-1.73493170972829));
#27757=CARTESIAN_POINT('Ctrl Pts',(0.386070790323281,-1.,-1.72162022244582));
#27758=CARTESIAN_POINT('Ctrl Pts',(0.386070790323281,1.,-1.72162022244582));
#27759=CARTESIAN_POINT('Ctrl Pts',(0.384119047314215,-1.,-1.71231062891398));
#27760=CARTESIAN_POINT('Ctrl Pts',(0.384119047314215,1.,-1.71231062891398));
#27761=CARTESIAN_POINT('Ctrl Pts',(0.383122945602004,-1.,-1.7075470150345));
#27762=CARTESIAN_POINT('Ctrl Pts',(0.383122945602004,1.,-1.7075470150345));
#27763=CARTESIAN_POINT('',(0.61342227326009,1.,-2.11275013067528));
#27764=CARTESIAN_POINT('Ctrl Pts',(0.61342227326009,1.,-2.11275013067528));
#27765=CARTESIAN_POINT('Ctrl Pts',(0.61246736556225,1.,-2.11187554260142));
#27766=CARTESIAN_POINT('Ctrl Pts',(0.610560911691113,1.,-2.11012443807661));
#27767=CARTESIAN_POINT('Ctrl Pts',(0.607711315456826,1.,-2.10749199615859));
#27768=CARTESIAN_POINT('Ctrl Pts',(0.603932030738212,1.,-2.10397049887709));
#27769=CARTESIAN_POINT('Ctrl Pts',(0.599241616422144,1.,-2.09954930865331));
#27770=CARTESIAN_POINT('Ctrl Pts',(0.594585006052823,1.,-2.09510876220501));
#27771=CARTESIAN_POINT('Ctrl Pts',(0.589962365403189,1.,-2.09064881812053));
#27772=CARTESIAN_POINT('Ctrl Pts',(0.585373918990895,1.,-2.086169437277));
#27773=CARTESIAN_POINT('Ctrl Pts',(0.580819952107256,1.,-2.08167059018138));
#27774=CARTESIAN_POINT('Ctrl Pts',(0.576300797416274,1.,-2.07715226767361));
#27775=CARTESIAN_POINT('Ctrl Pts',(0.571816823242411,1.,-2.07261449292758));
#27776=CARTESIAN_POINT('Ctrl Pts',(0.567368421181229,1.,-2.06805732997383));
#27777=CARTESIAN_POINT('Ctrl Pts',(0.562955993082574,1.,-2.06348090160697));
#27778=CARTESIAN_POINT('Ctrl Pts',(0.558579940185467,1.,-2.05888537756571));
#27779=CARTESIAN_POINT('Ctrl Pts',(0.554240657464109,1.,-2.05427091604482));
#27780=CARTESIAN_POINT('Ctrl Pts',(0.549938525150342,1.,-2.04963761077974));
#27781=CARTESIAN_POINT('Ctrl Pts',(0.545673903817348,1.,-2.0449854471456));
#27782=CARTESIAN_POINT('Ctrl Pts',(0.54144712061552,1.,-2.0403142269048));
#27783=CARTESIAN_POINT('Ctrl Pts',(0.537258489833134,1.,-2.03562362953993));
#27784=CARTESIAN_POINT('Ctrl Pts',(0.533108355132905,1.,-2.03091336214401));
#27785=CARTESIAN_POINT('Ctrl Pts',(0.52899712724191,1.,-2.02618329083289));
#27786=CARTESIAN_POINT('Ctrl Pts',(0.524925318333518,1.,-2.02143356304712));
#27787=CARTESIAN_POINT('Ctrl Pts',(0.520893590399428,1.,-2.01666477917306));
#27788=CARTESIAN_POINT('Ctrl Pts',(0.516902681728733,1.,-2.01187773939257));
#27789=CARTESIAN_POINT('Ctrl Pts',(0.512953306961813,1.,-2.00707309946955));
#27790=CARTESIAN_POINT('Ctrl Pts',(0.509046069886152,1.,-2.00225107134733));
#27791=CARTESIAN_POINT('Ctrl Pts',(0.505181361323011,1.,-1.99741107463567));
#27792=CARTESIAN_POINT('Ctrl Pts',(0.501359287727129,1.,-1.9925514912615));
#27793=CARTESIAN_POINT('Ctrl Pts',(0.497579909545564,1.,-1.98767044752929));
#27794=CARTESIAN_POINT('Ctrl Pts',(0.493843476541492,1.,-1.9827665876182));
#27795=CARTESIAN_POINT('Ctrl Pts',(0.490150627860955,1.,-1.97783973019229));
#27796=CARTESIAN_POINT('Ctrl Pts',(0.486502692907661,1.,-1.97289186263272));
#27797=CARTESIAN_POINT('Ctrl Pts',(0.482901662120686,1.,-1.96792703422358));
#27798=CARTESIAN_POINT('Ctrl Pts',(0.479349583074846,1.,-1.96294933055938));
#27799=CARTESIAN_POINT('Ctrl Pts',(0.475848034683171,1.,-1.95796111148175));
#27800=CARTESIAN_POINT('Ctrl Pts',(0.472397672264079,1.,-1.95296148278136));
#27801=CARTESIAN_POINT('Ctrl Pts',(0.468997482913158,1.,-1.94794381136524));
#27802=CARTESIAN_POINT('Ctrl Pts',(0.465645462026064,1.,-1.94289794196205));
#27803=CARTESIAN_POINT('Ctrl Pts',(0.462340031009087,1.,-1.93781486640834));
#27804=CARTESIAN_POINT('Ctrl Pts',(0.459081234547931,1.,-1.93269066517936));
#27805=CARTESIAN_POINT('Ctrl Pts',(0.455872005174335,1.,-1.92753067150461));
#27806=CARTESIAN_POINT('Ctrl Pts',(0.452719478359356,1.,-1.9223538064847));
#27807=CARTESIAN_POINT('Ctrl Pts',(0.449632260106572,1.,-1.91718342555717));
#27808=CARTESIAN_POINT('Ctrl Pts',(0.446617343485651,1.,-1.91203699981095));
#27809=CARTESIAN_POINT('Ctrl Pts',(0.44367755684917,1.,-1.90691756144906));
#27810=CARTESIAN_POINT('Ctrl Pts',(0.44080783370416,1.,-1.90180124389137));
#27811=CARTESIAN_POINT('Ctrl Pts',(0.437995003948443,1.,-1.89663648956549));
#27812=CARTESIAN_POINT('Ctrl Pts',(0.43522566096358,1.,-1.89136993975585));
#27813=CARTESIAN_POINT('Ctrl Pts',(0.432493038548833,1.,-1.88596913666828));
#27814=CARTESIAN_POINT('Ctrl Pts',(0.429803062482217,1.,-1.88044229001779));
#27815=CARTESIAN_POINT('Ctrl Pts',(0.427183828518743,1.,-1.87486989291334));
#27816=CARTESIAN_POINT('Ctrl Pts',(0.424678177290876,1.,-1.8693780394412));
#27817=CARTESIAN_POINT('Ctrl Pts',(0.422327307417884,1.,-1.86408083333863));
#27818=CARTESIAN_POINT('Ctrl Pts',(0.420157287975583,1.,-1.8590328109667));
#27819=CARTESIAN_POINT('Ctrl Pts',(0.418164129144045,1.,-1.8541763285645));
#27820=CARTESIAN_POINT('Ctrl Pts',(0.416300022039885,1.,-1.84929312930314));
#27821=CARTESIAN_POINT('Ctrl Pts',(0.414487438255542,1.,-1.84405757074218));
#27822=CARTESIAN_POINT('Ctrl Pts',(0.412633125322945,1.,-1.8380895347617));
#27823=CARTESIAN_POINT('Ctrl Pts',(0.410641256301276,1.,-1.83100408895047));
#27824=CARTESIAN_POINT('Ctrl Pts',(0.408428948106227,1.,-1.82247022677562));
#27825=CARTESIAN_POINT('Ctrl Pts',(0.405933518407175,1.,-1.81223801812013));
#27826=CARTESIAN_POINT('Ctrl Pts',(0.403107976163396,1.,-1.80012077173238));
#27827=CARTESIAN_POINT('Ctrl Pts',(0.399919403774155,1.,-1.78598826343754));
#27828=CARTESIAN_POINT('Ctrl Pts',(0.396346196110688,1.,-1.76975560043442));
#27829=CARTESIAN_POINT('Ctrl Pts',(0.392375812285395,1.,-1.75137405310193));
#27830=CARTESIAN_POINT('Ctrl Pts',(0.388877023502615,1.,-1.73493170972829));
#27831=CARTESIAN_POINT('Ctrl Pts',(0.386070790323281,1.,-1.72162022244582));
#27832=CARTESIAN_POINT('Ctrl Pts',(0.384119047314215,1.,-1.71231062891398));
#27833=CARTESIAN_POINT('Ctrl Pts',(0.383122945602004,1.,-1.7075470150345));
#27834=CARTESIAN_POINT('',(0.61342227326009,0.,-2.11275013067528));
#27835=CARTESIAN_POINT('Origin',(0.745574324794401,0.,-2.0698113262342));
#27836=CARTESIAN_POINT('',(0.745574324794401,1.,-2.0698113262342));
#27837=CARTESIAN_POINT('',(0.61342227326009,1.,-2.11275013067528));
#27838=CARTESIAN_POINT('',(0.745574324794401,0.,-2.0698113262342));
#27839=CARTESIAN_POINT('Ctrl Pts',(0.693717979106306,-1.,-1.60662857109684));
#27840=CARTESIAN_POINT('Ctrl Pts',(0.693717979106306,1.,-1.60662857109684));
#27841=CARTESIAN_POINT('Ctrl Pts',(0.695712097881194,-1.,-1.61106790958151));
#27842=CARTESIAN_POINT('Ctrl Pts',(0.695712097881194,1.,-1.61106790958151));
#27843=CARTESIAN_POINT('Ctrl Pts',(0.699605146405088,-1.,-1.61974673472612));
#27844=CARTESIAN_POINT('Ctrl Pts',(0.699605146405088,1.,-1.61974673472612));
#27845=CARTESIAN_POINT('Ctrl Pts',(0.705159151988319,-1.,-1.63216541664676));
#27846=CARTESIAN_POINT('Ctrl Pts',(0.705159151988319,1.,-1.63216541664676));
#27847=CARTESIAN_POINT('Ctrl Pts',(0.711993139355394,-1.,-1.64752408832016));
#27848=CARTESIAN_POINT('Ctrl Pts',(0.711993139355394,1.,-1.64752408832016));
#27849=CARTESIAN_POINT('Ctrl Pts',(0.719585433804282,-1.,-1.6647288055568));
#27850=CARTESIAN_POINT('Ctrl Pts',(0.719585433804282,1.,-1.6647288055568));
#27851=CARTESIAN_POINT('Ctrl Pts',(0.726235967997433,-1.,-1.67996158455503));
#27852=CARTESIAN_POINT('Ctrl Pts',(0.726235967997433,1.,-1.67996158455503));
#27853=CARTESIAN_POINT('Ctrl Pts',(0.731963238697195,-1.,-1.69326921975743));
#27854=CARTESIAN_POINT('Ctrl Pts',(0.731963238697195,1.,-1.69326921975743));
#27855=CARTESIAN_POINT('Ctrl Pts',(0.736799665724771,-1.,-1.70473309006121));
#27856=CARTESIAN_POINT('Ctrl Pts',(0.736799665724771,1.,-1.70473309006121));
#27857=CARTESIAN_POINT('Ctrl Pts',(0.740795162032087,-1.,-1.71447789751927));
#27858=CARTESIAN_POINT('Ctrl Pts',(0.740795162032087,1.,-1.71447789751927));
#27859=CARTESIAN_POINT('Ctrl Pts',(0.744021445433764,-1.,-1.7226822991693));
#27860=CARTESIAN_POINT('Ctrl Pts',(0.744021445433764,1.,-1.7226822991693));
#27861=CARTESIAN_POINT('Ctrl Pts',(0.746574710096436,-1.,-1.72958533647399));
#27862=CARTESIAN_POINT('Ctrl Pts',(0.746574710096436,1.,-1.72958533647399));
#27863=CARTESIAN_POINT('Ctrl Pts',(0.748582462954854,-1.,-1.73550351679848));
#27864=CARTESIAN_POINT('Ctrl Pts',(0.748582462954854,1.,-1.73550351679848));
#27865=CARTESIAN_POINT('Ctrl Pts',(0.75019343597954,-1.,-1.74080458266705));
#27866=CARTESIAN_POINT('Ctrl Pts',(0.75019343597954,1.,-1.74080458266705));
#27867=CARTESIAN_POINT('Ctrl Pts',(0.751555614163629,-1.,-1.74585086852298));
#27868=CARTESIAN_POINT('Ctrl Pts',(0.751555614163629,1.,-1.74585086852298));
#27869=CARTESIAN_POINT('Ctrl Pts',(0.752797683531377,-1.,-1.75095139468809));
#27870=CARTESIAN_POINT('Ctrl Pts',(0.752797683531377,1.,-1.75095139468809));
#27871=CARTESIAN_POINT('Ctrl Pts',(0.75400925402848,-1.,-1.75631083600175));
#27872=CARTESIAN_POINT('Ctrl Pts',(0.75400925402848,1.,-1.75631083600175));
#27873=CARTESIAN_POINT('Ctrl Pts',(0.755220979975262,-1.,-1.7619781724032));
#27874=CARTESIAN_POINT('Ctrl Pts',(0.755220979975262,1.,-1.7619781724032));
#27875=CARTESIAN_POINT('Ctrl Pts',(0.756421896028403,-1.,-1.76789396003141));
#27876=CARTESIAN_POINT('Ctrl Pts',(0.756421896028403,1.,-1.76789396003141));
#27877=CARTESIAN_POINT('Ctrl Pts',(0.757578264077238,-1.,-1.77394167108342));
#27878=CARTESIAN_POINT('Ctrl Pts',(0.757578264077238,1.,-1.77394167108342));
#27879=CARTESIAN_POINT('Ctrl Pts',(0.75865062667738,-1.,-1.77999411220912));
#27880=CARTESIAN_POINT('Ctrl Pts',(0.75865062667738,1.,-1.77999411220912));
#27881=CARTESIAN_POINT('Ctrl Pts',(0.759614401109868,-1.,-1.78596964884527));
#27882=CARTESIAN_POINT('Ctrl Pts',(0.759614401109868,1.,-1.78596964884527));
#27883=CARTESIAN_POINT('Ctrl Pts',(0.760469555880425,-1.,-1.79185815610802));
#27884=CARTESIAN_POINT('Ctrl Pts',(0.760469555880425,1.,-1.79185815610802));
#27885=CARTESIAN_POINT('Ctrl Pts',(0.761229695230359,-1.,-1.79768986997735));
#27886=CARTESIAN_POINT('Ctrl Pts',(0.761229695230359,1.,-1.79768986997735));
#27887=CARTESIAN_POINT('Ctrl Pts',(0.761915336443515,-1.,-1.80351583877334));
#27888=CARTESIAN_POINT('Ctrl Pts',(0.761915336443515,1.,-1.80351583877334));
#27889=CARTESIAN_POINT('Ctrl Pts',(0.762546129464036,-1.,-1.80938551463989));
#27890=CARTESIAN_POINT('Ctrl Pts',(0.762546129464036,1.,-1.80938551463989));
#27891=CARTESIAN_POINT('Ctrl Pts',(0.763132003836783,-1.,-1.81532118405566));
#27892=CARTESIAN_POINT('Ctrl Pts',(0.763132003836783,1.,-1.81532118405566));
#27893=CARTESIAN_POINT('Ctrl Pts',(0.763673465462854,-1.,-1.82131873145297));
#27894=CARTESIAN_POINT('Ctrl Pts',(0.763673465462854,1.,-1.82131873145297));
#27895=CARTESIAN_POINT('Ctrl Pts',(0.764165902606055,-1.,-1.8273599120008));
#27896=CARTESIAN_POINT('Ctrl Pts',(0.764165902606055,1.,-1.8273599120008));
#27897=CARTESIAN_POINT('Ctrl Pts',(0.764602549687845,-1.,-1.8334207722714));
#27898=CARTESIAN_POINT('Ctrl Pts',(0.764602549687845,1.,-1.8334207722714));
#27899=CARTESIAN_POINT('Ctrl Pts',(0.764978057881687,-1.,-1.83948181064823));
#27900=CARTESIAN_POINT('Ctrl Pts',(0.764978057881687,1.,-1.83948181064823));
#27901=CARTESIAN_POINT('Ctrl Pts',(0.765291664861971,-1.,-1.84553698875911));
#27902=CARTESIAN_POINT('Ctrl Pts',(0.765291664861971,1.,-1.84553698875911));
#27903=CARTESIAN_POINT('Ctrl Pts',(0.765545710619023,-1.,-1.85158945130054));
#27904=CARTESIAN_POINT('Ctrl Pts',(0.765545710619023,1.,-1.85158945130054));
#27905=CARTESIAN_POINT('Ctrl Pts',(0.765744212909305,-1.,-1.85764741390391));
#27906=CARTESIAN_POINT('Ctrl Pts',(0.765744212909305,1.,-1.85764741390391));
#27907=CARTESIAN_POINT('Ctrl Pts',(0.765891519092557,-1.,-1.86372027063315));
#27908=CARTESIAN_POINT('Ctrl Pts',(0.765891519092557,1.,-1.86372027063315));
#27909=CARTESIAN_POINT('Ctrl Pts',(0.765990708546111,-1.,-1.86981398314345));
#27910=CARTESIAN_POINT('Ctrl Pts',(0.765990708546111,1.,-1.86981398314345));
#27911=CARTESIAN_POINT('Ctrl Pts',(0.766042837036759,-1.,-1.87592888967886));
#27912=CARTESIAN_POINT('Ctrl Pts',(0.766042837036759,1.,-1.87592888967886));
#27913=CARTESIAN_POINT('Ctrl Pts',(0.766047794851868,-1.,-1.88206215302561));
#27914=CARTESIAN_POINT('Ctrl Pts',(0.766047794851868,1.,-1.88206215302561));
#27915=CARTESIAN_POINT('Ctrl Pts',(0.76600483706209,-1.,-1.88820926433409));
#27916=CARTESIAN_POINT('Ctrl Pts',(0.76600483706209,1.,-1.88820926433409));
#27917=CARTESIAN_POINT('Ctrl Pts',(0.765913193856979,-1.,-1.89436577771389));
#27918=CARTESIAN_POINT('Ctrl Pts',(0.765913193856979,1.,-1.89436577771389));
#27919=CARTESIAN_POINT('Ctrl Pts',(0.765772772593395,-1.,-1.90052930393599));
#27920=CARTESIAN_POINT('Ctrl Pts',(0.765772772593395,1.,-1.90052930393599));
#27921=CARTESIAN_POINT('Ctrl Pts',(0.765584196937936,-1.,-1.90669961402362));
#27922=CARTESIAN_POINT('Ctrl Pts',(0.765584196937936,1.,-1.90669961402362));
#27923=CARTESIAN_POINT('Ctrl Pts',(0.765348465884739,-1.,-1.91287765805174));
#27924=CARTESIAN_POINT('Ctrl Pts',(0.765348465884739,1.,-1.91287765805174));
#27925=CARTESIAN_POINT('Ctrl Pts',(0.765066729667095,-1.,-1.91906491634197));
#27926=CARTESIAN_POINT('Ctrl Pts',(0.765066729667095,1.,-1.91906491634197));
#27927=CARTESIAN_POINT('Ctrl Pts',(0.764740025488189,-1.,-1.92526263537041));
#27928=CARTESIAN_POINT('Ctrl Pts',(0.764740025488189,1.,-1.92526263537041));
#27929=CARTESIAN_POINT('Ctrl Pts',(0.764369010673889,-1.,-1.93147105496367));
#27930=CARTESIAN_POINT('Ctrl Pts',(0.764369010673889,1.,-1.93147105496367));
#27931=CARTESIAN_POINT('Ctrl Pts',(0.763954049121393,-1.,-1.93768964875867));
#27932=CARTESIAN_POINT('Ctrl Pts',(0.763954049121393,1.,-1.93768964875867));
#27933=CARTESIAN_POINT('Ctrl Pts',(0.76349533353858,-1.,-1.94391746617626));
#27934=CARTESIAN_POINT('Ctrl Pts',(0.76349533353858,1.,-1.94391746617626));
#27935=CARTESIAN_POINT('Ctrl Pts',(0.762992990878774,-1.,-1.95015342590025));
#27936=CARTESIAN_POINT('Ctrl Pts',(0.762992990878774,1.,-1.95015342590025));
#27937=CARTESIAN_POINT('Ctrl Pts',(0.762447203806263,-1.,-1.95639665309893));
#27938=CARTESIAN_POINT('Ctrl Pts',(0.762447203806263,1.,-1.95639665309893));
#27939=CARTESIAN_POINT('Ctrl Pts',(0.761858300014575,-1.,-1.96264672744229));
#27940=CARTESIAN_POINT('Ctrl Pts',(0.761858300014575,1.,-1.96264672744229));
#27941=CARTESIAN_POINT('Ctrl Pts',(0.761226690483986,-1.,-1.96890351582545));
#27942=CARTESIAN_POINT('Ctrl Pts',(0.761226690483986,1.,-1.96890351582545));
#27943=CARTESIAN_POINT('Ctrl Pts',(0.760552825409855,-1.,-1.97516705321521));
#27944=CARTESIAN_POINT('Ctrl Pts',(0.760552825409855,1.,-1.97516705321521));
#27945=CARTESIAN_POINT('Ctrl Pts',(0.759837147452135,-1.,-1.98143741418156));
#27946=CARTESIAN_POINT('Ctrl Pts',(0.759837147452135,1.,-1.98143741418156));
#27947=CARTESIAN_POINT('Ctrl Pts',(0.759080037802242,-1.,-1.98771456680806));
#27948=CARTESIAN_POINT('Ctrl Pts',(0.759080037802242,1.,-1.98771456680806));
#27949=CARTESIAN_POINT('Ctrl Pts',(0.758281796766377,-1.,-1.9939983109871));
#27950=CARTESIAN_POINT('Ctrl Pts',(0.758281796766377,1.,-1.9939983109871));
#27951=CARTESIAN_POINT('Ctrl Pts',(0.757442676862341,-1.,-2.00028834739072));
#27952=CARTESIAN_POINT('Ctrl Pts',(0.757442676862341,1.,-2.00028834739072));
#27953=CARTESIAN_POINT('Ctrl Pts',(0.756562904646496,-1.,-2.00658431587682));
#27954=CARTESIAN_POINT('Ctrl Pts',(0.756562904646496,1.,-2.00658431587682));
#27955=CARTESIAN_POINT('Ctrl Pts',(0.7556427049581,-1.,-2.01288584328149));
#27956=CARTESIAN_POINT('Ctrl Pts',(0.7556427049581,1.,-2.01288584328149));
#27957=CARTESIAN_POINT('Ctrl Pts',(0.75468233072352,-1.,-2.01919259406003));
#27958=CARTESIAN_POINT('Ctrl Pts',(0.75468233072352,1.,-2.01919259406003));
#27959=CARTESIAN_POINT('Ctrl Pts',(0.753682061113765,-1.,-2.02550428623587));
#27960=CARTESIAN_POINT('Ctrl Pts',(0.753682061113765,1.,-2.02550428623587));
#27961=CARTESIAN_POINT('Ctrl Pts',(0.752642180488104,-1.,-2.03182068456467));
#27962=CARTESIAN_POINT('Ctrl Pts',(0.752642180488104,1.,-2.03182068456467));
#27963=CARTESIAN_POINT('Ctrl Pts',(0.751562963361383,-1.,-2.03814160092173));
#27964=CARTESIAN_POINT('Ctrl Pts',(0.751562963361383,1.,-2.03814160092173));
#27965=CARTESIAN_POINT('Ctrl Pts',(0.750444657874758,-1.,-2.04446689147754));
#27966=CARTESIAN_POINT('Ctrl Pts',(0.750444657874758,1.,-2.04446689147754));
#27967=CARTESIAN_POINT('Ctrl Pts',(0.749287468663053,-1.,-2.05079645591606));
#27968=CARTESIAN_POINT('Ctrl Pts',(0.749287468663053,1.,-2.05079645591606));
#27969=CARTESIAN_POINT('Ctrl Pts',(0.748091554181101,-1.,-2.05713023030263));
#27970=CARTESIAN_POINT('Ctrl Pts',(0.748091554181101,1.,-2.05713023030263));
#27971=CARTESIAN_POINT('Ctrl Pts',(0.747103932785504,-1.,-2.06220058927162));
#27972=CARTESIAN_POINT('Ctrl Pts',(0.747103932785504,1.,-2.06220058927162));
#27973=CARTESIAN_POINT('Ctrl Pts',(0.746345871542695,-1.,-2.06600523016401));
#27974=CARTESIAN_POINT('Ctrl Pts',(0.746345871542695,1.,-2.06600523016401));
#27975=CARTESIAN_POINT('Ctrl Pts',(0.74583279137781,-1.,-2.06854248895575));
#27976=CARTESIAN_POINT('Ctrl Pts',(0.74583279137781,1.,-2.06854248895575));
#27977=CARTESIAN_POINT('Ctrl Pts',(0.745574324794401,-1.,-2.0698113262342));
#27978=CARTESIAN_POINT('Ctrl Pts',(0.745574324794401,1.,-2.0698113262342));
#27979=CARTESIAN_POINT('',(0.693717979106306,1.,-1.60662857109684));
#27980=CARTESIAN_POINT('Ctrl Pts',(0.693717979106306,1.,-1.60662857109684));
#27981=CARTESIAN_POINT('Ctrl Pts',(0.695712097881194,1.,-1.61106790958151));
#27982=CARTESIAN_POINT('Ctrl Pts',(0.699605146405088,1.,-1.61974673472612));
#27983=CARTESIAN_POINT('Ctrl Pts',(0.705159151988319,1.,-1.63216541664676));
#27984=CARTESIAN_POINT('Ctrl Pts',(0.711993139355394,1.,-1.64752408832016));
#27985=CARTESIAN_POINT('Ctrl Pts',(0.719585433804282,1.,-1.6647288055568));
#27986=CARTESIAN_POINT('Ctrl Pts',(0.726235967997433,1.,-1.67996158455503));
#27987=CARTESIAN_POINT('Ctrl Pts',(0.731963238697195,1.,-1.69326921975743));
#27988=CARTESIAN_POINT('Ctrl Pts',(0.736799665724771,1.,-1.70473309006121));
#27989=CARTESIAN_POINT('Ctrl Pts',(0.740795162032087,1.,-1.71447789751927));
#27990=CARTESIAN_POINT('Ctrl Pts',(0.744021445433764,1.,-1.7226822991693));
#27991=CARTESIAN_POINT('Ctrl Pts',(0.746574710096436,1.,-1.72958533647399));
#27992=CARTESIAN_POINT('Ctrl Pts',(0.748582462954854,1.,-1.73550351679848));
#27993=CARTESIAN_POINT('Ctrl Pts',(0.75019343597954,1.,-1.74080458266705));
#27994=CARTESIAN_POINT('Ctrl Pts',(0.751555614163629,1.,-1.74585086852298));
#27995=CARTESIAN_POINT('Ctrl Pts',(0.752797683531377,1.,-1.75095139468809));
#27996=CARTESIAN_POINT('Ctrl Pts',(0.75400925402848,1.,-1.75631083600175));
#27997=CARTESIAN_POINT('Ctrl Pts',(0.755220979975262,1.,-1.7619781724032));
#27998=CARTESIAN_POINT('Ctrl Pts',(0.756421896028403,1.,-1.76789396003141));
#27999=CARTESIAN_POINT('Ctrl Pts',(0.757578264077238,1.,-1.77394167108342));
#28000=CARTESIAN_POINT('Ctrl Pts',(0.75865062667738,1.,-1.77999411220912));
#28001=CARTESIAN_POINT('Ctrl Pts',(0.759614401109868,1.,-1.78596964884527));
#28002=CARTESIAN_POINT('Ctrl Pts',(0.760469555880425,1.,-1.79185815610802));
#28003=CARTESIAN_POINT('Ctrl Pts',(0.761229695230359,1.,-1.79768986997735));
#28004=CARTESIAN_POINT('Ctrl Pts',(0.761915336443515,1.,-1.80351583877334));
#28005=CARTESIAN_POINT('Ctrl Pts',(0.762546129464036,1.,-1.80938551463989));
#28006=CARTESIAN_POINT('Ctrl Pts',(0.763132003836783,1.,-1.81532118405566));
#28007=CARTESIAN_POINT('Ctrl Pts',(0.763673465462854,1.,-1.82131873145297));
#28008=CARTESIAN_POINT('Ctrl Pts',(0.764165902606055,1.,-1.8273599120008));
#28009=CARTESIAN_POINT('Ctrl Pts',(0.764602549687845,1.,-1.8334207722714));
#28010=CARTESIAN_POINT('Ctrl Pts',(0.764978057881687,1.,-1.83948181064823));
#28011=CARTESIAN_POINT('Ctrl Pts',(0.765291664861971,1.,-1.84553698875911));
#28012=CARTESIAN_POINT('Ctrl Pts',(0.765545710619023,1.,-1.85158945130054));
#28013=CARTESIAN_POINT('Ctrl Pts',(0.765744212909305,1.,-1.85764741390391));
#28014=CARTESIAN_POINT('Ctrl Pts',(0.765891519092557,1.,-1.86372027063315));
#28015=CARTESIAN_POINT('Ctrl Pts',(0.765990708546111,1.,-1.86981398314345));
#28016=CARTESIAN_POINT('Ctrl Pts',(0.766042837036759,1.,-1.87592888967886));
#28017=CARTESIAN_POINT('Ctrl Pts',(0.766047794851868,1.,-1.88206215302561));
#28018=CARTESIAN_POINT('Ctrl Pts',(0.76600483706209,1.,-1.88820926433409));
#28019=CARTESIAN_POINT('Ctrl Pts',(0.765913193856979,1.,-1.89436577771389));
#28020=CARTESIAN_POINT('Ctrl Pts',(0.765772772593395,1.,-1.90052930393599));
#28021=CARTESIAN_POINT('Ctrl Pts',(0.765584196937936,1.,-1.90669961402362));
#28022=CARTESIAN_POINT('Ctrl Pts',(0.765348465884739,1.,-1.91287765805174));
#28023=CARTESIAN_POINT('Ctrl Pts',(0.765066729667095,1.,-1.91906491634197));
#28024=CARTESIAN_POINT('Ctrl Pts',(0.764740025488189,1.,-1.92526263537041));
#28025=CARTESIAN_POINT('Ctrl Pts',(0.764369010673889,1.,-1.93147105496367));
#28026=CARTESIAN_POINT('Ctrl Pts',(0.763954049121393,1.,-1.93768964875867));
#28027=CARTESIAN_POINT('Ctrl Pts',(0.76349533353858,1.,-1.94391746617626));
#28028=CARTESIAN_POINT('Ctrl Pts',(0.762992990878774,1.,-1.95015342590025));
#28029=CARTESIAN_POINT('Ctrl Pts',(0.762447203806263,1.,-1.95639665309893));
#28030=CARTESIAN_POINT('Ctrl Pts',(0.761858300014575,1.,-1.96264672744229));
#28031=CARTESIAN_POINT('Ctrl Pts',(0.761226690483986,1.,-1.96890351582545));
#28032=CARTESIAN_POINT('Ctrl Pts',(0.760552825409855,1.,-1.97516705321521));
#28033=CARTESIAN_POINT('Ctrl Pts',(0.759837147452135,1.,-1.98143741418156));
#28034=CARTESIAN_POINT('Ctrl Pts',(0.759080037802242,1.,-1.98771456680806));
#28035=CARTESIAN_POINT('Ctrl Pts',(0.758281796766377,1.,-1.9939983109871));
#28036=CARTESIAN_POINT('Ctrl Pts',(0.757442676862341,1.,-2.00028834739072));
#28037=CARTESIAN_POINT('Ctrl Pts',(0.756562904646496,1.,-2.00658431587682));
#28038=CARTESIAN_POINT('Ctrl Pts',(0.7556427049581,1.,-2.01288584328149));
#28039=CARTESIAN_POINT('Ctrl Pts',(0.75468233072352,1.,-2.01919259406003));
#28040=CARTESIAN_POINT('Ctrl Pts',(0.753682061113765,1.,-2.02550428623587));
#28041=CARTESIAN_POINT('Ctrl Pts',(0.752642180488104,1.,-2.03182068456467));
#28042=CARTESIAN_POINT('Ctrl Pts',(0.751562963361383,1.,-2.03814160092173));
#28043=CARTESIAN_POINT('Ctrl Pts',(0.750444657874758,1.,-2.04446689147754));
#28044=CARTESIAN_POINT('Ctrl Pts',(0.749287468663053,1.,-2.05079645591606));
#28045=CARTESIAN_POINT('Ctrl Pts',(0.748091554181101,1.,-2.05713023030263));
#28046=CARTESIAN_POINT('Ctrl Pts',(0.747103932785504,1.,-2.06220058927162));
#28047=CARTESIAN_POINT('Ctrl Pts',(0.746345871542695,1.,-2.06600523016401));
#28048=CARTESIAN_POINT('Ctrl Pts',(0.74583279137781,1.,-2.06854248895575));
#28049=CARTESIAN_POINT('Ctrl Pts',(0.745574324794401,1.,-2.0698113262342));
#28050=CARTESIAN_POINT('',(0.693717979106306,0.,-1.60662857109684));
#28051=CARTESIAN_POINT('Origin',(0.,0.,0.));
#28052=CARTESIAN_POINT('',(0.892032620296855,1.,-1.5055822144029));
#28053=CARTESIAN_POINT('Origin',(0.,1.,0.));
#28054=CARTESIAN_POINT('',(0.892032620296855,0.,-1.5055822144029));
#28055=CARTESIAN_POINT('Ctrl Pts',(1.23627494547115,-1.,-1.81978687191668));
#28056=CARTESIAN_POINT('Ctrl Pts',(1.23627494547115,1.,-1.81978687191668));
#28057=CARTESIAN_POINT('Ctrl Pts',(1.23509651170476,-1.,-1.81925017193666));
#28058=CARTESIAN_POINT('Ctrl Pts',(1.23509651170476,1.,-1.81925017193666));
#28059=CARTESIAN_POINT('Ctrl Pts',(1.2327422452705,-1.,-1.81817389921279));
#28060=CARTESIAN_POINT('Ctrl Pts',(1.2327422452705,1.,-1.81817389921279));
#28061=CARTESIAN_POINT('Ctrl Pts',(1.2292186489137,-1.,-1.8165508718364));
#28062=CARTESIAN_POINT('Ctrl Pts',(1.2292186489137,1.,-1.8165508718364));
#28063=CARTESIAN_POINT('Ctrl Pts',(1.2245361330495,-1.,-1.81436959210434));
#28064=CARTESIAN_POINT('Ctrl Pts',(1.2245361330495,1.,-1.81436959210434));
#28065=CARTESIAN_POINT('Ctrl Pts',(1.21870906103557,-1.,-1.81161420806656));
#28066=CARTESIAN_POINT('Ctrl Pts',(1.21870906103557,1.,-1.81161420806656));
#28067=CARTESIAN_POINT('Ctrl Pts',(1.21290815708314,-1.,-1.80882996917129));
#28068=CARTESIAN_POINT('Ctrl Pts',(1.21290815708314,1.,-1.80882996917129));
#28069=CARTESIAN_POINT('Ctrl Pts',(1.20713356605475,-1.,-1.80601678480707));
#28070=CARTESIAN_POINT('Ctrl Pts',(1.20713356605475,1.,-1.80601678480707));
#28071=CARTESIAN_POINT('Ctrl Pts',(1.20138548938974,-1.,-1.80317454838603));
#28072=CARTESIAN_POINT('Ctrl Pts',(1.20138548938974,1.,-1.80317454838603));
#28073=CARTESIAN_POINT('Ctrl Pts',(1.19566418930242,-1.,-1.80030314369879));
#28074=CARTESIAN_POINT('Ctrl Pts',(1.19566418930242,1.,-1.80030314369879));
#28075=CARTESIAN_POINT('Ctrl Pts',(1.18996997934445,-1.,-1.79740245923478));
#28076=CARTESIAN_POINT('Ctrl Pts',(1.18996997934445,1.,-1.79740245923478));
#28077=CARTESIAN_POINT('Ctrl Pts',(1.18430321697432,-1.,-1.79447240321515));
#28078=CARTESIAN_POINT('Ctrl Pts',(1.18430321697432,1.,-1.79447240321515));
#28079=CARTESIAN_POINT('Ctrl Pts',(1.17866429440809,-1.,-1.79151291552689));
#28080=CARTESIAN_POINT('Ctrl Pts',(1.17866429440809,1.,-1.79151291552689));
#28081=CARTESIAN_POINT('Ctrl Pts',(1.17305363177328,-1.,-1.78852398877617));
#28082=CARTESIAN_POINT('Ctrl Pts',(1.17305363177328,1.,-1.78852398877617));
#28083=CARTESIAN_POINT('Ctrl Pts',(1.16747166312303,-1.,-1.78550566040443));
#28084=CARTESIAN_POINT('Ctrl Pts',(1.16747166312303,1.,-1.78550566040443));
#28085=CARTESIAN_POINT('Ctrl Pts',(1.16191881298499,-1.,-1.78245795881009));
#28086=CARTESIAN_POINT('Ctrl Pts',(1.16191881298499,1.,-1.78245795881009));
#28087=CARTESIAN_POINT('Ctrl Pts',(1.15639547194698,-1.,-1.77938085564275));
#28088=CARTESIAN_POINT('Ctrl Pts',(1.15639547194698,1.,-1.77938085564275));
#28089=CARTESIAN_POINT('Ctrl Pts',(1.15090197841514,-1.,-1.7762742255701));
#28090=CARTESIAN_POINT('Ctrl Pts',(1.15090197841514,1.,-1.7762742255701));
#28091=CARTESIAN_POINT('Ctrl Pts',(1.1454385822692,-1.,-1.77313777896194));
#28092=CARTESIAN_POINT('Ctrl Pts',(1.1454385822692,1.,-1.77313777896194));
#28093=CARTESIAN_POINT('Ctrl Pts',(1.14000548336975,-1.,-1.76997111386769));
#28094=CARTESIAN_POINT('Ctrl Pts',(1.14000548336975,1.,-1.76997111386769));
#28095=CARTESIAN_POINT('Ctrl Pts',(1.1346029180462,-1.,-1.76677384551862));
#28096=CARTESIAN_POINT('Ctrl Pts',(1.1346029180462,1.,-1.76677384551862));
#28097=CARTESIAN_POINT('Ctrl Pts',(1.12923123555075,-1.,-1.7635457196617));
#28098=CARTESIAN_POINT('Ctrl Pts',(1.12923123555075,1.,-1.7635457196617));
#28099=CARTESIAN_POINT('Ctrl Pts',(1.12389096855086,-1.,-1.76028671825096));
#28100=CARTESIAN_POINT('Ctrl Pts',(1.12389096855086,1.,-1.76028671825096));
#28101=CARTESIAN_POINT('Ctrl Pts',(1.11858293216763,-1.,-1.75699720772105));
#28102=CARTESIAN_POINT('Ctrl Pts',(1.11858293216763,1.,-1.75699720772105));
#28103=CARTESIAN_POINT('Ctrl Pts',(1.11330807582551,-1.,-1.7536777209463));
#28104=CARTESIAN_POINT('Ctrl Pts',(1.11330807582551,1.,-1.7536777209463));
#28105=CARTESIAN_POINT('Ctrl Pts',(1.10806728183007,-1.,-1.7503286607592));
#28106=CARTESIAN_POINT('Ctrl Pts',(1.10806728183007,1.,-1.7503286607592));
#28107=CARTESIAN_POINT('Ctrl Pts',(1.10286118991143,-1.,-1.74695004214923));
#28108=CARTESIAN_POINT('Ctrl Pts',(1.10286118991143,1.,-1.74695004214923));
#28109=CARTESIAN_POINT('Ctrl Pts',(1.09768999241225,-1.,-1.74354119236208));
#28110=CARTESIAN_POINT('Ctrl Pts',(1.09768999241225,1.,-1.74354119236208));
#28111=CARTESIAN_POINT('Ctrl Pts',(1.09255329056493,-1.,-1.74010053962247));
#28112=CARTESIAN_POINT('Ctrl Pts',(1.09255329056493,1.,-1.74010053962247));
#28113=CARTESIAN_POINT('Ctrl Pts',(1.08745056285427,-1.,-1.73662628326091));
#28114=CARTESIAN_POINT('Ctrl Pts',(1.08745056285427,1.,-1.73662628326091));
#28115=CARTESIAN_POINT('Ctrl Pts',(1.08238162784749,-1.,-1.73311705663407));
#28116=CARTESIAN_POINT('Ctrl Pts',(1.08238162784749,1.,-1.73311705663407));
#28117=CARTESIAN_POINT('Ctrl Pts',(1.0773470373727,-1.,-1.72957248977424));
#28118=CARTESIAN_POINT('Ctrl Pts',(1.0773470373727,1.,-1.72957248977424));
#28119=CARTESIAN_POINT('Ctrl Pts',(1.07234866990252,-1.,-1.72599406198488));
#28120=CARTESIAN_POINT('Ctrl Pts',(1.07234866990252,1.,-1.72599406198488));
#28121=CARTESIAN_POINT('Ctrl Pts',(1.06738966975462,-1.,-1.72238500928453));
#28122=CARTESIAN_POINT('Ctrl Pts',(1.06738966975462,1.,-1.72238500928453));
#28123=CARTESIAN_POINT('Ctrl Pts',(1.06247324680647,-1.,-1.71874858456904));
#28124=CARTESIAN_POINT('Ctrl Pts',(1.06247324680647,1.,-1.71874858456904));
#28125=CARTESIAN_POINT('Ctrl Pts',(1.05760163192479,-1.,-1.7150865442702));
#28126=CARTESIAN_POINT('Ctrl Pts',(1.05760163192479,1.,-1.7150865442702));
#28127=CARTESIAN_POINT('Ctrl Pts',(1.05277517202855,-1.,-1.71139783543989));
#28128=CARTESIAN_POINT('Ctrl Pts',(1.05277517202855,1.,-1.71139783543989));
#28129=CARTESIAN_POINT('Ctrl Pts',(1.04799085404995,-1.,-1.70767646263649));
#28130=CARTESIAN_POINT('Ctrl Pts',(1.04799085404995,1.,-1.70767646263649));
#28131=CARTESIAN_POINT('Ctrl Pts',(1.04324363334554,-1.,-1.70391338707982));
#28132=CARTESIAN_POINT('Ctrl Pts',(1.04324363334554,1.,-1.70391338707982));
#28133=CARTESIAN_POINT('Ctrl Pts',(1.03852922490789,-1.,-1.70010052930962));
#28134=CARTESIAN_POINT('Ctrl Pts',(1.03852922490789,1.,-1.70010052930962));
#28135=CARTESIAN_POINT('Ctrl Pts',(1.03384646003588,-1.,-1.69623414782771));
#28136=CARTESIAN_POINT('Ctrl Pts',(1.03384646003588,1.,-1.69623414782771));
#28137=CARTESIAN_POINT('Ctrl Pts',(1.02919977579147,-1.,-1.69231840863458));
#28138=CARTESIAN_POINT('Ctrl Pts',(1.02919977579147,1.,-1.69231840863458));
#28139=CARTESIAN_POINT('Ctrl Pts',(1.02460180535255,-1.,-1.68836910178447));
#28140=CARTESIAN_POINT('Ctrl Pts',(1.02460180535255,1.,-1.68836910178447));
#28141=CARTESIAN_POINT('Ctrl Pts',(1.02006795074201,-1.,-1.68440578021706));
#28142=CARTESIAN_POINT('Ctrl Pts',(1.02006795074201,1.,-1.68440578021706));
#28143=CARTESIAN_POINT('Ctrl Pts',(1.01561026162773,-1.,-1.68044289894798));
#28144=CARTESIAN_POINT('Ctrl Pts',(1.01561026162773,1.,-1.68044289894798));
#28145=CARTESIAN_POINT('Ctrl Pts',(1.01123236493511,-1.,-1.67648246776464));
#28146=CARTESIAN_POINT('Ctrl Pts',(1.01123236493511,1.,-1.67648246776464));
#28147=CARTESIAN_POINT('Ctrl Pts',(1.00692206696414,-1.,-1.67250335383293));
#28148=CARTESIAN_POINT('Ctrl Pts',(1.00692206696414,1.,-1.67250335383293));
#28149=CARTESIAN_POINT('Ctrl Pts',(1.00265091003727,-1.,-1.66846059277303));
#28150=CARTESIAN_POINT('Ctrl Pts',(1.00265091003727,1.,-1.66846059277303));
#28151=CARTESIAN_POINT('Ctrl Pts',(0.998389654952757,-1.,-1.66430758030376));
#28152=CARTESIAN_POINT('Ctrl Pts',(0.998389654952757,1.,-1.66430758030376));
#28153=CARTESIAN_POINT('Ctrl Pts',(0.994121836661305,-1.,-1.66001553809947));
#28154=CARTESIAN_POINT('Ctrl Pts',(0.994121836661305,1.,-1.66001553809947));
#28155=CARTESIAN_POINT('Ctrl Pts',(0.989855627854164,-1.,-1.65559044289699));
#28156=CARTESIAN_POINT('Ctrl Pts',(0.989855627854164,1.,-1.65559044289699));
#28157=CARTESIAN_POINT('Ctrl Pts',(0.98564262292082,-1.,-1.65110016612638));
#28158=CARTESIAN_POINT('Ctrl Pts',(0.98564262292082,1.,-1.65110016612638));
#28159=CARTESIAN_POINT('Ctrl Pts',(0.981562530939489,-1.,-1.64665139190656));
#28160=CARTESIAN_POINT('Ctrl Pts',(0.981562530939489,1.,-1.64665139190656));
#28161=CARTESIAN_POINT('Ctrl Pts',(0.977689794119416,-1.,-1.64233990826687));
#28162=CARTESIAN_POINT('Ctrl Pts',(0.977689794119416,1.,-1.64233990826687));
#28163=CARTESIAN_POINT('Ctrl Pts',(0.974066058287418,-1.,-1.63820952658144));
#28164=CARTESIAN_POINT('Ctrl Pts',(0.974066058287418,1.,-1.63820952658144));
#28165=CARTESIAN_POINT('Ctrl Pts',(0.970669715997509,-1.,-1.63420665729798));
#28166=CARTESIAN_POINT('Ctrl Pts',(0.970669715997509,1.,-1.63420665729798));
#28167=CARTESIAN_POINT('Ctrl Pts',(0.967387853230345,-1.,-1.63013849959462));
#28168=CARTESIAN_POINT('Ctrl Pts',(0.967387853230345,1.,-1.63013849959462));
#28169=CARTESIAN_POINT('Ctrl Pts',(0.964046107040535,-1.,-1.62571930670187));
#28170=CARTESIAN_POINT('Ctrl Pts',(0.964046107040535,1.,-1.62571930670187));
#28171=CARTESIAN_POINT('Ctrl Pts',(0.960438326101728,-1.,-1.62061638140221));
#28172=CARTESIAN_POINT('Ctrl Pts',(0.960438326101728,1.,-1.62061638140221));
#28173=CARTESIAN_POINT('Ctrl Pts',(0.95635442292067,-1.,-1.61449324337085));
#28174=CARTESIAN_POINT('Ctrl Pts',(0.95635442292067,1.,-1.61449324337085));
#28175=CARTESIAN_POINT('Ctrl Pts',(0.951613284356035,-1.,-1.60706069896936));
#28176=CARTESIAN_POINT('Ctrl Pts',(0.951613284356035,1.,-1.60706069896936));
#28177=CARTESIAN_POINT('Ctrl Pts',(0.946078063315257,-1.,-1.59810042043673));
#28178=CARTESIAN_POINT('Ctrl Pts',(0.946078063315257,1.,-1.59810042043673));
#28179=CARTESIAN_POINT('Ctrl Pts',(0.939646377893399,-1.,-1.58744937487176));
#28180=CARTESIAN_POINT('Ctrl Pts',(0.939646377893399,1.,-1.58744937487176));
#28181=CARTESIAN_POINT('Ctrl Pts',(0.932246680108685,-1.,-1.57499388382243));
#28182=CARTESIAN_POINT('Ctrl Pts',(0.932246680108685,1.,-1.57499388382243));
#28183=CARTESIAN_POINT('Ctrl Pts',(0.923832188944341,-1.,-1.56065988578893));
#28184=CARTESIAN_POINT('Ctrl Pts',(0.923832188944341,1.,-1.56065988578893));
#28185=CARTESIAN_POINT('Ctrl Pts',(0.914375919026456,-1.,-1.54440491149498));
#28186=CARTESIAN_POINT('Ctrl Pts',(0.914375919026456,1.,-1.54440491149498));
#28187=CARTESIAN_POINT('Ctrl Pts',(0.905967409625651,-1.,-1.52984849887993));
#28188=CARTESIAN_POINT('Ctrl Pts',(0.905967409625651,1.,-1.52984849887993));
#28189=CARTESIAN_POINT('Ctrl Pts',(0.89918504748351,-1.,-1.51805569590094));
#28190=CARTESIAN_POINT('Ctrl Pts',(0.89918504748351,1.,-1.51805569590094));
#28191=CARTESIAN_POINT('Ctrl Pts',(0.894452006964543,-1.,-1.50980486806688));
#28192=CARTESIAN_POINT('Ctrl Pts',(0.894452006964543,1.,-1.50980486806688));
#28193=CARTESIAN_POINT('Ctrl Pts',(0.892032620296855,-1.,-1.5055822144029));
#28194=CARTESIAN_POINT('Ctrl Pts',(0.892032620296855,1.,-1.5055822144029));
#28195=CARTESIAN_POINT('',(1.23627494547115,1.,-1.81978687191668));
#28196=CARTESIAN_POINT('Ctrl Pts',(1.23627494547115,1.,-1.81978687191668));
#28197=CARTESIAN_POINT('Ctrl Pts',(1.23509651170476,1.,-1.81925017193666));
#28198=CARTESIAN_POINT('Ctrl Pts',(1.2327422452705,1.,-1.81817389921279));
#28199=CARTESIAN_POINT('Ctrl Pts',(1.2292186489137,1.,-1.8165508718364));
#28200=CARTESIAN_POINT('Ctrl Pts',(1.2245361330495,1.,-1.81436959210434));
#28201=CARTESIAN_POINT('Ctrl Pts',(1.21870906103557,1.,-1.81161420806656));
#28202=CARTESIAN_POINT('Ctrl Pts',(1.21290815708314,1.,-1.80882996917129));
#28203=CARTESIAN_POINT('Ctrl Pts',(1.20713356605475,1.,-1.80601678480707));
#28204=CARTESIAN_POINT('Ctrl Pts',(1.20138548938974,1.,-1.80317454838603));
#28205=CARTESIAN_POINT('Ctrl Pts',(1.19566418930242,1.,-1.80030314369879));
#28206=CARTESIAN_POINT('Ctrl Pts',(1.18996997934445,1.,-1.79740245923478));
#28207=CARTESIAN_POINT('Ctrl Pts',(1.18430321697432,1.,-1.79447240321515));
#28208=CARTESIAN_POINT('Ctrl Pts',(1.17866429440809,1.,-1.79151291552689));
#28209=CARTESIAN_POINT('Ctrl Pts',(1.17305363177328,1.,-1.78852398877617));
#28210=CARTESIAN_POINT('Ctrl Pts',(1.16747166312303,1.,-1.78550566040443));
#28211=CARTESIAN_POINT('Ctrl Pts',(1.16191881298499,1.,-1.78245795881009));
#28212=CARTESIAN_POINT('Ctrl Pts',(1.15639547194698,1.,-1.77938085564275));
#28213=CARTESIAN_POINT('Ctrl Pts',(1.15090197841514,1.,-1.7762742255701));
#28214=CARTESIAN_POINT('Ctrl Pts',(1.1454385822692,1.,-1.77313777896194));
#28215=CARTESIAN_POINT('Ctrl Pts',(1.14000548336975,1.,-1.76997111386769));
#28216=CARTESIAN_POINT('Ctrl Pts',(1.1346029180462,1.,-1.76677384551862));
#28217=CARTESIAN_POINT('Ctrl Pts',(1.12923123555075,1.,-1.7635457196617));
#28218=CARTESIAN_POINT('Ctrl Pts',(1.12389096855086,1.,-1.76028671825096));
#28219=CARTESIAN_POINT('Ctrl Pts',(1.11858293216763,1.,-1.75699720772105));
#28220=CARTESIAN_POINT('Ctrl Pts',(1.11330807582551,1.,-1.7536777209463));
#28221=CARTESIAN_POINT('Ctrl Pts',(1.10806728183007,1.,-1.7503286607592));
#28222=CARTESIAN_POINT('Ctrl Pts',(1.10286118991143,1.,-1.74695004214923));
#28223=CARTESIAN_POINT('Ctrl Pts',(1.09768999241225,1.,-1.74354119236208));
#28224=CARTESIAN_POINT('Ctrl Pts',(1.09255329056493,1.,-1.74010053962247));
#28225=CARTESIAN_POINT('Ctrl Pts',(1.08745056285427,1.,-1.73662628326091));
#28226=CARTESIAN_POINT('Ctrl Pts',(1.08238162784749,1.,-1.73311705663407));
#28227=CARTESIAN_POINT('Ctrl Pts',(1.0773470373727,1.,-1.72957248977424));
#28228=CARTESIAN_POINT('Ctrl Pts',(1.07234866990252,1.,-1.72599406198488));
#28229=CARTESIAN_POINT('Ctrl Pts',(1.06738966975462,1.,-1.72238500928453));
#28230=CARTESIAN_POINT('Ctrl Pts',(1.06247324680647,1.,-1.71874858456904));
#28231=CARTESIAN_POINT('Ctrl Pts',(1.05760163192479,1.,-1.7150865442702));
#28232=CARTESIAN_POINT('Ctrl Pts',(1.05277517202855,1.,-1.71139783543989));
#28233=CARTESIAN_POINT('Ctrl Pts',(1.04799085404995,1.,-1.70767646263649));
#28234=CARTESIAN_POINT('Ctrl Pts',(1.04324363334554,1.,-1.70391338707982));
#28235=CARTESIAN_POINT('Ctrl Pts',(1.03852922490789,1.,-1.70010052930962));
#28236=CARTESIAN_POINT('Ctrl Pts',(1.03384646003588,1.,-1.69623414782771));
#28237=CARTESIAN_POINT('Ctrl Pts',(1.02919977579147,1.,-1.69231840863458));
#28238=CARTESIAN_POINT('Ctrl Pts',(1.02460180535255,1.,-1.68836910178447));
#28239=CARTESIAN_POINT('Ctrl Pts',(1.02006795074201,1.,-1.68440578021706));
#28240=CARTESIAN_POINT('Ctrl Pts',(1.01561026162773,1.,-1.68044289894798));
#28241=CARTESIAN_POINT('Ctrl Pts',(1.01123236493511,1.,-1.67648246776464));
#28242=CARTESIAN_POINT('Ctrl Pts',(1.00692206696414,1.,-1.67250335383293));
#28243=CARTESIAN_POINT('Ctrl Pts',(1.00265091003727,1.,-1.66846059277303));
#28244=CARTESIAN_POINT('Ctrl Pts',(0.998389654952757,1.,-1.66430758030376));
#28245=CARTESIAN_POINT('Ctrl Pts',(0.994121836661305,1.,-1.66001553809947));
#28246=CARTESIAN_POINT('Ctrl Pts',(0.989855627854164,1.,-1.65559044289699));
#28247=CARTESIAN_POINT('Ctrl Pts',(0.98564262292082,1.,-1.65110016612638));
#28248=CARTESIAN_POINT('Ctrl Pts',(0.981562530939489,1.,-1.64665139190656));
#28249=CARTESIAN_POINT('Ctrl Pts',(0.977689794119416,1.,-1.64233990826687));
#28250=CARTESIAN_POINT('Ctrl Pts',(0.974066058287418,1.,-1.63820952658144));
#28251=CARTESIAN_POINT('Ctrl Pts',(0.970669715997509,1.,-1.63420665729798));
#28252=CARTESIAN_POINT('Ctrl Pts',(0.967387853230345,1.,-1.63013849959462));
#28253=CARTESIAN_POINT('Ctrl Pts',(0.964046107040535,1.,-1.62571930670187));
#28254=CARTESIAN_POINT('Ctrl Pts',(0.960438326101728,1.,-1.62061638140221));
#28255=CARTESIAN_POINT('Ctrl Pts',(0.95635442292067,1.,-1.61449324337085));
#28256=CARTESIAN_POINT('Ctrl Pts',(0.951613284356035,1.,-1.60706069896936));
#28257=CARTESIAN_POINT('Ctrl Pts',(0.946078063315257,1.,-1.59810042043673));
#28258=CARTESIAN_POINT('Ctrl Pts',(0.939646377893399,1.,-1.58744937487176));
#28259=CARTESIAN_POINT('Ctrl Pts',(0.932246680108685,1.,-1.57499388382243));
#28260=CARTESIAN_POINT('Ctrl Pts',(0.923832188944341,1.,-1.56065988578893));
#28261=CARTESIAN_POINT('Ctrl Pts',(0.914375919026456,1.,-1.54440491149498));
#28262=CARTESIAN_POINT('Ctrl Pts',(0.905967409625651,1.,-1.52984849887993));
#28263=CARTESIAN_POINT('Ctrl Pts',(0.89918504748351,1.,-1.51805569590094));
#28264=CARTESIAN_POINT('Ctrl Pts',(0.894452006964543,1.,-1.50980486806688));
#28265=CARTESIAN_POINT('Ctrl Pts',(0.892032620296855,1.,-1.5055822144029));
#28266=CARTESIAN_POINT('',(1.23627494547115,0.,-1.81978687191668));
#28267=CARTESIAN_POINT('Origin',(1.34869019493419,0.,-1.73811241238545));
#28268=CARTESIAN_POINT('',(1.34869019493419,1.,-1.73811241238545));
#28269=CARTESIAN_POINT('',(1.23627494547115,1.,-1.81978687191668));
#28270=CARTESIAN_POINT('',(1.34869019493419,0.,-1.73811241238545));
#28271=CARTESIAN_POINT('Ctrl Pts',(1.15624053661742,-1.,-1.31362392696032));
#28272=CARTESIAN_POINT('Ctrl Pts',(1.15624053661742,1.,-1.31362392696032));
#28273=CARTESIAN_POINT('Ctrl Pts',(1.15950888730809,-1.,-1.31722977216397));
#28274=CARTESIAN_POINT('Ctrl Pts',(1.15950888730809,1.,-1.31722977216397));
#28275=CARTESIAN_POINT('Ctrl Pts',(1.16589330093588,-1.,-1.32428080721772));
#28276=CARTESIAN_POINT('Ctrl Pts',(1.16589330093588,1.,-1.32428080721772));
#28277=CARTESIAN_POINT('Ctrl Pts',(1.17501305789857,-1.,-1.33437539347008));
#28278=CARTESIAN_POINT('Ctrl Pts',(1.17501305789857,1.,-1.33437539347008));
#28279=CARTESIAN_POINT('Ctrl Pts',(1.18625865667441,-1.,-1.34687054001093));
#28280=CARTESIAN_POINT('Ctrl Pts',(1.18625865667441,1.,-1.34687054001093));
#28281=CARTESIAN_POINT('Ctrl Pts',(1.1987959077932,-1.,-1.36088705043885));
#28282=CARTESIAN_POINT('Ctrl Pts',(1.1987959077932,1.,-1.36088705043885));
#28283=CARTESIAN_POINT('Ctrl Pts',(1.20982812925645,-1.,-1.37331915607905));
#28284=CARTESIAN_POINT('Ctrl Pts',(1.20982812925645,1.,-1.37331915607905));
#28285=CARTESIAN_POINT('Ctrl Pts',(1.21938737280852,-1.,-1.38420564527715));
#28286=CARTESIAN_POINT('Ctrl Pts',(1.21938737280852,1.,-1.38420564527715));
#28287=CARTESIAN_POINT('Ctrl Pts',(1.22752961899387,-1.,-1.39361389568796));
#28288=CARTESIAN_POINT('Ctrl Pts',(1.22752961899387,1.,-1.39361389568796));
#28289=CARTESIAN_POINT('Ctrl Pts',(1.23434087290423,-1.,-1.40164708206106));
#28290=CARTESIAN_POINT('Ctrl Pts',(1.23434087290423,1.,-1.40164708206106));
#28291=CARTESIAN_POINT('Ctrl Pts',(1.23994455029534,-1.,-1.40845295531283));
#28292=CARTESIAN_POINT('Ctrl Pts',(1.23994455029534,1.,-1.40845295531283));
#28293=CARTESIAN_POINT('Ctrl Pts',(1.24450600513056,-1.,-1.41422913175179));
#28294=CARTESIAN_POINT('Ctrl Pts',(1.24450600513056,1.,-1.41422913175179));
#28295=CARTESIAN_POINT('Ctrl Pts',(1.24824430986571,-1.,-1.41923722596025));
#28296=CARTESIAN_POINT('Ctrl Pts',(1.24824430986571,1.,-1.41923722596025));
#28297=CARTESIAN_POINT('Ctrl Pts',(1.2514145557001,-1.,-1.42378102115575));
#28298=CARTESIAN_POINT('Ctrl Pts',(1.2514145557001,1.,-1.42378102115575));
#28299=CARTESIAN_POINT('Ctrl Pts',(1.25426945222639,-1.,-1.42815938799387));
#28300=CARTESIAN_POINT('Ctrl Pts',(1.25426945222639,1.,-1.42815938799387));
#28301=CARTESIAN_POINT('Ctrl Pts',(1.25702687965755,-1.,-1.43262645609691));
#28302=CARTESIAN_POINT('Ctrl Pts',(1.25702687965755,1.,-1.43262645609691));
#28303=CARTESIAN_POINT('Ctrl Pts',(1.25983531012005,-1.,-1.43734919180848));
#28304=CARTESIAN_POINT('Ctrl Pts',(1.25983531012005,1.,-1.43734919180848));
#28305=CARTESIAN_POINT('Ctrl Pts',(1.26273903323858,-1.,-1.44236470511303));
#28306=CARTESIAN_POINT('Ctrl Pts',(1.26273903323858,1.,-1.44236470511303));
#28307=CARTESIAN_POINT('Ctrl Pts',(1.26570925118868,-1.,-1.44761985001662));
#28308=CARTESIAN_POINT('Ctrl Pts',(1.26570925118868,1.,-1.44761985001662));
#28309=CARTESIAN_POINT('Ctrl Pts',(1.2686778680489,-1.,-1.45301422764247));
#28310=CARTESIAN_POINT('Ctrl Pts',(1.2686778680489,1.,-1.45301422764247));
#28311=CARTESIAN_POINT('Ctrl Pts',(1.27156805265289,-1.,-1.45843906294697));
#28312=CARTESIAN_POINT('Ctrl Pts',(1.27156805265289,1.,-1.45843906294697));
#28313=CARTESIAN_POINT('Ctrl Pts',(1.27433119897822,-1.,-1.46382431332476));
#28314=CARTESIAN_POINT('Ctrl Pts',(1.27433119897822,1.,-1.46382431332476));
#28315=CARTESIAN_POINT('Ctrl Pts',(1.27696414831089,-1.,-1.46916035917133));
#28316=CARTESIAN_POINT('Ctrl Pts',(1.27696414831089,1.,-1.46916035917133));
#28317=CARTESIAN_POINT('Ctrl Pts',(1.2794891824849,-1.,-1.4744717526707));
#28318=CARTESIAN_POINT('Ctrl Pts',(1.2794891824849,1.,-1.4744717526707));
#28319=CARTESIAN_POINT('Ctrl Pts',(1.28194158939517,-1.,-1.47980070347096));
#28320=CARTESIAN_POINT('Ctrl Pts',(1.28194158939517,1.,-1.47980070347096));
#28321=CARTESIAN_POINT('Ctrl Pts',(1.28435533880201,-1.,-1.4851881711891));
#28322=CARTESIAN_POINT('Ctrl Pts',(1.28435533880201,1.,-1.4851881711891));
#28323=CARTESIAN_POINT('Ctrl Pts',(1.2867467611644,-1.,-1.4906522831278));
#28324=CARTESIAN_POINT('Ctrl Pts',(1.2867467611644,1.,-1.4906522831278));
#28325=CARTESIAN_POINT('Ctrl Pts',(1.28911506584254,-1.,-1.49618896881754));
#28326=CARTESIAN_POINT('Ctrl Pts',(1.28911506584254,1.,-1.49618896881754));
#28327=CARTESIAN_POINT('Ctrl Pts',(1.29145022885181,-1.,-1.50178230149776));
#28328=CARTESIAN_POINT('Ctrl Pts',(1.29145022885181,1.,-1.50178230149776));
#28329=CARTESIAN_POINT('Ctrl Pts',(1.29373841372842,-1.,-1.50741159078365));
#28330=CARTESIAN_POINT('Ctrl Pts',(1.29373841372842,1.,-1.50741159078365));
#28331=CARTESIAN_POINT('Ctrl Pts',(1.29596850710509,-1.,-1.51305994241402));
#28332=CARTESIAN_POINT('Ctrl Pts',(1.29596850710509,1.,-1.51305994241402));
#28333=CARTESIAN_POINT('Ctrl Pts',(1.29813791800747,-1.,-1.51872184912724));
#28334=CARTESIAN_POINT('Ctrl Pts',(1.29813791800747,1.,-1.51872184912724));
#28335=CARTESIAN_POINT('Ctrl Pts',(1.30024984366328,-1.,-1.52439957861062));
#28336=CARTESIAN_POINT('Ctrl Pts',(1.30024984366328,1.,-1.52439957861062));
#28337=CARTESIAN_POINT('Ctrl Pts',(1.30231064395568,-1.,-1.53009970283891));
#28338=CARTESIAN_POINT('Ctrl Pts',(1.30231064395568,1.,-1.53009970283891));
#28339=CARTESIAN_POINT('Ctrl Pts',(1.30432735639489,-1.,-1.53582981268977));
#28340=CARTESIAN_POINT('Ctrl Pts',(1.30432735639489,1.,-1.53582981268977));
#28341=CARTESIAN_POINT('Ctrl Pts',(1.30630475189556,-1.,-1.54159462645432));
#28342=CARTESIAN_POINT('Ctrl Pts',(1.30630475189556,1.,-1.54159462645432));
#28343=CARTESIAN_POINT('Ctrl Pts',(1.30824393907473,-1.,-1.54739413957185));
#28344=CARTESIAN_POINT('Ctrl Pts',(1.30824393907473,1.,-1.54739413957185));
#28345=CARTESIAN_POINT('Ctrl Pts',(1.31014393684222,-1.,-1.55322568759481));
#28346=CARTESIAN_POINT('Ctrl Pts',(1.31014393684222,1.,-1.55322568759481));
#28347=CARTESIAN_POINT('Ctrl Pts',(1.31200264341696,-1.,-1.55908521254821));
#28348=CARTESIAN_POINT('Ctrl Pts',(1.31200264341696,1.,-1.55908521254821));
#28349=CARTESIAN_POINT('Ctrl Pts',(1.31381795281002,-1.,-1.56496872402353));
#28350=CARTESIAN_POINT('Ctrl Pts',(1.31381795281002,1.,-1.56496872402353));
#28351=CARTESIAN_POINT('Ctrl Pts',(1.31558903860016,-1.,-1.57087397835723));
#28352=CARTESIAN_POINT('Ctrl Pts',(1.31558903860016,1.,-1.57087397835723));
#28353=CARTESIAN_POINT('Ctrl Pts',(1.31731642317187,-1.,-1.5768005650559));
#28354=CARTESIAN_POINT('Ctrl Pts',(1.31731642317187,1.,-1.5768005650559));
#28355=CARTESIAN_POINT('Ctrl Pts',(1.31900135021432,-1.,-1.58274907898834));
#28356=CARTESIAN_POINT('Ctrl Pts',(1.31900135021432,1.,-1.58274907898834));
#28357=CARTESIAN_POINT('Ctrl Pts',(1.32064537110892,-1.,-1.58872057258245));
#28358=CARTESIAN_POINT('Ctrl Pts',(1.32064537110892,1.,-1.58872057258245));
#28359=CARTESIAN_POINT('Ctrl Pts',(1.32224985747682,-1.,-1.59471591079403));
#28360=CARTESIAN_POINT('Ctrl Pts',(1.32224985747682,1.,-1.59471591079403));
#28361=CARTESIAN_POINT('Ctrl Pts',(1.32381550858256,-1.,-1.60073511858687));
#28362=CARTESIAN_POINT('Ctrl Pts',(1.32381550858256,1.,-1.60073511858687));
#28363=CARTESIAN_POINT('Ctrl Pts',(1.32534250785782,-1.,-1.60677758290954));
#28364=CARTESIAN_POINT('Ctrl Pts',(1.32534250785782,1.,-1.60677758290954));
#28365=CARTESIAN_POINT('Ctrl Pts',(1.32683074483356,-1.,-1.6128423401575));
#28366=CARTESIAN_POINT('Ctrl Pts',(1.32683074483356,1.,-1.6128423401575));
#28367=CARTESIAN_POINT('Ctrl Pts',(1.32828000610449,-1.,-1.61892832270724));
#28368=CARTESIAN_POINT('Ctrl Pts',(1.32828000610449,1.,-1.61892832270724));
#28369=CARTESIAN_POINT('Ctrl Pts',(1.3296901950568,-1.,-1.62503464209797));
#28370=CARTESIAN_POINT('Ctrl Pts',(1.3296901950568,1.,-1.62503464209797));
#28371=CARTESIAN_POINT('Ctrl Pts',(1.33106149345645,-1.,-1.63116079730923));
#28372=CARTESIAN_POINT('Ctrl Pts',(1.33106149345645,1.,-1.63116079730923));
#28373=CARTESIAN_POINT('Ctrl Pts',(1.33239425103724,-1.,-1.63730653475089));
#28374=CARTESIAN_POINT('Ctrl Pts',(1.33239425103724,1.,-1.63730653475089));
#28375=CARTESIAN_POINT('Ctrl Pts',(1.33368890676572,-1.,-1.6434717485603));
#28376=CARTESIAN_POINT('Ctrl Pts',(1.33368890676572,1.,-1.6434717485603));
#28377=CARTESIAN_POINT('Ctrl Pts',(1.33494590467993,-1.,-1.6496563728683));
#28378=CARTESIAN_POINT('Ctrl Pts',(1.33494590467993,1.,-1.6496563728683));
#28379=CARTESIAN_POINT('Ctrl Pts',(1.33616559745172,-1.,-1.65586025952593));
#28380=CARTESIAN_POINT('Ctrl Pts',(1.33616559745172,1.,-1.65586025952593));
#28381=CARTESIAN_POINT('Ctrl Pts',(1.33734820885262,-1.,-1.66208312541983));
#28382=CARTESIAN_POINT('Ctrl Pts',(1.33734820885262,1.,-1.66208312541983));
#28383=CARTESIAN_POINT('Ctrl Pts',(1.33849388654388,-1.,-1.66832460783989));
#28384=CARTESIAN_POINT('Ctrl Pts',(1.33849388654388,1.,-1.66832460783989));
#28385=CARTESIAN_POINT('Ctrl Pts',(1.3396027347034,-1.,-1.67458429426086));
#28386=CARTESIAN_POINT('Ctrl Pts',(1.3396027347034,1.,-1.67458429426086));
#28387=CARTESIAN_POINT('Ctrl Pts',(1.34067485185203,-1.,-1.68086176030362));
#28388=CARTESIAN_POINT('Ctrl Pts',(1.34067485185203,1.,-1.68086176030362));
#28389=CARTESIAN_POINT('Ctrl Pts',(1.341710374848,-1.,-1.68715660868764));
#28390=CARTESIAN_POINT('Ctrl Pts',(1.341710374848,1.,-1.68715660868764));
#28391=CARTESIAN_POINT('Ctrl Pts',(1.34270948206319,-1.,-1.6934684849687));
#28392=CARTESIAN_POINT('Ctrl Pts',(1.34270948206319,1.,-1.6934684849687));
#28393=CARTESIAN_POINT('Ctrl Pts',(1.34367237124483,-1.,-1.69979707754427));
#28394=CARTESIAN_POINT('Ctrl Pts',(1.34367237124483,1.,-1.69979707754427));
#28395=CARTESIAN_POINT('Ctrl Pts',(1.34459924533831,-1.,-1.70614212266738));
#28396=CARTESIAN_POINT('Ctrl Pts',(1.34459924533831,1.,-1.70614212266738));
#28397=CARTESIAN_POINT('Ctrl Pts',(1.34549029589416,-1.,-1.71250340686822));
#28398=CARTESIAN_POINT('Ctrl Pts',(1.34549029589416,1.,-1.71250340686822));
#28399=CARTESIAN_POINT('Ctrl Pts',(1.34634568653227,-1.,-1.7188807715049));
#28400=CARTESIAN_POINT('Ctrl Pts',(1.34634568653227,1.,-1.7188807715049));
#28401=CARTESIAN_POINT('Ctrl Pts',(1.34716554819527,-1.,-1.72527410680674));
#28402=CARTESIAN_POINT('Ctrl Pts',(1.34716554819527,1.,-1.72527410680674));
#28403=CARTESIAN_POINT('Ctrl Pts',(1.34779309152035,-1.,-1.7304014965394));
#28404=CARTESIAN_POINT('Ctrl Pts',(1.34779309152035,1.,-1.7304014965394));
#28405=CARTESIAN_POINT('Ctrl Pts',(1.34824783112887,-1.,-1.73425417885907));
#28406=CARTESIAN_POINT('Ctrl Pts',(1.34824783112887,1.,-1.73425417885907));
#28407=CARTESIAN_POINT('Ctrl Pts',(1.34854391898045,-1.,-1.73682580585691));
#28408=CARTESIAN_POINT('Ctrl Pts',(1.34854391898045,1.,-1.73682580585691));
#28409=CARTESIAN_POINT('Ctrl Pts',(1.34869019493419,-1.,-1.73811241238545));
#28410=CARTESIAN_POINT('Ctrl Pts',(1.34869019493419,1.,-1.73811241238545));
#28411=CARTESIAN_POINT('',(1.15624053661742,1.,-1.31362392696032));
#28412=CARTESIAN_POINT('Ctrl Pts',(1.15624053661742,1.,-1.31362392696032));
#28413=CARTESIAN_POINT('Ctrl Pts',(1.15950888730809,1.,-1.31722977216397));
#28414=CARTESIAN_POINT('Ctrl Pts',(1.16589330093588,1.,-1.32428080721772));
#28415=CARTESIAN_POINT('Ctrl Pts',(1.17501305789857,1.,-1.33437539347008));
#28416=CARTESIAN_POINT('Ctrl Pts',(1.18625865667441,1.,-1.34687054001093));
#28417=CARTESIAN_POINT('Ctrl Pts',(1.1987959077932,1.,-1.36088705043885));
#28418=CARTESIAN_POINT('Ctrl Pts',(1.20982812925645,1.,-1.37331915607905));
#28419=CARTESIAN_POINT('Ctrl Pts',(1.21938737280852,1.,-1.38420564527715));
#28420=CARTESIAN_POINT('Ctrl Pts',(1.22752961899387,1.,-1.39361389568796));
#28421=CARTESIAN_POINT('Ctrl Pts',(1.23434087290423,1.,-1.40164708206106));
#28422=CARTESIAN_POINT('Ctrl Pts',(1.23994455029534,1.,-1.40845295531283));
#28423=CARTESIAN_POINT('Ctrl Pts',(1.24450600513056,1.,-1.41422913175179));
#28424=CARTESIAN_POINT('Ctrl Pts',(1.24824430986571,1.,-1.41923722596025));
#28425=CARTESIAN_POINT('Ctrl Pts',(1.2514145557001,1.,-1.42378102115575));
#28426=CARTESIAN_POINT('Ctrl Pts',(1.25426945222639,1.,-1.42815938799387));
#28427=CARTESIAN_POINT('Ctrl Pts',(1.25702687965755,1.,-1.43262645609691));
#28428=CARTESIAN_POINT('Ctrl Pts',(1.25983531012005,1.,-1.43734919180848));
#28429=CARTESIAN_POINT('Ctrl Pts',(1.26273903323858,1.,-1.44236470511303));
#28430=CARTESIAN_POINT('Ctrl Pts',(1.26570925118868,1.,-1.44761985001662));
#28431=CARTESIAN_POINT('Ctrl Pts',(1.2686778680489,1.,-1.45301422764247));
#28432=CARTESIAN_POINT('Ctrl Pts',(1.27156805265289,1.,-1.45843906294697));
#28433=CARTESIAN_POINT('Ctrl Pts',(1.27433119897822,1.,-1.46382431332476));
#28434=CARTESIAN_POINT('Ctrl Pts',(1.27696414831089,1.,-1.46916035917133));
#28435=CARTESIAN_POINT('Ctrl Pts',(1.2794891824849,1.,-1.4744717526707));
#28436=CARTESIAN_POINT('Ctrl Pts',(1.28194158939517,1.,-1.47980070347096));
#28437=CARTESIAN_POINT('Ctrl Pts',(1.28435533880201,1.,-1.4851881711891));
#28438=CARTESIAN_POINT('Ctrl Pts',(1.2867467611644,1.,-1.4906522831278));
#28439=CARTESIAN_POINT('Ctrl Pts',(1.28911506584254,1.,-1.49618896881754));
#28440=CARTESIAN_POINT('Ctrl Pts',(1.29145022885181,1.,-1.50178230149776));
#28441=CARTESIAN_POINT('Ctrl Pts',(1.29373841372842,1.,-1.50741159078365));
#28442=CARTESIAN_POINT('Ctrl Pts',(1.29596850710509,1.,-1.51305994241402));
#28443=CARTESIAN_POINT('Ctrl Pts',(1.29813791800747,1.,-1.51872184912724));
#28444=CARTESIAN_POINT('Ctrl Pts',(1.30024984366328,1.,-1.52439957861062));
#28445=CARTESIAN_POINT('Ctrl Pts',(1.30231064395568,1.,-1.53009970283891));
#28446=CARTESIAN_POINT('Ctrl Pts',(1.30432735639489,1.,-1.53582981268977));
#28447=CARTESIAN_POINT('Ctrl Pts',(1.30630475189556,1.,-1.54159462645432));
#28448=CARTESIAN_POINT('Ctrl Pts',(1.30824393907473,1.,-1.54739413957185));
#28449=CARTESIAN_POINT('Ctrl Pts',(1.31014393684222,1.,-1.55322568759481));
#28450=CARTESIAN_POINT('Ctrl Pts',(1.31200264341696,1.,-1.55908521254821));
#28451=CARTESIAN_POINT('Ctrl Pts',(1.31381795281002,1.,-1.56496872402353));
#28452=CARTESIAN_POINT('Ctrl Pts',(1.31558903860016,1.,-1.57087397835723));
#28453=CARTESIAN_POINT('Ctrl Pts',(1.31731642317187,1.,-1.5768005650559));
#28454=CARTESIAN_POINT('Ctrl Pts',(1.31900135021432,1.,-1.58274907898834));
#28455=CARTESIAN_POINT('Ctrl Pts',(1.32064537110892,1.,-1.58872057258245));
#28456=CARTESIAN_POINT('Ctrl Pts',(1.32224985747682,1.,-1.59471591079403));
#28457=CARTESIAN_POINT('Ctrl Pts',(1.32381550858256,1.,-1.60073511858687));
#28458=CARTESIAN_POINT('Ctrl Pts',(1.32534250785782,1.,-1.60677758290954));
#28459=CARTESIAN_POINT('Ctrl Pts',(1.32683074483356,1.,-1.6128423401575));
#28460=CARTESIAN_POINT('Ctrl Pts',(1.32828000610449,1.,-1.61892832270724));
#28461=CARTESIAN_POINT('Ctrl Pts',(1.3296901950568,1.,-1.62503464209797));
#28462=CARTESIAN_POINT('Ctrl Pts',(1.33106149345645,1.,-1.63116079730923));
#28463=CARTESIAN_POINT('Ctrl Pts',(1.33239425103724,1.,-1.63730653475089));
#28464=CARTESIAN_POINT('Ctrl Pts',(1.33368890676572,1.,-1.6434717485603));
#28465=CARTESIAN_POINT('Ctrl Pts',(1.33494590467993,1.,-1.6496563728683));
#28466=CARTESIAN_POINT('Ctrl Pts',(1.33616559745172,1.,-1.65586025952593));
#28467=CARTESIAN_POINT('Ctrl Pts',(1.33734820885262,1.,-1.66208312541983));
#28468=CARTESIAN_POINT('Ctrl Pts',(1.33849388654388,1.,-1.66832460783989));
#28469=CARTESIAN_POINT('Ctrl Pts',(1.3396027347034,1.,-1.67458429426086));
#28470=CARTESIAN_POINT('Ctrl Pts',(1.34067485185203,1.,-1.68086176030362));
#28471=CARTESIAN_POINT('Ctrl Pts',(1.341710374848,1.,-1.68715660868764));
#28472=CARTESIAN_POINT('Ctrl Pts',(1.34270948206319,1.,-1.6934684849687));
#28473=CARTESIAN_POINT('Ctrl Pts',(1.34367237124483,1.,-1.69979707754427));
#28474=CARTESIAN_POINT('Ctrl Pts',(1.34459924533831,1.,-1.70614212266738));
#28475=CARTESIAN_POINT('Ctrl Pts',(1.34549029589416,1.,-1.71250340686822));
#28476=CARTESIAN_POINT('Ctrl Pts',(1.34634568653227,1.,-1.7188807715049));
#28477=CARTESIAN_POINT('Ctrl Pts',(1.34716554819527,1.,-1.72527410680674));
#28478=CARTESIAN_POINT('Ctrl Pts',(1.34779309152035,1.,-1.7304014965394));
#28479=CARTESIAN_POINT('Ctrl Pts',(1.34824783112887,1.,-1.73425417885907));
#28480=CARTESIAN_POINT('Ctrl Pts',(1.34854391898045,1.,-1.73682580585691));
#28481=CARTESIAN_POINT('Ctrl Pts',(1.34869019493419,1.,-1.73811241238545));
#28482=CARTESIAN_POINT('',(1.15624053661742,0.,-1.31362392696032));
#28483=CARTESIAN_POINT('Origin',(0.,0.,0.));
#28484=CARTESIAN_POINT('',(1.31362392696032,1.,-1.15624053661742));
#28485=CARTESIAN_POINT('Origin',(0.,1.,0.));
#28486=CARTESIAN_POINT('',(1.31362392696032,0.,-1.15624053661742));
#28487=CARTESIAN_POINT('Ctrl Pts',(1.73811241238545,-1.,-1.34869019493419));
#28488=CARTESIAN_POINT('Ctrl Pts',(1.73811241238545,1.,-1.34869019493419));
#28489=CARTESIAN_POINT('Ctrl Pts',(1.73682580585819,-1.,-1.34854391898145));
#28490=CARTESIAN_POINT('Ctrl Pts',(1.73682580585819,1.,-1.34854391898145));
#28491=CARTESIAN_POINT('Ctrl Pts',(1.73425417886254,-1.,-1.34824783113158));
#28492=CARTESIAN_POINT('Ctrl Pts',(1.73425417886254,1.,-1.34824783113158));
#28493=CARTESIAN_POINT('Ctrl Pts',(1.73040149654497,-1.,-1.3477930915247));
#28494=CARTESIAN_POINT('Ctrl Pts',(1.73040149654497,1.,-1.3477930915247));
#28495=CARTESIAN_POINT('Ctrl Pts',(1.72527410681298,-1.,-1.34716554820013));
#28496=CARTESIAN_POINT('Ctrl Pts',(1.72527410681298,1.,-1.34716554820013));
#28497=CARTESIAN_POINT('Ctrl Pts',(1.7188807715095,-1.,-1.34634568653586));
#28498=CARTESIAN_POINT('Ctrl Pts',(1.7188807715095,1.,-1.34634568653586));
#28499=CARTESIAN_POINT('Ctrl Pts',(1.71250340687011,-1.,-1.34549029589563));
#28500=CARTESIAN_POINT('Ctrl Pts',(1.71250340687011,1.,-1.34549029589563));
#28501=CARTESIAN_POINT('Ctrl Pts',(1.70614212266676,-1.,-1.34459924533783));
#28502=CARTESIAN_POINT('Ctrl Pts',(1.70614212266676,1.,-1.34459924533783));
#28503=CARTESIAN_POINT('Ctrl Pts',(1.69979707754221,-1.,-1.34367237124322));
#28504=CARTESIAN_POINT('Ctrl Pts',(1.69979707754221,1.,-1.34367237124322));
#28505=CARTESIAN_POINT('Ctrl Pts',(1.6934684849664,-1.,-1.34270948206139));
#28506=CARTESIAN_POINT('Ctrl Pts',(1.6934684849664,1.,-1.34270948206139));
#28507=CARTESIAN_POINT('Ctrl Pts',(1.68715660868602,-1.,-1.34171037484673));
#28508=CARTESIAN_POINT('Ctrl Pts',(1.68715660868602,1.,-1.34171037484673));
#28509=CARTESIAN_POINT('Ctrl Pts',(1.68086176030308,-1.,-1.3406748518516));
#28510=CARTESIAN_POINT('Ctrl Pts',(1.68086176030308,1.,-1.3406748518516));
#28511=CARTESIAN_POINT('Ctrl Pts',(1.67458429426126,-1.,-1.33960273470372));
#28512=CARTESIAN_POINT('Ctrl Pts',(1.67458429426126,1.,-1.33960273470372));
#28513=CARTESIAN_POINT('Ctrl Pts',(1.66832460784078,-1.,-1.33849388654458));
#28514=CARTESIAN_POINT('Ctrl Pts',(1.66832460784078,1.,-1.33849388654458));
#28515=CARTESIAN_POINT('Ctrl Pts',(1.66208312542073,-1.,-1.33734820885331));
#28516=CARTESIAN_POINT('Ctrl Pts',(1.66208312542073,1.,-1.33734820885331));
#28517=CARTESIAN_POINT('Ctrl Pts',(1.65586025952651,-1.,-1.33616559745217));
#28518=CARTESIAN_POINT('Ctrl Pts',(1.65586025952651,1.,-1.33616559745217));
#28519=CARTESIAN_POINT('Ctrl Pts',(1.64965637286843,-1.,-1.33494590468003));
#28520=CARTESIAN_POINT('Ctrl Pts',(1.64965637286843,1.,-1.33494590468003));
#28521=CARTESIAN_POINT('Ctrl Pts',(1.64347174856007,-1.,-1.33368890676554));
#28522=CARTESIAN_POINT('Ctrl Pts',(1.64347174856007,1.,-1.33368890676554));
#28523=CARTESIAN_POINT('Ctrl Pts',(1.63730653475049,-1.,-1.33239425103694));
#28524=CARTESIAN_POINT('Ctrl Pts',(1.63730653475049,1.,-1.33239425103694));
#28525=CARTESIAN_POINT('Ctrl Pts',(1.63116079730887,-1.,-1.33106149345618));
#28526=CARTESIAN_POINT('Ctrl Pts',(1.63116079730887,1.,-1.33106149345618));
#28527=CARTESIAN_POINT('Ctrl Pts',(1.62503464209777,-1.,-1.32969019505665));
#28528=CARTESIAN_POINT('Ctrl Pts',(1.62503464209777,1.,-1.32969019505665));
#28529=CARTESIAN_POINT('Ctrl Pts',(1.61892832270723,-1.,-1.32828000610448));
#28530=CARTESIAN_POINT('Ctrl Pts',(1.61892832270723,1.,-1.32828000610448));
#28531=CARTESIAN_POINT('Ctrl Pts',(1.61284234015762,-1.,-1.32683074483365));
#28532=CARTESIAN_POINT('Ctrl Pts',(1.61284234015762,1.,-1.32683074483365));
#28533=CARTESIAN_POINT('Ctrl Pts',(1.6067775829097,-1.,-1.32534250785794));
#28534=CARTESIAN_POINT('Ctrl Pts',(1.6067775829097,1.,-1.32534250785794));
#28535=CARTESIAN_POINT('Ctrl Pts',(1.600735118587,-1.,-1.32381550858266));
#28536=CARTESIAN_POINT('Ctrl Pts',(1.600735118587,1.,-1.32381550858266));
#28537=CARTESIAN_POINT('Ctrl Pts',(1.59471591079408,-1.,-1.32224985747686));
#28538=CARTESIAN_POINT('Ctrl Pts',(1.59471591079408,1.,-1.32224985747686));
#28539=CARTESIAN_POINT('Ctrl Pts',(1.58872057258244,-1.,-1.32064537110891));
#28540=CARTESIAN_POINT('Ctrl Pts',(1.58872057258244,1.,-1.32064537110891));
#28541=CARTESIAN_POINT('Ctrl Pts',(1.58274907898829,-1.,-1.31900135021428));
#28542=CARTESIAN_POINT('Ctrl Pts',(1.58274907898829,1.,-1.31900135021428));
#28543=CARTESIAN_POINT('Ctrl Pts',(1.57680056505585,-1.,-1.31731642317183));
#28544=CARTESIAN_POINT('Ctrl Pts',(1.57680056505585,1.,-1.31731642317183));
#28545=CARTESIAN_POINT('Ctrl Pts',(1.57087397835721,-1.,-1.31558903860015));
#28546=CARTESIAN_POINT('Ctrl Pts',(1.57087397835721,1.,-1.31558903860015));
#28547=CARTESIAN_POINT('Ctrl Pts',(1.56496872402352,-1.,-1.31381795281002));
#28548=CARTESIAN_POINT('Ctrl Pts',(1.56496872402352,1.,-1.31381795281002));
#28549=CARTESIAN_POINT('Ctrl Pts',(1.55908521254822,-1.,-1.31200264341696));
#28550=CARTESIAN_POINT('Ctrl Pts',(1.55908521254822,1.,-1.31200264341696));
#28551=CARTESIAN_POINT('Ctrl Pts',(1.55322568759481,-1.,-1.31014393684221));
#28552=CARTESIAN_POINT('Ctrl Pts',(1.55322568759481,1.,-1.31014393684221));
#28553=CARTESIAN_POINT('Ctrl Pts',(1.54739413957183,-1.,-1.30824393907471));
#28554=CARTESIAN_POINT('Ctrl Pts',(1.54739413957183,1.,-1.30824393907471));
#28555=CARTESIAN_POINT('Ctrl Pts',(1.54159462645428,-1.,-1.30630475189553));
#28556=CARTESIAN_POINT('Ctrl Pts',(1.54159462645428,1.,-1.30630475189553));
#28557=CARTESIAN_POINT('Ctrl Pts',(1.53582981268976,-1.,-1.30432735639487));
#28558=CARTESIAN_POINT('Ctrl Pts',(1.53582981268976,1.,-1.30432735639487));
#28559=CARTESIAN_POINT('Ctrl Pts',(1.53009970283893,-1.,-1.3023106439557));
#28560=CARTESIAN_POINT('Ctrl Pts',(1.53009970283893,1.,-1.3023106439557));
#28561=CARTESIAN_POINT('Ctrl Pts',(1.5243995786107,-1.,-1.30024984366334));
#28562=CARTESIAN_POINT('Ctrl Pts',(1.5243995786107,1.,-1.30024984366334));
#28563=CARTESIAN_POINT('Ctrl Pts',(1.51872184912735,-1.,-1.29813791800757));
#28564=CARTESIAN_POINT('Ctrl Pts',(1.51872184912735,1.,-1.29813791800757));
#28565=CARTESIAN_POINT('Ctrl Pts',(1.51305994241412,-1.,-1.29596850710518));
#28566=CARTESIAN_POINT('Ctrl Pts',(1.51305994241412,1.,-1.29596850710518));
#28567=CARTESIAN_POINT('Ctrl Pts',(1.50741159078367,-1.,-1.29373841372843));
#28568=CARTESIAN_POINT('Ctrl Pts',(1.50741159078367,1.,-1.29373841372843));
#28569=CARTESIAN_POINT('Ctrl Pts',(1.50178230149764,-1.,-1.29145022885171));
#28570=CARTESIAN_POINT('Ctrl Pts',(1.50178230149764,1.,-1.29145022885171));
#28571=CARTESIAN_POINT('Ctrl Pts',(1.49618896881729,-1.,-1.28911506584232));
#28572=CARTESIAN_POINT('Ctrl Pts',(1.49618896881729,1.,-1.28911506584232));
#28573=CARTESIAN_POINT('Ctrl Pts',(1.4906522831275,-1.,-1.28674676116415));
#28574=CARTESIAN_POINT('Ctrl Pts',(1.4906522831275,1.,-1.28674676116415));
#28575=CARTESIAN_POINT('Ctrl Pts',(1.48518817118891,-1.,-1.28435533880184));
#28576=CARTESIAN_POINT('Ctrl Pts',(1.48518817118891,1.,-1.28435533880184));
#28577=CARTESIAN_POINT('Ctrl Pts',(1.47980070347102,-1.,-1.28194158939522));
#28578=CARTESIAN_POINT('Ctrl Pts',(1.47980070347102,1.,-1.28194158939522));
#28579=CARTESIAN_POINT('Ctrl Pts',(1.4744717526711,-1.,-1.27948918248524));
#28580=CARTESIAN_POINT('Ctrl Pts',(1.4744717526711,1.,-1.27948918248524));
#28581=CARTESIAN_POINT('Ctrl Pts',(1.46916035917197,-1.,-1.27696414831144));
#28582=CARTESIAN_POINT('Ctrl Pts',(1.46916035917197,1.,-1.27696414831144));
#28583=CARTESIAN_POINT('Ctrl Pts',(1.4638243133254,-1.,-1.27433119897877));
#28584=CARTESIAN_POINT('Ctrl Pts',(1.4638243133254,1.,-1.27433119897877));
#28585=CARTESIAN_POINT('Ctrl Pts',(1.45843906294725,-1.,-1.27156805265312));
#28586=CARTESIAN_POINT('Ctrl Pts',(1.45843906294725,1.,-1.27156805265312));
#28587=CARTESIAN_POINT('Ctrl Pts',(1.45301422764205,-1.,-1.26867786804854));
#28588=CARTESIAN_POINT('Ctrl Pts',(1.45301422764205,1.,-1.26867786804854));
#28589=CARTESIAN_POINT('Ctrl Pts',(1.44761985001544,-1.,-1.26570925118767));
#28590=CARTESIAN_POINT('Ctrl Pts',(1.44761985001544,1.,-1.26570925118767));
#28591=CARTESIAN_POINT('Ctrl Pts',(1.44236470511145,-1.,-1.26273903323723));
#28592=CARTESIAN_POINT('Ctrl Pts',(1.44236470511145,1.,-1.26273903323723));
#28593=CARTESIAN_POINT('Ctrl Pts',(1.43734919180719,-1.,-1.25983531011894));
#28594=CARTESIAN_POINT('Ctrl Pts',(1.43734919180719,1.,-1.25983531011894));
#28595=CARTESIAN_POINT('Ctrl Pts',(1.43262645609679,-1.,-1.25702687965744));
#28596=CARTESIAN_POINT('Ctrl Pts',(1.43262645609679,1.,-1.25702687965744));
#28597=CARTESIAN_POINT('Ctrl Pts',(1.42815938799555,-1.,-1.25426945222783));
#28598=CARTESIAN_POINT('Ctrl Pts',(1.42815938799555,1.,-1.25426945222783));
#28599=CARTESIAN_POINT('Ctrl Pts',(1.42378102115911,-1.,-1.25141455570299));
#28600=CARTESIAN_POINT('Ctrl Pts',(1.42378102115911,1.,-1.25141455570299));
#28601=CARTESIAN_POINT('Ctrl Pts',(1.41923722596421,-1.,-1.24824430986911));
#28602=CARTESIAN_POINT('Ctrl Pts',(1.41923722596421,1.,-1.24824430986911));
#28603=CARTESIAN_POINT('Ctrl Pts',(1.41422913175437,-1.,-1.24450600513278));
#28604=CARTESIAN_POINT('Ctrl Pts',(1.41422913175437,1.,-1.24450600513278));
#28605=CARTESIAN_POINT('Ctrl Pts',(1.40845295531151,-1.,-1.23994455029421));
#28606=CARTESIAN_POINT('Ctrl Pts',(1.40845295531151,1.,-1.23994455029421));
#28607=CARTESIAN_POINT('Ctrl Pts',(1.40164708205345,-1.,-1.23434087289768));
#28608=CARTESIAN_POINT('Ctrl Pts',(1.40164708205345,1.,-1.23434087289768));
#28609=CARTESIAN_POINT('Ctrl Pts',(1.39361389567257,-1.,-1.22752961898063));
#28610=CARTESIAN_POINT('Ctrl Pts',(1.39361389567257,1.,-1.22752961898063));
#28611=CARTESIAN_POINT('Ctrl Pts',(1.38420564525391,-1.,-1.21938737278853));
#28612=CARTESIAN_POINT('Ctrl Pts',(1.38420564525391,1.,-1.21938737278853));
#28613=CARTESIAN_POINT('Ctrl Pts',(1.37331915604962,-1.,-1.20982812923113));
#28614=CARTESIAN_POINT('Ctrl Pts',(1.37331915604962,1.,-1.20982812923113));
#28615=CARTESIAN_POINT('Ctrl Pts',(1.36088705040677,-1.,-1.1987959077656));
#28616=CARTESIAN_POINT('Ctrl Pts',(1.36088705040677,1.,-1.1987959077656));
#28617=CARTESIAN_POINT('Ctrl Pts',(1.34687053998157,-1.,-1.18625865664915));
#28618=CARTESIAN_POINT('Ctrl Pts',(1.34687053998157,1.,-1.18625865664915));
#28619=CARTESIAN_POINT('Ctrl Pts',(1.33437539344842,-1.,-1.17501305787994));
#28620=CARTESIAN_POINT('Ctrl Pts',(1.33437539344842,1.,-1.17501305787994));
#28621=CARTESIAN_POINT('Ctrl Pts',(1.32428080720544,-1.,-1.16589330092532));
#28622=CARTESIAN_POINT('Ctrl Pts',(1.32428080720544,1.,-1.16589330092532));
#28623=CARTESIAN_POINT('Ctrl Pts',(1.3172297721596,-1.,-1.15950888730433));
#28624=CARTESIAN_POINT('Ctrl Pts',(1.3172297721596,1.,-1.15950888730433));
#28625=CARTESIAN_POINT('Ctrl Pts',(1.31362392696032,-1.,-1.15624053661742));
#28626=CARTESIAN_POINT('Ctrl Pts',(1.31362392696032,1.,-1.15624053661742));
#28627=CARTESIAN_POINT('',(1.73811241238545,1.,-1.34869019493419));
#28628=CARTESIAN_POINT('Ctrl Pts',(1.73811241238545,1.,-1.34869019493419));
#28629=CARTESIAN_POINT('Ctrl Pts',(1.73682580585819,1.,-1.34854391898145));
#28630=CARTESIAN_POINT('Ctrl Pts',(1.73425417886254,1.,-1.34824783113158));
#28631=CARTESIAN_POINT('Ctrl Pts',(1.73040149654497,1.,-1.3477930915247));
#28632=CARTESIAN_POINT('Ctrl Pts',(1.72527410681298,1.,-1.34716554820013));
#28633=CARTESIAN_POINT('Ctrl Pts',(1.7188807715095,1.,-1.34634568653586));
#28634=CARTESIAN_POINT('Ctrl Pts',(1.71250340687011,1.,-1.34549029589563));
#28635=CARTESIAN_POINT('Ctrl Pts',(1.70614212266676,1.,-1.34459924533783));
#28636=CARTESIAN_POINT('Ctrl Pts',(1.69979707754221,1.,-1.34367237124322));
#28637=CARTESIAN_POINT('Ctrl Pts',(1.6934684849664,1.,-1.34270948206139));
#28638=CARTESIAN_POINT('Ctrl Pts',(1.68715660868602,1.,-1.34171037484673));
#28639=CARTESIAN_POINT('Ctrl Pts',(1.68086176030308,1.,-1.3406748518516));
#28640=CARTESIAN_POINT('Ctrl Pts',(1.67458429426126,1.,-1.33960273470372));
#28641=CARTESIAN_POINT('Ctrl Pts',(1.66832460784078,1.,-1.33849388654458));
#28642=CARTESIAN_POINT('Ctrl Pts',(1.66208312542073,1.,-1.33734820885331));
#28643=CARTESIAN_POINT('Ctrl Pts',(1.65586025952651,1.,-1.33616559745217));
#28644=CARTESIAN_POINT('Ctrl Pts',(1.64965637286843,1.,-1.33494590468003));
#28645=CARTESIAN_POINT('Ctrl Pts',(1.64347174856007,1.,-1.33368890676554));
#28646=CARTESIAN_POINT('Ctrl Pts',(1.63730653475049,1.,-1.33239425103694));
#28647=CARTESIAN_POINT('Ctrl Pts',(1.63116079730887,1.,-1.33106149345618));
#28648=CARTESIAN_POINT('Ctrl Pts',(1.62503464209777,1.,-1.32969019505665));
#28649=CARTESIAN_POINT('Ctrl Pts',(1.61892832270723,1.,-1.32828000610448));
#28650=CARTESIAN_POINT('Ctrl Pts',(1.61284234015762,1.,-1.32683074483365));
#28651=CARTESIAN_POINT('Ctrl Pts',(1.6067775829097,1.,-1.32534250785794));
#28652=CARTESIAN_POINT('Ctrl Pts',(1.600735118587,1.,-1.32381550858266));
#28653=CARTESIAN_POINT('Ctrl Pts',(1.59471591079408,1.,-1.32224985747686));
#28654=CARTESIAN_POINT('Ctrl Pts',(1.58872057258244,1.,-1.32064537110891));
#28655=CARTESIAN_POINT('Ctrl Pts',(1.58274907898829,1.,-1.31900135021428));
#28656=CARTESIAN_POINT('Ctrl Pts',(1.57680056505585,1.,-1.31731642317183));
#28657=CARTESIAN_POINT('Ctrl Pts',(1.57087397835721,1.,-1.31558903860015));
#28658=CARTESIAN_POINT('Ctrl Pts',(1.56496872402352,1.,-1.31381795281002));
#28659=CARTESIAN_POINT('Ctrl Pts',(1.55908521254822,1.,-1.31200264341696));
#28660=CARTESIAN_POINT('Ctrl Pts',(1.55322568759481,1.,-1.31014393684221));
#28661=CARTESIAN_POINT('Ctrl Pts',(1.54739413957183,1.,-1.30824393907471));
#28662=CARTESIAN_POINT('Ctrl Pts',(1.54159462645428,1.,-1.30630475189553));
#28663=CARTESIAN_POINT('Ctrl Pts',(1.53582981268976,1.,-1.30432735639487));
#28664=CARTESIAN_POINT('Ctrl Pts',(1.53009970283893,1.,-1.3023106439557));
#28665=CARTESIAN_POINT('Ctrl Pts',(1.5243995786107,1.,-1.30024984366334));
#28666=CARTESIAN_POINT('Ctrl Pts',(1.51872184912735,1.,-1.29813791800757));
#28667=CARTESIAN_POINT('Ctrl Pts',(1.51305994241412,1.,-1.29596850710518));
#28668=CARTESIAN_POINT('Ctrl Pts',(1.50741159078367,1.,-1.29373841372843));
#28669=CARTESIAN_POINT('Ctrl Pts',(1.50178230149764,1.,-1.29145022885171));
#28670=CARTESIAN_POINT('Ctrl Pts',(1.49618896881729,1.,-1.28911506584232));
#28671=CARTESIAN_POINT('Ctrl Pts',(1.4906522831275,1.,-1.28674676116415));
#28672=CARTESIAN_POINT('Ctrl Pts',(1.48518817118891,1.,-1.28435533880184));
#28673=CARTESIAN_POINT('Ctrl Pts',(1.47980070347102,1.,-1.28194158939522));
#28674=CARTESIAN_POINT('Ctrl Pts',(1.4744717526711,1.,-1.27948918248524));
#28675=CARTESIAN_POINT('Ctrl Pts',(1.46916035917197,1.,-1.27696414831144));
#28676=CARTESIAN_POINT('Ctrl Pts',(1.4638243133254,1.,-1.27433119897877));
#28677=CARTESIAN_POINT('Ctrl Pts',(1.45843906294725,1.,-1.27156805265312));
#28678=CARTESIAN_POINT('Ctrl Pts',(1.45301422764205,1.,-1.26867786804854));
#28679=CARTESIAN_POINT('Ctrl Pts',(1.44761985001544,1.,-1.26570925118767));
#28680=CARTESIAN_POINT('Ctrl Pts',(1.44236470511145,1.,-1.26273903323723));
#28681=CARTESIAN_POINT('Ctrl Pts',(1.43734919180719,1.,-1.25983531011894));
#28682=CARTESIAN_POINT('Ctrl Pts',(1.43262645609679,1.,-1.25702687965744));
#28683=CARTESIAN_POINT('Ctrl Pts',(1.42815938799555,1.,-1.25426945222783));
#28684=CARTESIAN_POINT('Ctrl Pts',(1.42378102115911,1.,-1.25141455570299));
#28685=CARTESIAN_POINT('Ctrl Pts',(1.41923722596421,1.,-1.24824430986911));
#28686=CARTESIAN_POINT('Ctrl Pts',(1.41422913175437,1.,-1.24450600513278));
#28687=CARTESIAN_POINT('Ctrl Pts',(1.40845295531151,1.,-1.23994455029421));
#28688=CARTESIAN_POINT('Ctrl Pts',(1.40164708205345,1.,-1.23434087289768));
#28689=CARTESIAN_POINT('Ctrl Pts',(1.39361389567257,1.,-1.22752961898063));
#28690=CARTESIAN_POINT('Ctrl Pts',(1.38420564525391,1.,-1.21938737278853));
#28691=CARTESIAN_POINT('Ctrl Pts',(1.37331915604962,1.,-1.20982812923113));
#28692=CARTESIAN_POINT('Ctrl Pts',(1.36088705040677,1.,-1.1987959077656));
#28693=CARTESIAN_POINT('Ctrl Pts',(1.34687053998157,1.,-1.18625865664915));
#28694=CARTESIAN_POINT('Ctrl Pts',(1.33437539344842,1.,-1.17501305787994));
#28695=CARTESIAN_POINT('Ctrl Pts',(1.32428080720544,1.,-1.16589330092532));
#28696=CARTESIAN_POINT('Ctrl Pts',(1.3172297721596,1.,-1.15950888730433));
#28697=CARTESIAN_POINT('Ctrl Pts',(1.31362392696032,1.,-1.15624053661742));
#28698=CARTESIAN_POINT('',(1.73811241238545,0.,-1.34869019493419));
#28699=CARTESIAN_POINT('Origin',(1.81978687191668,0.,-1.23627494547115));
#28700=CARTESIAN_POINT('',(1.81978687191668,1.,-1.23627494547115));
#28701=CARTESIAN_POINT('',(1.73811241238545,1.,-1.34869019493419));
#28702=CARTESIAN_POINT('',(1.81978687191668,0.,-1.23627494547115));
#28703=CARTESIAN_POINT('Ctrl Pts',(1.5055822144029,-1.,-0.892032620296855));
#28704=CARTESIAN_POINT('Ctrl Pts',(1.5055822144029,1.,-0.892032620296855));
#28705=CARTESIAN_POINT('Ctrl Pts',(1.50980486807181,-1.,-0.894452006967538));
#28706=CARTESIAN_POINT('Ctrl Pts',(1.50980486807181,1.,-0.894452006967538));
#28707=CARTESIAN_POINT('Ctrl Pts',(1.51805569591479,-1.,-0.89918504749193));
#28708=CARTESIAN_POINT('Ctrl Pts',(1.51805569591479,1.,-0.89918504749193));
#28709=CARTESIAN_POINT('Ctrl Pts',(1.52984849890434,-1.,-0.905967409640499));
#28710=CARTESIAN_POINT('Ctrl Pts',(1.52984849890434,1.,-0.905967409640499));
#28711=CARTESIAN_POINT('Ctrl Pts',(1.54440491152807,-1.,-0.91437591904658));
#28712=CARTESIAN_POINT('Ctrl Pts',(1.54440491152807,1.,-0.91437591904658));
#28713=CARTESIAN_POINT('Ctrl Pts',(1.56065988582509,-1.,-0.923832188966322));
#28714=CARTESIAN_POINT('Ctrl Pts',(1.56065988582509,1.,-0.923832188966322));
#28715=CARTESIAN_POINT('Ctrl Pts',(1.57499388385561,-1.,-0.932246680128849));
#28716=CARTESIAN_POINT('Ctrl Pts',(1.57499388385561,1.,-0.932246680128849));
#28717=CARTESIAN_POINT('Ctrl Pts',(1.58744937489796,-1.,-0.939646377909319));
#28718=CARTESIAN_POINT('Ctrl Pts',(1.58744937489796,1.,-0.939646377909319));
#28719=CARTESIAN_POINT('Ctrl Pts',(1.59810042045408,-1.,-0.946078063325796));
#28720=CARTESIAN_POINT('Ctrl Pts',(1.59810042045408,1.,-0.946078063325796));
#28721=CARTESIAN_POINT('Ctrl Pts',(1.60706069897794,-1.,-0.951613284361248));
#28722=CARTESIAN_POINT('Ctrl Pts',(1.60706069897794,1.,-0.951613284361248));
#28723=CARTESIAN_POINT('Ctrl Pts',(1.61449324337233,-1.,-0.956354422921573));
#28724=CARTESIAN_POINT('Ctrl Pts',(1.61449324337233,1.,-0.956354422921573));
#28725=CARTESIAN_POINT('Ctrl Pts',(1.62061638139929,-1.,-0.960438326099958));
#28726=CARTESIAN_POINT('Ctrl Pts',(1.62061638139929,1.,-0.960438326099958));
#28727=CARTESIAN_POINT('Ctrl Pts',(1.6257193066974,-1.,-0.964046107037821));
#28728=CARTESIAN_POINT('Ctrl Pts',(1.6257193066974,1.,-0.964046107037821));
#28729=CARTESIAN_POINT('Ctrl Pts',(1.63013849959083,-1.,-0.967387853228041));
#28730=CARTESIAN_POINT('Ctrl Pts',(1.63013849959083,1.,-0.967387853228041));
#28731=CARTESIAN_POINT('Ctrl Pts',(1.63420665729609,-1.,-0.970669715996356));
#28732=CARTESIAN_POINT('Ctrl Pts',(1.63420665729609,1.,-0.970669715996356));
#28733=CARTESIAN_POINT('Ctrl Pts',(1.63820952658157,-1.,-0.974066058287501));
#28734=CARTESIAN_POINT('Ctrl Pts',(1.63820952658157,1.,-0.974066058287501));
#28735=CARTESIAN_POINT('Ctrl Pts',(1.64233990826831,-1.,-0.977689794120297));
#28736=CARTESIAN_POINT('Ctrl Pts',(1.64233990826831,1.,-0.977689794120297));
#28737=CARTESIAN_POINT('Ctrl Pts',(1.64665139190834,-1.,-0.981562530940574));
#28738=CARTESIAN_POINT('Ctrl Pts',(1.64665139190834,1.,-0.981562530940574));
#28739=CARTESIAN_POINT('Ctrl Pts',(1.6511001661277,-1.,-0.985642622921626));
#28740=CARTESIAN_POINT('Ctrl Pts',(1.6511001661277,1.,-0.985642622921626));
#28741=CARTESIAN_POINT('Ctrl Pts',(1.65559044289746,-1.,-0.98985562785445));
#28742=CARTESIAN_POINT('Ctrl Pts',(1.65559044289746,1.,-0.98985562785445));
#28743=CARTESIAN_POINT('Ctrl Pts',(1.66001553809916,-1.,-0.994121836661116));
#28744=CARTESIAN_POINT('Ctrl Pts',(1.66001553809916,1.,-0.994121836661116));
#28745=CARTESIAN_POINT('Ctrl Pts',(1.66430758030304,-1.,-0.998389654952317));
#28746=CARTESIAN_POINT('Ctrl Pts',(1.66430758030304,1.,-0.998389654952317));
#28747=CARTESIAN_POINT('Ctrl Pts',(1.66846059277231,-1.,-1.00265091003682));
#28748=CARTESIAN_POINT('Ctrl Pts',(1.66846059277231,1.,-1.00265091003682));
#28749=CARTESIAN_POINT('Ctrl Pts',(1.67250335383248,-1.,-1.00692206696387));
#28750=CARTESIAN_POINT('Ctrl Pts',(1.67250335383248,1.,-1.00692206696387));
#28751=CARTESIAN_POINT('Ctrl Pts',(1.67648246776457,-1.,-1.01123236493507));
#28752=CARTESIAN_POINT('Ctrl Pts',(1.67648246776457,1.,-1.01123236493507));
#28753=CARTESIAN_POINT('Ctrl Pts',(1.6804428989482,-1.,-1.01561026162787));
#28754=CARTESIAN_POINT('Ctrl Pts',(1.6804428989482,1.,-1.01561026162787));
#28755=CARTESIAN_POINT('Ctrl Pts',(1.68440578021739,-1.,-1.02006795074222));
#28756=CARTESIAN_POINT('Ctrl Pts',(1.68440578021739,1.,-1.02006795074222));
#28757=CARTESIAN_POINT('Ctrl Pts',(1.68836910178475,-1.,-1.02460180535272));
#28758=CARTESIAN_POINT('Ctrl Pts',(1.68836910178475,1.,-1.02460180535272));
#28759=CARTESIAN_POINT('Ctrl Pts',(1.69231840863471,-1.,-1.02919977579155));
#28760=CARTESIAN_POINT('Ctrl Pts',(1.69231840863471,1.,-1.02919977579155));
#28761=CARTESIAN_POINT('Ctrl Pts',(1.69623414782769,-1.,-1.03384646003587));
#28762=CARTESIAN_POINT('Ctrl Pts',(1.69623414782769,1.,-1.03384646003587));
#28763=CARTESIAN_POINT('Ctrl Pts',(1.70010052930951,-1.,-1.03852922490782));
#28764=CARTESIAN_POINT('Ctrl Pts',(1.70010052930951,1.,-1.03852922490782));
#28765=CARTESIAN_POINT('Ctrl Pts',(1.70391338707969,-1.,-1.04324363334546));
#28766=CARTESIAN_POINT('Ctrl Pts',(1.70391338707969,1.,-1.04324363334546));
#28767=CARTESIAN_POINT('Ctrl Pts',(1.70767646263641,-1.,-1.0479908540499));
#28768=CARTESIAN_POINT('Ctrl Pts',(1.70767646263641,1.,-1.0479908540499));
#28769=CARTESIAN_POINT('Ctrl Pts',(1.71139783543986,-1.,-1.05277517202854));
#28770=CARTESIAN_POINT('Ctrl Pts',(1.71139783543986,1.,-1.05277517202854));
#28771=CARTESIAN_POINT('Ctrl Pts',(1.71508654427022,-1.,-1.05760163192481));
#28772=CARTESIAN_POINT('Ctrl Pts',(1.71508654427022,1.,-1.05760163192481));
#28773=CARTESIAN_POINT('Ctrl Pts',(1.71874858456908,-1.,-1.0624732468065));
#28774=CARTESIAN_POINT('Ctrl Pts',(1.71874858456908,1.,-1.0624732468065));
#28775=CARTESIAN_POINT('Ctrl Pts',(1.72238500928456,-1.,-1.06738966975463));
#28776=CARTESIAN_POINT('Ctrl Pts',(1.72238500928456,1.,-1.06738966975463));
#28777=CARTESIAN_POINT('Ctrl Pts',(1.72599406198489,-1.,-1.07234866990252));
#28778=CARTESIAN_POINT('Ctrl Pts',(1.72599406198489,1.,-1.07234866990252));
#28779=CARTESIAN_POINT('Ctrl Pts',(1.72957248977424,-1.,-1.0773470373727));
#28780=CARTESIAN_POINT('Ctrl Pts',(1.72957248977424,1.,-1.0773470373727));
#28781=CARTESIAN_POINT('Ctrl Pts',(1.73311705663407,-1.,-1.08238162784749));
#28782=CARTESIAN_POINT('Ctrl Pts',(1.73311705663407,1.,-1.08238162784749));
#28783=CARTESIAN_POINT('Ctrl Pts',(1.73662628326093,-1.,-1.08745056285429));
#28784=CARTESIAN_POINT('Ctrl Pts',(1.73662628326093,1.,-1.08745056285429));
#28785=CARTESIAN_POINT('Ctrl Pts',(1.74010053962252,-1.,-1.09255329056496));
#28786=CARTESIAN_POINT('Ctrl Pts',(1.74010053962252,1.,-1.09255329056496));
#28787=CARTESIAN_POINT('Ctrl Pts',(1.74354119236212,-1.,-1.09768999241229));
#28788=CARTESIAN_POINT('Ctrl Pts',(1.74354119236212,1.,-1.09768999241229));
#28789=CARTESIAN_POINT('Ctrl Pts',(1.74695004214924,-1.,-1.10286118991144));
#28790=CARTESIAN_POINT('Ctrl Pts',(1.74695004214924,1.,-1.10286118991144));
#28791=CARTESIAN_POINT('Ctrl Pts',(1.75032866075914,-1.,-1.10806728183003));
#28792=CARTESIAN_POINT('Ctrl Pts',(1.75032866075914,1.,-1.10806728183003));
#28793=CARTESIAN_POINT('Ctrl Pts',(1.75367772094617,-1.,-1.11330807582542));
#28794=CARTESIAN_POINT('Ctrl Pts',(1.75367772094617,1.,-1.11330807582542));
#28795=CARTESIAN_POINT('Ctrl Pts',(1.75699720772089,-1.,-1.11858293216752));
#28796=CARTESIAN_POINT('Ctrl Pts',(1.75699720772089,1.,-1.11858293216752));
#28797=CARTESIAN_POINT('Ctrl Pts',(1.76028671825084,-1.,-1.12389096855078));
#28798=CARTESIAN_POINT('Ctrl Pts',(1.76028671825084,1.,-1.12389096855078));
#28799=CARTESIAN_POINT('Ctrl Pts',(1.76354571966171,-1.,-1.12923123555076));
#28800=CARTESIAN_POINT('Ctrl Pts',(1.76354571966171,1.,-1.12923123555076));
#28801=CARTESIAN_POINT('Ctrl Pts',(1.76677384551883,-1.,-1.13460291804635));
#28802=CARTESIAN_POINT('Ctrl Pts',(1.76677384551883,1.,-1.13460291804635));
#28803=CARTESIAN_POINT('Ctrl Pts',(1.76997111386806,-1.,-1.14000548337));
#28804=CARTESIAN_POINT('Ctrl Pts',(1.76997111386806,1.,-1.14000548337));
#28805=CARTESIAN_POINT('Ctrl Pts',(1.77313777896234,-1.,-1.14543858226948));
#28806=CARTESIAN_POINT('Ctrl Pts',(1.77313777896234,1.,-1.14543858226948));
#28807=CARTESIAN_POINT('Ctrl Pts',(1.77627422557034,-1.,-1.15090197841531));
#28808=CARTESIAN_POINT('Ctrl Pts',(1.77627422557034,1.,-1.15090197841531));
#28809=CARTESIAN_POINT('Ctrl Pts',(1.77938085564261,-1.,-1.15639547194689));
#28810=CARTESIAN_POINT('Ctrl Pts',(1.77938085564261,1.,-1.15639547194689));
#28811=CARTESIAN_POINT('Ctrl Pts',(1.78245795880949,-1.,-1.16191881298458));
#28812=CARTESIAN_POINT('Ctrl Pts',(1.78245795880949,1.,-1.16191881298458));
#28813=CARTESIAN_POINT('Ctrl Pts',(1.78550566040349,-1.,-1.16747166312239));
#28814=CARTESIAN_POINT('Ctrl Pts',(1.78550566040349,1.,-1.16747166312239));
#28815=CARTESIAN_POINT('Ctrl Pts',(1.78852398877523,-1.,-1.17305363177265));
#28816=CARTESIAN_POINT('Ctrl Pts',(1.78852398877523,1.,-1.17305363177265));
#28817=CARTESIAN_POINT('Ctrl Pts',(1.79151291552646,-1.,-1.17866429440781));
#28818=CARTESIAN_POINT('Ctrl Pts',(1.79151291552646,1.,-1.17866429440781));
#28819=CARTESIAN_POINT('Ctrl Pts',(1.79447240321572,-1.,-1.18430321697471));
#28820=CARTESIAN_POINT('Ctrl Pts',(1.79447240321572,1.,-1.18430321697471));
#28821=CARTESIAN_POINT('Ctrl Pts',(1.79740245923649,-1.,-1.1899699793456));
#28822=CARTESIAN_POINT('Ctrl Pts',(1.79740245923649,1.,-1.1899699793456));
#28823=CARTESIAN_POINT('Ctrl Pts',(1.80030314370121,-1.,-1.19566418930405));
#28824=CARTESIAN_POINT('Ctrl Pts',(1.80030314370121,1.,-1.19566418930405));
#28825=CARTESIAN_POINT('Ctrl Pts',(1.8031745483882,-1.,-1.2013854893912));
#28826=CARTESIAN_POINT('Ctrl Pts',(1.8031745483882,1.,-1.2013854893912));
#28827=CARTESIAN_POINT('Ctrl Pts',(1.80601678480772,-1.,-1.20713356605519));
#28828=CARTESIAN_POINT('Ctrl Pts',(1.80601678480772,1.,-1.20713356605519));
#28829=CARTESIAN_POINT('Ctrl Pts',(1.80882996916931,-1.,-1.2129081570818));
#28830=CARTESIAN_POINT('Ctrl Pts',(1.80882996916931,1.,-1.2129081570818));
#28831=CARTESIAN_POINT('Ctrl Pts',(1.81161420806172,-1.,-1.2187090610323));
#28832=CARTESIAN_POINT('Ctrl Pts',(1.81161420806172,1.,-1.2187090610323));
#28833=CARTESIAN_POINT('Ctrl Pts',(1.81436959209778,-1.,-1.22453613304507));
#28834=CARTESIAN_POINT('Ctrl Pts',(1.81436959209778,1.,-1.22453613304507));
#28835=CARTESIAN_POINT('Ctrl Pts',(1.81655087183054,-1.,-1.22921864890975));
#28836=CARTESIAN_POINT('Ctrl Pts',(1.81655087183054,1.,-1.22921864890975));
#28837=CARTESIAN_POINT('Ctrl Pts',(1.81817389920914,-1.,-1.23274224526804));
#28838=CARTESIAN_POINT('Ctrl Pts',(1.81817389920914,1.,-1.23274224526804));
#28839=CARTESIAN_POINT('Ctrl Pts',(1.81925017193531,-1.,-1.23509651170384));
#28840=CARTESIAN_POINT('Ctrl Pts',(1.81925017193531,1.,-1.23509651170384));
#28841=CARTESIAN_POINT('Ctrl Pts',(1.81978687191668,-1.,-1.23627494547115));
#28842=CARTESIAN_POINT('Ctrl Pts',(1.81978687191668,1.,-1.23627494547115));
#28843=CARTESIAN_POINT('',(1.5055822144029,1.,-0.892032620296855));
#28844=CARTESIAN_POINT('Ctrl Pts',(1.5055822144029,1.,-0.892032620296855));
#28845=CARTESIAN_POINT('Ctrl Pts',(1.50980486807181,1.,-0.894452006967538));
#28846=CARTESIAN_POINT('Ctrl Pts',(1.51805569591479,1.,-0.89918504749193));
#28847=CARTESIAN_POINT('Ctrl Pts',(1.52984849890434,1.,-0.905967409640499));
#28848=CARTESIAN_POINT('Ctrl Pts',(1.54440491152807,1.,-0.91437591904658));
#28849=CARTESIAN_POINT('Ctrl Pts',(1.56065988582509,1.,-0.923832188966322));
#28850=CARTESIAN_POINT('Ctrl Pts',(1.57499388385561,1.,-0.932246680128849));
#28851=CARTESIAN_POINT('Ctrl Pts',(1.58744937489796,1.,-0.939646377909319));
#28852=CARTESIAN_POINT('Ctrl Pts',(1.59810042045408,1.,-0.946078063325796));
#28853=CARTESIAN_POINT('Ctrl Pts',(1.60706069897794,1.,-0.951613284361248));
#28854=CARTESIAN_POINT('Ctrl Pts',(1.61449324337233,1.,-0.956354422921573));
#28855=CARTESIAN_POINT('Ctrl Pts',(1.62061638139929,1.,-0.960438326099958));
#28856=CARTESIAN_POINT('Ctrl Pts',(1.6257193066974,1.,-0.964046107037821));
#28857=CARTESIAN_POINT('Ctrl Pts',(1.63013849959083,1.,-0.967387853228041));
#28858=CARTESIAN_POINT('Ctrl Pts',(1.63420665729609,1.,-0.970669715996356));
#28859=CARTESIAN_POINT('Ctrl Pts',(1.63820952658157,1.,-0.974066058287501));
#28860=CARTESIAN_POINT('Ctrl Pts',(1.64233990826831,1.,-0.977689794120297));
#28861=CARTESIAN_POINT('Ctrl Pts',(1.64665139190834,1.,-0.981562530940574));
#28862=CARTESIAN_POINT('Ctrl Pts',(1.6511001661277,1.,-0.985642622921626));
#28863=CARTESIAN_POINT('Ctrl Pts',(1.65559044289746,1.,-0.98985562785445));
#28864=CARTESIAN_POINT('Ctrl Pts',(1.66001553809916,1.,-0.994121836661116));
#28865=CARTESIAN_POINT('Ctrl Pts',(1.66430758030304,1.,-0.998389654952317));
#28866=CARTESIAN_POINT('Ctrl Pts',(1.66846059277231,1.,-1.00265091003682));
#28867=CARTESIAN_POINT('Ctrl Pts',(1.67250335383248,1.,-1.00692206696387));
#28868=CARTESIAN_POINT('Ctrl Pts',(1.67648246776457,1.,-1.01123236493507));
#28869=CARTESIAN_POINT('Ctrl Pts',(1.6804428989482,1.,-1.01561026162787));
#28870=CARTESIAN_POINT('Ctrl Pts',(1.68440578021739,1.,-1.02006795074222));
#28871=CARTESIAN_POINT('Ctrl Pts',(1.68836910178475,1.,-1.02460180535272));
#28872=CARTESIAN_POINT('Ctrl Pts',(1.69231840863471,1.,-1.02919977579155));
#28873=CARTESIAN_POINT('Ctrl Pts',(1.69623414782769,1.,-1.03384646003587));
#28874=CARTESIAN_POINT('Ctrl Pts',(1.70010052930951,1.,-1.03852922490782));
#28875=CARTESIAN_POINT('Ctrl Pts',(1.70391338707969,1.,-1.04324363334546));
#28876=CARTESIAN_POINT('Ctrl Pts',(1.70767646263641,1.,-1.0479908540499));
#28877=CARTESIAN_POINT('Ctrl Pts',(1.71139783543986,1.,-1.05277517202854));
#28878=CARTESIAN_POINT('Ctrl Pts',(1.71508654427022,1.,-1.05760163192481));
#28879=CARTESIAN_POINT('Ctrl Pts',(1.71874858456908,1.,-1.0624732468065));
#28880=CARTESIAN_POINT('Ctrl Pts',(1.72238500928456,1.,-1.06738966975463));
#28881=CARTESIAN_POINT('Ctrl Pts',(1.72599406198489,1.,-1.07234866990252));
#28882=CARTESIAN_POINT('Ctrl Pts',(1.72957248977424,1.,-1.0773470373727));
#28883=CARTESIAN_POINT('Ctrl Pts',(1.73311705663407,1.,-1.08238162784749));
#28884=CARTESIAN_POINT('Ctrl Pts',(1.73662628326093,1.,-1.08745056285429));
#28885=CARTESIAN_POINT('Ctrl Pts',(1.74010053962252,1.,-1.09255329056496));
#28886=CARTESIAN_POINT('Ctrl Pts',(1.74354119236212,1.,-1.09768999241229));
#28887=CARTESIAN_POINT('Ctrl Pts',(1.74695004214924,1.,-1.10286118991144));
#28888=CARTESIAN_POINT('Ctrl Pts',(1.75032866075914,1.,-1.10806728183003));
#28889=CARTESIAN_POINT('Ctrl Pts',(1.75367772094617,1.,-1.11330807582542));
#28890=CARTESIAN_POINT('Ctrl Pts',(1.75699720772089,1.,-1.11858293216752));
#28891=CARTESIAN_POINT('Ctrl Pts',(1.76028671825084,1.,-1.12389096855078));
#28892=CARTESIAN_POINT('Ctrl Pts',(1.76354571966171,1.,-1.12923123555076));
#28893=CARTESIAN_POINT('Ctrl Pts',(1.76677384551883,1.,-1.13460291804635));
#28894=CARTESIAN_POINT('Ctrl Pts',(1.76997111386806,1.,-1.14000548337));
#28895=CARTESIAN_POINT('Ctrl Pts',(1.77313777896234,1.,-1.14543858226948));
#28896=CARTESIAN_POINT('Ctrl Pts',(1.77627422557034,1.,-1.15090197841531));
#28897=CARTESIAN_POINT('Ctrl Pts',(1.77938085564261,1.,-1.15639547194689));
#28898=CARTESIAN_POINT('Ctrl Pts',(1.78245795880949,1.,-1.16191881298458));
#28899=CARTESIAN_POINT('Ctrl Pts',(1.78550566040349,1.,-1.16747166312239));
#28900=CARTESIAN_POINT('Ctrl Pts',(1.78852398877523,1.,-1.17305363177265));
#28901=CARTESIAN_POINT('Ctrl Pts',(1.79151291552646,1.,-1.17866429440781));
#28902=CARTESIAN_POINT('Ctrl Pts',(1.79447240321572,1.,-1.18430321697471));
#28903=CARTESIAN_POINT('Ctrl Pts',(1.79740245923649,1.,-1.1899699793456));
#28904=CARTESIAN_POINT('Ctrl Pts',(1.80030314370121,1.,-1.19566418930405));
#28905=CARTESIAN_POINT('Ctrl Pts',(1.8031745483882,1.,-1.2013854893912));
#28906=CARTESIAN_POINT('Ctrl Pts',(1.80601678480772,1.,-1.20713356605519));
#28907=CARTESIAN_POINT('Ctrl Pts',(1.80882996916931,1.,-1.2129081570818));
#28908=CARTESIAN_POINT('Ctrl Pts',(1.81161420806172,1.,-1.2187090610323));
#28909=CARTESIAN_POINT('Ctrl Pts',(1.81436959209778,1.,-1.22453613304507));
#28910=CARTESIAN_POINT('Ctrl Pts',(1.81655087183054,1.,-1.22921864890975));
#28911=CARTESIAN_POINT('Ctrl Pts',(1.81817389920914,1.,-1.23274224526804));
#28912=CARTESIAN_POINT('Ctrl Pts',(1.81925017193531,1.,-1.23509651170384));
#28913=CARTESIAN_POINT('Ctrl Pts',(1.81978687191668,1.,-1.23627494547115));
#28914=CARTESIAN_POINT('',(1.5055822144029,0.,-0.892032620296855));
#28915=CARTESIAN_POINT('Origin',(0.,0.,0.));
#28916=CARTESIAN_POINT('',(1.60662857109684,1.,-0.693717979106306));
#28917=CARTESIAN_POINT('Origin',(0.,1.,0.));
#28918=CARTESIAN_POINT('',(1.60662857109684,0.,-0.693717979106308));
#28919=CARTESIAN_POINT('Ctrl Pts',(2.0698113262342,-1.,-0.745574324794401));
#28920=CARTESIAN_POINT('Ctrl Pts',(2.0698113262342,1.,-0.745574324794401));
#28921=CARTESIAN_POINT('Ctrl Pts',(2.06854248895728,-1.,-0.745832791378367));
#28922=CARTESIAN_POINT('Ctrl Pts',(2.06854248895728,1.,-0.745832791378367));
#28923=CARTESIAN_POINT('Ctrl Pts',(2.06600523016815,-1.,-0.746345871544201));
#28924=CARTESIAN_POINT('Ctrl Pts',(2.06600523016815,1.,-0.746345871544201));
#28925=CARTESIAN_POINT('Ctrl Pts',(2.06220058927826,-1.,-0.74710393278792));
#28926=CARTESIAN_POINT('Ctrl Pts',(2.06220058927826,1.,-0.74710393278792));
#28927=CARTESIAN_POINT('Ctrl Pts',(2.05713023031006,-1.,-0.748091554183803));
#28928=CARTESIAN_POINT('Ctrl Pts',(2.05713023031006,1.,-0.748091554183803));
#28929=CARTESIAN_POINT('Ctrl Pts',(2.05079645592154,-1.,-0.749287468665046));
#28930=CARTESIAN_POINT('Ctrl Pts',(2.05079645592154,1.,-0.749287468665046));
#28931=CARTESIAN_POINT('Ctrl Pts',(2.04446689147979,-1.,-0.750444657875576));
#28932=CARTESIAN_POINT('Ctrl Pts',(2.04446689147979,1.,-0.750444657875576));
#28933=CARTESIAN_POINT('Ctrl Pts',(2.03814160092099,-1.,-0.751562963361115));
#28934=CARTESIAN_POINT('Ctrl Pts',(2.03814160092099,1.,-0.751562963361115));
#28935=CARTESIAN_POINT('Ctrl Pts',(2.03182068456221,-1.,-0.752642180487211));
#28936=CARTESIAN_POINT('Ctrl Pts',(2.03182068456221,1.,-0.752642180487211));
#28937=CARTESIAN_POINT('Ctrl Pts',(2.02550428623313,-1.,-0.753682061112768));
#28938=CARTESIAN_POINT('Ctrl Pts',(2.02550428623313,1.,-0.753682061112768));
#28939=CARTESIAN_POINT('Ctrl Pts',(2.01919259405809,-1.,-0.754682330722816));
#28940=CARTESIAN_POINT('Ctrl Pts',(2.01919259405809,1.,-0.754682330722816));
#28941=CARTESIAN_POINT('Ctrl Pts',(2.01288584328084,-1.,-0.755642704957865));
#28942=CARTESIAN_POINT('Ctrl Pts',(2.01288584328084,1.,-0.755642704957865));
#28943=CARTESIAN_POINT('Ctrl Pts',(2.0065843158773,-1.,-0.756562904646671));
#28944=CARTESIAN_POINT('Ctrl Pts',(2.0065843158773,1.,-0.756562904646671));
#28945=CARTESIAN_POINT('Ctrl Pts',(2.00028834739178,-1.,-0.757442676862724));
#28946=CARTESIAN_POINT('Ctrl Pts',(2.00028834739178,1.,-0.757442676862724));
#28947=CARTESIAN_POINT('Ctrl Pts',(1.99399831098817,-1.,-0.758281796766761));
#28948=CARTESIAN_POINT('Ctrl Pts',(1.99399831098817,1.,-0.758281796766761));
#28949=CARTESIAN_POINT('Ctrl Pts',(1.98771456680874,-1.,-0.759080037802488));
#28950=CARTESIAN_POINT('Ctrl Pts',(1.98771456680874,1.,-0.759080037802488));
#28951=CARTESIAN_POINT('Ctrl Pts',(1.98143741418172,-1.,-0.75983714745219));
#28952=CARTESIAN_POINT('Ctrl Pts',(1.98143741418172,1.,-0.75983714745219));
#28953=CARTESIAN_POINT('Ctrl Pts',(1.97516705321494,-1.,-0.760552825409757));
#28954=CARTESIAN_POINT('Ctrl Pts',(1.97516705321494,1.,-0.760552825409757));
#28955=CARTESIAN_POINT('Ctrl Pts',(1.96890351582499,-1.,-0.761226690483821));
#28956=CARTESIAN_POINT('Ctrl Pts',(1.96890351582499,1.,-0.761226690483821));
#28957=CARTESIAN_POINT('Ctrl Pts',(1.96264672744186,-1.,-0.761858300014424));
#28958=CARTESIAN_POINT('Ctrl Pts',(1.96264672744186,1.,-0.761858300014424));
#28959=CARTESIAN_POINT('Ctrl Pts',(1.95639665309869,-1.,-0.762447203806179));
#28960=CARTESIAN_POINT('Ctrl Pts',(1.95639665309869,1.,-0.762447203806179));
#28961=CARTESIAN_POINT('Ctrl Pts',(1.95015342590024,-1.,-0.762992990878769));
#28962=CARTESIAN_POINT('Ctrl Pts',(1.95015342590024,1.,-0.762992990878769));
#28963=CARTESIAN_POINT('Ctrl Pts',(1.9439174661764,-1.,-0.763495333538629));
#28964=CARTESIAN_POINT('Ctrl Pts',(1.9439174661764,1.,-0.763495333538629));
#28965=CARTESIAN_POINT('Ctrl Pts',(1.93768964875886,-1.,-0.763954049121459));
#28966=CARTESIAN_POINT('Ctrl Pts',(1.93768964875886,1.,-0.763954049121459));
#28967=CARTESIAN_POINT('Ctrl Pts',(1.93147105496382,-1.,-0.764369010673941));
#28968=CARTESIAN_POINT('Ctrl Pts',(1.93147105496382,1.,-0.764369010673941));
#28969=CARTESIAN_POINT('Ctrl Pts',(1.92526263537048,-1.,-0.764740025488212));
#28970=CARTESIAN_POINT('Ctrl Pts',(1.92526263537048,1.,-0.764740025488212));
#28971=CARTESIAN_POINT('Ctrl Pts',(1.91906491634196,-1.,-0.765066729667089));
#28972=CARTESIAN_POINT('Ctrl Pts',(1.91906491634196,1.,-0.765066729667089));
#28973=CARTESIAN_POINT('Ctrl Pts',(1.91287765805169,-1.,-0.765348465884722));
#28974=CARTESIAN_POINT('Ctrl Pts',(1.91287765805169,1.,-0.765348465884722));
#28975=CARTESIAN_POINT('Ctrl Pts',(1.90669961402356,-1.,-0.765584196937919));
#28976=CARTESIAN_POINT('Ctrl Pts',(1.90669961402356,1.,-0.765584196937919));
#28977=CARTESIAN_POINT('Ctrl Pts',(1.90052930393596,-1.,-0.765772772593386));
#28978=CARTESIAN_POINT('Ctrl Pts',(1.90052930393596,1.,-0.765772772593386));
#28979=CARTESIAN_POINT('Ctrl Pts',(1.89436577771388,-1.,-0.765913193856978));
#28980=CARTESIAN_POINT('Ctrl Pts',(1.89436577771388,1.,-0.765913193856978));
#28981=CARTESIAN_POINT('Ctrl Pts',(1.88820926433409,-1.,-0.766004837062091));
#28982=CARTESIAN_POINT('Ctrl Pts',(1.88820926433409,1.,-0.766004837062091));
#28983=CARTESIAN_POINT('Ctrl Pts',(1.88206215302561,-1.,-0.766047794851865));
#28984=CARTESIAN_POINT('Ctrl Pts',(1.88206215302561,1.,-0.766047794851865));
#28985=CARTESIAN_POINT('Ctrl Pts',(1.87592888967883,-1.,-0.766042837036744));
#28986=CARTESIAN_POINT('Ctrl Pts',(1.87592888967883,1.,-0.766042837036744));
#28987=CARTESIAN_POINT('Ctrl Pts',(1.86981398314341,-1.,-0.765990708546091));
#28988=CARTESIAN_POINT('Ctrl Pts',(1.86981398314341,1.,-0.765990708546091));
#28989=CARTESIAN_POINT('Ctrl Pts',(1.86372027063312,-1.,-0.765891519092547));
#28990=CARTESIAN_POINT('Ctrl Pts',(1.86372027063312,1.,-0.765891519092547));
#28991=CARTESIAN_POINT('Ctrl Pts',(1.85764741390394,-1.,-0.765744212909319));
#28992=CARTESIAN_POINT('Ctrl Pts',(1.85764741390394,1.,-0.765744212909319));
#28993=CARTESIAN_POINT('Ctrl Pts',(1.85158945130063,-1.,-0.765545710619063));
#28994=CARTESIAN_POINT('Ctrl Pts',(1.85158945130063,1.,-0.765545710619063));
#28995=CARTESIAN_POINT('Ctrl Pts',(1.84553698875924,-1.,-0.765291664862029));
#28996=CARTESIAN_POINT('Ctrl Pts',(1.84553698875924,1.,-0.765291664862029));
#28997=CARTESIAN_POINT('Ctrl Pts',(1.83948181064835,-1.,-0.764978057881738));
#28998=CARTESIAN_POINT('Ctrl Pts',(1.83948181064835,1.,-0.764978057881738));
#28999=CARTESIAN_POINT('Ctrl Pts',(1.83342077227142,-1.,-0.764602549687853));
#29000=CARTESIAN_POINT('Ctrl Pts',(1.83342077227142,1.,-0.764602549687853));
#29001=CARTESIAN_POINT('Ctrl Pts',(1.82735991200065,-1.,-0.764165902605995));
#29002=CARTESIAN_POINT('Ctrl Pts',(1.82735991200065,1.,-0.764165902605995));
#29003=CARTESIAN_POINT('Ctrl Pts',(1.82131873145266,-1.,-0.763673465462727));
#29004=CARTESIAN_POINT('Ctrl Pts',(1.82131873145266,1.,-0.763673465462727));
#29005=CARTESIAN_POINT('Ctrl Pts',(1.8153211840553,-1.,-0.763132003836634));
#29006=CARTESIAN_POINT('Ctrl Pts',(1.8153211840553,1.,-0.763132003836634));
#29007=CARTESIAN_POINT('Ctrl Pts',(1.80938551463965,-1.,-0.762546129463938));
#29008=CARTESIAN_POINT('Ctrl Pts',(1.80938551463965,1.,-0.762546129463938));
#29009=CARTESIAN_POINT('Ctrl Pts',(1.80351583877342,-1.,-0.761915336443547));
#29010=CARTESIAN_POINT('Ctrl Pts',(1.80351583877342,1.,-0.761915336443547));
#29011=CARTESIAN_POINT('Ctrl Pts',(1.79768986997783,-1.,-0.761229695230558));
#29012=CARTESIAN_POINT('Ctrl Pts',(1.79768986997783,1.,-0.761229695230558));
#29013=CARTESIAN_POINT('Ctrl Pts',(1.7918581561088,-1.,-0.760469555880749));
#29014=CARTESIAN_POINT('Ctrl Pts',(1.7918581561088,1.,-0.760469555880749));
#29015=CARTESIAN_POINT('Ctrl Pts',(1.78596964884604,-1.,-0.75961440111019));
#29016=CARTESIAN_POINT('Ctrl Pts',(1.78596964884604,1.,-0.75961440111019));
#29017=CARTESIAN_POINT('Ctrl Pts',(1.77999411220945,-1.,-0.758650626677519));
#29018=CARTESIAN_POINT('Ctrl Pts',(1.77999411220945,1.,-0.758650626677519));
#29019=CARTESIAN_POINT('Ctrl Pts',(1.77394167108292,-1.,-0.757578264077029));
#29020=CARTESIAN_POINT('Ctrl Pts',(1.77394167108292,1.,-0.757578264077029));
#29021=CARTESIAN_POINT('Ctrl Pts',(1.76789396002998,-1.,-0.75642189602781));
#29022=CARTESIAN_POINT('Ctrl Pts',(1.76789396002998,1.,-0.75642189602781));
#29023=CARTESIAN_POINT('Ctrl Pts',(1.76197817240128,-1.,-0.755220979974462));
#29024=CARTESIAN_POINT('Ctrl Pts',(1.76197817240128,1.,-0.755220979974462));
#29025=CARTESIAN_POINT('Ctrl Pts',(1.75631083600019,-1.,-0.754009254027829));
#29026=CARTESIAN_POINT('Ctrl Pts',(1.75631083600019,1.,-0.754009254027829));
#29027=CARTESIAN_POINT('Ctrl Pts',(1.75095139468794,-1.,-0.752797683531314));
#29028=CARTESIAN_POINT('Ctrl Pts',(1.75095139468794,1.,-0.752797683531314));
#29029=CARTESIAN_POINT('Ctrl Pts',(1.74585086852502,-1.,-0.751555614164483));
#29030=CARTESIAN_POINT('Ctrl Pts',(1.74585086852502,1.,-0.751555614164483));
#29031=CARTESIAN_POINT('Ctrl Pts',(1.74080458267114,-1.,-0.75019343598125));
#29032=CARTESIAN_POINT('Ctrl Pts',(1.74080458267114,1.,-0.75019343598125));
#29033=CARTESIAN_POINT('Ctrl Pts',(1.7355035168033,-1.,-0.74858246295687));
#29034=CARTESIAN_POINT('Ctrl Pts',(1.7355035168033,1.,-0.74858246295687));
#29035=CARTESIAN_POINT('Ctrl Pts',(1.72958533647714,-1.,-0.746574710097752));
#29036=CARTESIAN_POINT('Ctrl Pts',(1.72958533647714,1.,-0.746574710097752));
#29037=CARTESIAN_POINT('Ctrl Pts',(1.72268229916769,-1.,-0.744021445433094));
#29038=CARTESIAN_POINT('Ctrl Pts',(1.72268229916769,1.,-0.744021445433094));
#29039=CARTESIAN_POINT('Ctrl Pts',(1.71447789751001,-1.,-0.74079516202821));
#29040=CARTESIAN_POINT('Ctrl Pts',(1.71447789751001,1.,-0.74079516202821));
#29041=CARTESIAN_POINT('Ctrl Pts',(1.70473309004249,-1.,-0.736799665716932));
#29042=CARTESIAN_POINT('Ctrl Pts',(1.70473309004249,1.,-0.736799665716932));
#29043=CARTESIAN_POINT('Ctrl Pts',(1.69326921972915,-1.,-0.731963238685357));
#29044=CARTESIAN_POINT('Ctrl Pts',(1.69326921972915,1.,-0.731963238685357));
#29045=CARTESIAN_POINT('Ctrl Pts',(1.67996158451922,-1.,-0.726235967982445));
#29046=CARTESIAN_POINT('Ctrl Pts',(1.67996158451922,1.,-0.726235967982445));
#29047=CARTESIAN_POINT('Ctrl Pts',(1.66472880551777,-1.,-0.71958543378795));
#29048=CARTESIAN_POINT('Ctrl Pts',(1.66472880551777,1.,-0.71958543378795));
#29049=CARTESIAN_POINT('Ctrl Pts',(1.64752408828442,-1.,-0.711993139340448));
#29050=CARTESIAN_POINT('Ctrl Pts',(1.64752408828442,1.,-0.711993139340448));
#29051=CARTESIAN_POINT('Ctrl Pts',(1.6321654166204,-1.,-0.705159151977294));
#29052=CARTESIAN_POINT('Ctrl Pts',(1.6321654166204,1.,-0.705159151977294));
#29053=CARTESIAN_POINT('Ctrl Pts',(1.61974673471117,-1.,-0.699605146398837));
#29054=CARTESIAN_POINT('Ctrl Pts',(1.61974673471117,1.,-0.699605146398837));
#29055=CARTESIAN_POINT('Ctrl Pts',(1.61106790957619,-1.,-0.69571209787897));
#29056=CARTESIAN_POINT('Ctrl Pts',(1.61106790957619,1.,-0.69571209787897));
#29057=CARTESIAN_POINT('Ctrl Pts',(1.60662857109684,-1.,-0.693717979106306));
#29058=CARTESIAN_POINT('Ctrl Pts',(1.60662857109684,1.,-0.693717979106306));
#29059=CARTESIAN_POINT('',(2.0698113262342,1.,-0.745574324794401));
#29060=CARTESIAN_POINT('Ctrl Pts',(2.0698113262342,1.,-0.745574324794401));
#29061=CARTESIAN_POINT('Ctrl Pts',(2.06854248895728,1.,-0.745832791378367));
#29062=CARTESIAN_POINT('Ctrl Pts',(2.06600523016815,1.,-0.746345871544201));
#29063=CARTESIAN_POINT('Ctrl Pts',(2.06220058927826,1.,-0.74710393278792));
#29064=CARTESIAN_POINT('Ctrl Pts',(2.05713023031006,1.,-0.748091554183803));
#29065=CARTESIAN_POINT('Ctrl Pts',(2.05079645592154,1.,-0.749287468665046));
#29066=CARTESIAN_POINT('Ctrl Pts',(2.04446689147979,1.,-0.750444657875576));
#29067=CARTESIAN_POINT('Ctrl Pts',(2.03814160092099,1.,-0.751562963361115));
#29068=CARTESIAN_POINT('Ctrl Pts',(2.03182068456221,1.,-0.752642180487211));
#29069=CARTESIAN_POINT('Ctrl Pts',(2.02550428623313,1.,-0.753682061112768));
#29070=CARTESIAN_POINT('Ctrl Pts',(2.01919259405809,1.,-0.754682330722816));
#29071=CARTESIAN_POINT('Ctrl Pts',(2.01288584328084,1.,-0.755642704957865));
#29072=CARTESIAN_POINT('Ctrl Pts',(2.0065843158773,1.,-0.756562904646671));
#29073=CARTESIAN_POINT('Ctrl Pts',(2.00028834739178,1.,-0.757442676862724));
#29074=CARTESIAN_POINT('Ctrl Pts',(1.99399831098817,1.,-0.758281796766761));
#29075=CARTESIAN_POINT('Ctrl Pts',(1.98771456680874,1.,-0.759080037802488));
#29076=CARTESIAN_POINT('Ctrl Pts',(1.98143741418172,1.,-0.75983714745219));
#29077=CARTESIAN_POINT('Ctrl Pts',(1.97516705321494,1.,-0.760552825409757));
#29078=CARTESIAN_POINT('Ctrl Pts',(1.96890351582499,1.,-0.761226690483821));
#29079=CARTESIAN_POINT('Ctrl Pts',(1.96264672744186,1.,-0.761858300014424));
#29080=CARTESIAN_POINT('Ctrl Pts',(1.95639665309869,1.,-0.762447203806179));
#29081=CARTESIAN_POINT('Ctrl Pts',(1.95015342590024,1.,-0.762992990878769));
#29082=CARTESIAN_POINT('Ctrl Pts',(1.9439174661764,1.,-0.763495333538629));
#29083=CARTESIAN_POINT('Ctrl Pts',(1.93768964875886,1.,-0.763954049121459));
#29084=CARTESIAN_POINT('Ctrl Pts',(1.93147105496382,1.,-0.764369010673941));
#29085=CARTESIAN_POINT('Ctrl Pts',(1.92526263537048,1.,-0.764740025488212));
#29086=CARTESIAN_POINT('Ctrl Pts',(1.91906491634196,1.,-0.765066729667089));
#29087=CARTESIAN_POINT('Ctrl Pts',(1.91287765805169,1.,-0.765348465884722));
#29088=CARTESIAN_POINT('Ctrl Pts',(1.90669961402356,1.,-0.765584196937919));
#29089=CARTESIAN_POINT('Ctrl Pts',(1.90052930393596,1.,-0.765772772593386));
#29090=CARTESIAN_POINT('Ctrl Pts',(1.89436577771388,1.,-0.765913193856978));
#29091=CARTESIAN_POINT('Ctrl Pts',(1.88820926433409,1.,-0.766004837062091));
#29092=CARTESIAN_POINT('Ctrl Pts',(1.88206215302561,1.,-0.766047794851865));
#29093=CARTESIAN_POINT('Ctrl Pts',(1.87592888967883,1.,-0.766042837036744));
#29094=CARTESIAN_POINT('Ctrl Pts',(1.86981398314341,1.,-0.765990708546091));
#29095=CARTESIAN_POINT('Ctrl Pts',(1.86372027063312,1.,-0.765891519092547));
#29096=CARTESIAN_POINT('Ctrl Pts',(1.85764741390394,1.,-0.765744212909319));
#29097=CARTESIAN_POINT('Ctrl Pts',(1.85158945130063,1.,-0.765545710619063));
#29098=CARTESIAN_POINT('Ctrl Pts',(1.84553698875924,1.,-0.765291664862029));
#29099=CARTESIAN_POINT('Ctrl Pts',(1.83948181064835,1.,-0.764978057881738));
#29100=CARTESIAN_POINT('Ctrl Pts',(1.83342077227142,1.,-0.764602549687853));
#29101=CARTESIAN_POINT('Ctrl Pts',(1.82735991200065,1.,-0.764165902605995));
#29102=CARTESIAN_POINT('Ctrl Pts',(1.82131873145266,1.,-0.763673465462727));
#29103=CARTESIAN_POINT('Ctrl Pts',(1.8153211840553,1.,-0.763132003836634));
#29104=CARTESIAN_POINT('Ctrl Pts',(1.80938551463965,1.,-0.762546129463938));
#29105=CARTESIAN_POINT('Ctrl Pts',(1.80351583877342,1.,-0.761915336443547));
#29106=CARTESIAN_POINT('Ctrl Pts',(1.79768986997783,1.,-0.761229695230558));
#29107=CARTESIAN_POINT('Ctrl Pts',(1.7918581561088,1.,-0.760469555880749));
#29108=CARTESIAN_POINT('Ctrl Pts',(1.78596964884604,1.,-0.75961440111019));
#29109=CARTESIAN_POINT('Ctrl Pts',(1.77999411220945,1.,-0.758650626677519));
#29110=CARTESIAN_POINT('Ctrl Pts',(1.77394167108292,1.,-0.757578264077029));
#29111=CARTESIAN_POINT('Ctrl Pts',(1.76789396002998,1.,-0.75642189602781));
#29112=CARTESIAN_POINT('Ctrl Pts',(1.76197817240128,1.,-0.755220979974462));
#29113=CARTESIAN_POINT('Ctrl Pts',(1.75631083600019,1.,-0.754009254027829));
#29114=CARTESIAN_POINT('Ctrl Pts',(1.75095139468794,1.,-0.752797683531314));
#29115=CARTESIAN_POINT('Ctrl Pts',(1.74585086852502,1.,-0.751555614164483));
#29116=CARTESIAN_POINT('Ctrl Pts',(1.74080458267114,1.,-0.75019343598125));
#29117=CARTESIAN_POINT('Ctrl Pts',(1.7355035168033,1.,-0.74858246295687));
#29118=CARTESIAN_POINT('Ctrl Pts',(1.72958533647714,1.,-0.746574710097752));
#29119=CARTESIAN_POINT('Ctrl Pts',(1.72268229916769,1.,-0.744021445433094));
#29120=CARTESIAN_POINT('Ctrl Pts',(1.71447789751001,1.,-0.74079516202821));
#29121=CARTESIAN_POINT('Ctrl Pts',(1.70473309004249,1.,-0.736799665716932));
#29122=CARTESIAN_POINT('Ctrl Pts',(1.69326921972915,1.,-0.731963238685357));
#29123=CARTESIAN_POINT('Ctrl Pts',(1.67996158451922,1.,-0.726235967982445));
#29124=CARTESIAN_POINT('Ctrl Pts',(1.66472880551777,1.,-0.71958543378795));
#29125=CARTESIAN_POINT('Ctrl Pts',(1.64752408828442,1.,-0.711993139340448));
#29126=CARTESIAN_POINT('Ctrl Pts',(1.6321654166204,1.,-0.705159151977294));
#29127=CARTESIAN_POINT('Ctrl Pts',(1.61974673471117,1.,-0.699605146398837));
#29128=CARTESIAN_POINT('Ctrl Pts',(1.61106790957619,1.,-0.69571209787897));
#29129=CARTESIAN_POINT('Ctrl Pts',(1.60662857109684,1.,-0.693717979106306));
#29130=CARTESIAN_POINT('',(2.0698113262342,0.,-0.745574324794401));
#29131=CARTESIAN_POINT('Origin',(2.11275013067528,0.,-0.61342227326009));
#29132=CARTESIAN_POINT('',(2.11275013067528,1.,-0.61342227326009));
#29133=CARTESIAN_POINT('',(2.0698113262342,1.,-0.745574324794401));
#29134=CARTESIAN_POINT('',(2.11275013067528,0.,-0.61342227326009));
#29135=CARTESIAN_POINT('Ctrl Pts',(1.7075470150345,-1.,-0.383122945602004));
#29136=CARTESIAN_POINT('Ctrl Pts',(1.7075470150345,1.,-0.383122945602004));
#29137=CARTESIAN_POINT('Ctrl Pts',(1.71231062891958,-1.,-0.384119047315542));
#29138=CARTESIAN_POINT('Ctrl Pts',(1.71231062891958,1.,-0.384119047315542));
#29139=CARTESIAN_POINT('Ctrl Pts',(1.72162022246158,-1.,-0.38607079032701));
#29140=CARTESIAN_POINT('Ctrl Pts',(1.72162022246158,1.,-0.38607079032701));
#29141=CARTESIAN_POINT('Ctrl Pts',(1.7349317097561,-1.,-0.388877023509192));
#29142=CARTESIAN_POINT('Ctrl Pts',(1.7349317097561,1.,-0.388877023509192));
#29143=CARTESIAN_POINT('Ctrl Pts',(1.75137405313962,-1.,-0.392375812294307));
#29144=CARTESIAN_POINT('Ctrl Pts',(1.75137405313962,1.,-0.392375812294307));
#29145=CARTESIAN_POINT('Ctrl Pts',(1.7697556004756,-1.,-0.39634619612042));
#29146=CARTESIAN_POINT('Ctrl Pts',(1.7697556004756,1.,-0.39634619612042));
#29147=CARTESIAN_POINT('Ctrl Pts',(1.78598826347533,-1.,-0.399919403783081));
#29148=CARTESIAN_POINT('Ctrl Pts',(1.78598826347533,1.,-0.399919403783081));
#29149=CARTESIAN_POINT('Ctrl Pts',(1.80012077176221,-1.,-0.403107976170441));
#29150=CARTESIAN_POINT('Ctrl Pts',(1.80012077176221,1.,-0.403107976170441));
#29151=CARTESIAN_POINT('Ctrl Pts',(1.81223801813988,-1.,-0.405933518411838));
#29152=CARTESIAN_POINT('Ctrl Pts',(1.81223801813988,1.,-0.405933518411838));
#29153=CARTESIAN_POINT('Ctrl Pts',(1.8224702267854,-1.,-0.408428948108534));
#29154=CARTESIAN_POINT('Ctrl Pts',(1.8224702267854,1.,-0.408428948108534));
#29155=CARTESIAN_POINT('Ctrl Pts',(1.83100408895216,-1.,-0.410641256301675));
#29156=CARTESIAN_POINT('Ctrl Pts',(1.83100408895216,1.,-0.410641256301675));
#29157=CARTESIAN_POINT('Ctrl Pts',(1.83808953475839,-1.,-0.412633125322162));
#29158=CARTESIAN_POINT('Ctrl Pts',(1.83808953475839,1.,-0.412633125322162));
#29159=CARTESIAN_POINT('Ctrl Pts',(1.8440575707371,-1.,-0.41448743825434));
#29160=CARTESIAN_POINT('Ctrl Pts',(1.8440575707371,1.,-0.41448743825434));
#29161=CARTESIAN_POINT('Ctrl Pts',(1.84929312929882,-1.,-0.416300022038864));
#29162=CARTESIAN_POINT('Ctrl Pts',(1.84929312929882,1.,-0.416300022038864));
#29163=CARTESIAN_POINT('Ctrl Pts',(1.85417632856234,-1.,-0.418164129143534));
#29164=CARTESIAN_POINT('Ctrl Pts',(1.85417632856234,1.,-0.418164129143534));
#29165=CARTESIAN_POINT('Ctrl Pts',(1.85903281096686,-1.,-0.42015728797562));
#29166=CARTESIAN_POINT('Ctrl Pts',(1.85903281096686,1.,-0.42015728797562));
#29167=CARTESIAN_POINT('Ctrl Pts',(1.86408083334028,-1.,-0.422327307418275));
#29168=CARTESIAN_POINT('Ctrl Pts',(1.86408083334028,1.,-0.422327307418275));
#29169=CARTESIAN_POINT('Ctrl Pts',(1.86937803944323,-1.,-0.424678177291359));
#29170=CARTESIAN_POINT('Ctrl Pts',(1.86937803944323,1.,-0.424678177291359));
#29171=CARTESIAN_POINT('Ctrl Pts',(1.87486989291484,-1.,-0.427183828519102));
#29172=CARTESIAN_POINT('Ctrl Pts',(1.87486989291484,1.,-0.427183828519102));
#29173=CARTESIAN_POINT('Ctrl Pts',(1.88044229001832,-1.,-0.429803062482345));
#29174=CARTESIAN_POINT('Ctrl Pts',(1.88044229001832,1.,-0.429803062482345));
#29175=CARTESIAN_POINT('Ctrl Pts',(1.88596913666793,-1.,-0.432493038548748));
#29176=CARTESIAN_POINT('Ctrl Pts',(1.88596913666793,1.,-0.432493038548748));
#29177=CARTESIAN_POINT('Ctrl Pts',(1.89136993975504,-1.,-0.435225660963383));
#29178=CARTESIAN_POINT('Ctrl Pts',(1.89136993975504,1.,-0.435225660963383));
#29179=CARTESIAN_POINT('Ctrl Pts',(1.89663648956466,-1.,-0.437995003948244));
#29180=CARTESIAN_POINT('Ctrl Pts',(1.89663648956466,1.,-0.437995003948244));
#29181=CARTESIAN_POINT('Ctrl Pts',(1.90180124389086,-1.,-0.440807833704038));
#29182=CARTESIAN_POINT('Ctrl Pts',(1.90180124389086,1.,-0.440807833704038));
#29183=CARTESIAN_POINT('Ctrl Pts',(1.90691756144898,-1.,-0.443677556849151));
#29184=CARTESIAN_POINT('Ctrl Pts',(1.90691756144898,1.,-0.443677556849151));
#29185=CARTESIAN_POINT('Ctrl Pts',(1.9120369998112,-1.,-0.446617343485711));
#29186=CARTESIAN_POINT('Ctrl Pts',(1.9120369998112,1.,-0.446617343485711));
#29187=CARTESIAN_POINT('Ctrl Pts',(1.91718342555755,-1.,-0.449632260106662));
#29188=CARTESIAN_POINT('Ctrl Pts',(1.91718342555755,1.,-0.449632260106662));
#29189=CARTESIAN_POINT('Ctrl Pts',(1.92235380648502,-1.,-0.452719478359433));
#29190=CARTESIAN_POINT('Ctrl Pts',(1.92235380648502,1.,-0.452719478359433));
#29191=CARTESIAN_POINT('Ctrl Pts',(1.92753067150476,-1.,-0.455872005174371));
#29192=CARTESIAN_POINT('Ctrl Pts',(1.92753067150476,1.,-0.455872005174371));
#29193=CARTESIAN_POINT('Ctrl Pts',(1.93269066517934,-1.,-0.459081234547926));
#29194=CARTESIAN_POINT('Ctrl Pts',(1.93269066517934,1.,-0.459081234547926));
#29195=CARTESIAN_POINT('Ctrl Pts',(1.93781486640821,-1.,-0.462340031009057));
#29196=CARTESIAN_POINT('Ctrl Pts',(1.93781486640821,1.,-0.462340031009057));
#29197=CARTESIAN_POINT('Ctrl Pts',(1.9428979419619,-1.,-0.46564546202603));
#29198=CARTESIAN_POINT('Ctrl Pts',(1.9428979419619,1.,-0.46564546202603));
#29199=CARTESIAN_POINT('Ctrl Pts',(1.94794381136514,-1.,-0.468997482913135));
#29200=CARTESIAN_POINT('Ctrl Pts',(1.94794381136514,1.,-0.468997482913135));
#29201=CARTESIAN_POINT('Ctrl Pts',(1.95296148278133,-1.,-0.472397672264072));
#29202=CARTESIAN_POINT('Ctrl Pts',(1.95296148278133,1.,-0.472397672264072));
#29203=CARTESIAN_POINT('Ctrl Pts',(1.95796111148177,-1.,-0.475848034683176));
#29204=CARTESIAN_POINT('Ctrl Pts',(1.95796111148177,1.,-0.475848034683176));
#29205=CARTESIAN_POINT('Ctrl Pts',(1.96294933055943,-1.,-0.479349583074855));
#29206=CARTESIAN_POINT('Ctrl Pts',(1.96294933055943,1.,-0.479349583074855));
#29207=CARTESIAN_POINT('Ctrl Pts',(1.96792703422362,-1.,-0.482901662120691));
#29208=CARTESIAN_POINT('Ctrl Pts',(1.96792703422362,1.,-0.482901662120691));
#29209=CARTESIAN_POINT('Ctrl Pts',(1.97289186263272,-1.,-0.486502692907659));
#29210=CARTESIAN_POINT('Ctrl Pts',(1.97289186263272,1.,-0.486502692907659));
#29211=CARTESIAN_POINT('Ctrl Pts',(1.97783973019229,-1.,-0.490150627860953));
#29212=CARTESIAN_POINT('Ctrl Pts',(1.97783973019229,1.,-0.490150627860953));
#29213=CARTESIAN_POINT('Ctrl Pts',(1.98276658761821,-1.,-0.493843476541495));
#29214=CARTESIAN_POINT('Ctrl Pts',(1.98276658761821,1.,-0.493843476541495));
#29215=CARTESIAN_POINT('Ctrl Pts',(1.98767044752932,-1.,-0.497579909545574));
#29216=CARTESIAN_POINT('Ctrl Pts',(1.98767044752932,1.,-0.497579909545574));
#29217=CARTESIAN_POINT('Ctrl Pts',(1.99255149126155,-1.,-0.501359287727146));
#29218=CARTESIAN_POINT('Ctrl Pts',(1.99255149126155,1.,-0.501359287727146));
#29219=CARTESIAN_POINT('Ctrl Pts',(1.99741107463572,-1.,-0.505181361323026));
#29220=CARTESIAN_POINT('Ctrl Pts',(1.99741107463572,1.,-0.505181361323026));
#29221=CARTESIAN_POINT('Ctrl Pts',(2.00225107134734,-1.,-0.509046069886157));
#29222=CARTESIAN_POINT('Ctrl Pts',(2.00225107134734,1.,-0.509046069886157));
#29223=CARTESIAN_POINT('Ctrl Pts',(2.00707309946949,-1.,-0.512953306961793));
#29224=CARTESIAN_POINT('Ctrl Pts',(2.00707309946949,1.,-0.512953306961793));
#29225=CARTESIAN_POINT('Ctrl Pts',(2.01187773939242,-1.,-0.516902681728687));
#29226=CARTESIAN_POINT('Ctrl Pts',(2.01187773939242,1.,-0.516902681728687));
#29227=CARTESIAN_POINT('Ctrl Pts',(2.01666477917286,-1.,-0.520893590399371));
#29228=CARTESIAN_POINT('Ctrl Pts',(2.01666477917286,1.,-0.520893590399371));
#29229=CARTESIAN_POINT('Ctrl Pts',(2.02143356304698,-1.,-0.524925318333476));
#29230=CARTESIAN_POINT('Ctrl Pts',(2.02143356304698,1.,-0.524925318333476));
#29231=CARTESIAN_POINT('Ctrl Pts',(2.0261832908329,-1.,-0.528997127241914));
#29232=CARTESIAN_POINT('Ctrl Pts',(2.0261832908329,1.,-0.528997127241914));
#29233=CARTESIAN_POINT('Ctrl Pts',(2.03091336214426,-1.,-0.533108355132977));
#29234=CARTESIAN_POINT('Ctrl Pts',(2.03091336214426,1.,-0.533108355132977));
#29235=CARTESIAN_POINT('Ctrl Pts',(2.03562362954037,-1.,-0.537258489833262));
#29236=CARTESIAN_POINT('Ctrl Pts',(2.03562362954037,1.,-0.537258489833262));
#29237=CARTESIAN_POINT('Ctrl Pts',(2.04031422690527,-1.,-0.541447120615659));
#29238=CARTESIAN_POINT('Ctrl Pts',(2.04031422690527,1.,-0.541447120615659));
#29239=CARTESIAN_POINT('Ctrl Pts',(2.04498544714588,-1.,-0.54567390381743));
#29240=CARTESIAN_POINT('Ctrl Pts',(2.04498544714588,1.,-0.54567390381743));
#29241=CARTESIAN_POINT('Ctrl Pts',(2.04963761077958,-1.,-0.549938525150295));
#29242=CARTESIAN_POINT('Ctrl Pts',(2.04963761077958,1.,-0.549938525150295));
#29243=CARTESIAN_POINT('Ctrl Pts',(2.05427091604413,-1.,-0.554240657463906));
#29244=CARTESIAN_POINT('Ctrl Pts',(2.05427091604413,1.,-0.554240657463906));
#29245=CARTESIAN_POINT('Ctrl Pts',(2.05888537756462,-1.,-0.558579940185152));
#29246=CARTESIAN_POINT('Ctrl Pts',(2.05888537756462,1.,-0.558579940185152));
#29247=CARTESIAN_POINT('Ctrl Pts',(2.06348090160589,-1.,-0.562955993082262));
#29248=CARTESIAN_POINT('Ctrl Pts',(2.06348090160589,1.,-0.562955993082262));
#29249=CARTESIAN_POINT('Ctrl Pts',(2.06805732997334,-1.,-0.567368421181087));
#29250=CARTESIAN_POINT('Ctrl Pts',(2.06805732997334,1.,-0.567368421181087));
#29251=CARTESIAN_POINT('Ctrl Pts',(2.07261449292824,-1.,-0.571816823242603));
#29252=CARTESIAN_POINT('Ctrl Pts',(2.07261449292824,1.,-0.571816823242603));
#29253=CARTESIAN_POINT('Ctrl Pts',(2.07715226767559,-1.,-0.576300797416845));
#29254=CARTESIAN_POINT('Ctrl Pts',(2.07715226767559,1.,-0.576300797416845));
#29255=CARTESIAN_POINT('Ctrl Pts',(2.08167059018418,-1.,-0.580819952108064));
#29256=CARTESIAN_POINT('Ctrl Pts',(2.08167059018418,1.,-0.580819952108064));
#29257=CARTESIAN_POINT('Ctrl Pts',(2.08616943727951,-1.,-0.585373918991617));
#29258=CARTESIAN_POINT('Ctrl Pts',(2.08616943727951,1.,-0.585373918991617));
#29259=CARTESIAN_POINT('Ctrl Pts',(2.09064881812129,-1.,-0.589962365403406));
#29260=CARTESIAN_POINT('Ctrl Pts',(2.09064881812129,1.,-0.589962365403406));
#29261=CARTESIAN_POINT('Ctrl Pts',(2.0951087622027,-1.,-0.594585006052162));
#29262=CARTESIAN_POINT('Ctrl Pts',(2.0951087622027,1.,-0.594585006052162));
#29263=CARTESIAN_POINT('Ctrl Pts',(2.0995493086477,-1.,-0.599241616420534));
#29264=CARTESIAN_POINT('Ctrl Pts',(2.0995493086477,1.,-0.599241616420534));
#29265=CARTESIAN_POINT('Ctrl Pts',(2.10397049886949,-1.,-0.60393203073603));
#29266=CARTESIAN_POINT('Ctrl Pts',(2.10397049886949,1.,-0.60393203073603));
#29267=CARTESIAN_POINT('Ctrl Pts',(2.1074919961518,-1.,-0.607711315454876));
#29268=CARTESIAN_POINT('Ctrl Pts',(2.1074919961518,1.,-0.607711315454876));
#29269=CARTESIAN_POINT('Ctrl Pts',(2.11012443807238,-1.,-0.610560911689899));
#29270=CARTESIAN_POINT('Ctrl Pts',(2.11012443807238,1.,-0.610560911689899));
#29271=CARTESIAN_POINT('Ctrl Pts',(2.11187554259986,-1.,-0.6124673655618));
#29272=CARTESIAN_POINT('Ctrl Pts',(2.11187554259986,1.,-0.6124673655618));
#29273=CARTESIAN_POINT('Ctrl Pts',(2.11275013067528,-1.,-0.61342227326009));
#29274=CARTESIAN_POINT('Ctrl Pts',(2.11275013067528,1.,-0.61342227326009));
#29275=CARTESIAN_POINT('',(1.7075470150345,1.,-0.383122945602004));
#29276=CARTESIAN_POINT('Ctrl Pts',(1.7075470150345,1.,-0.383122945602004));
#29277=CARTESIAN_POINT('Ctrl Pts',(1.71231062891958,1.,-0.384119047315542));
#29278=CARTESIAN_POINT('Ctrl Pts',(1.72162022246158,1.,-0.38607079032701));
#29279=CARTESIAN_POINT('Ctrl Pts',(1.7349317097561,1.,-0.388877023509192));
#29280=CARTESIAN_POINT('Ctrl Pts',(1.75137405313962,1.,-0.392375812294307));
#29281=CARTESIAN_POINT('Ctrl Pts',(1.7697556004756,1.,-0.39634619612042));
#29282=CARTESIAN_POINT('Ctrl Pts',(1.78598826347533,1.,-0.399919403783081));
#29283=CARTESIAN_POINT('Ctrl Pts',(1.80012077176221,1.,-0.403107976170441));
#29284=CARTESIAN_POINT('Ctrl Pts',(1.81223801813988,1.,-0.405933518411838));
#29285=CARTESIAN_POINT('Ctrl Pts',(1.8224702267854,1.,-0.408428948108534));
#29286=CARTESIAN_POINT('Ctrl Pts',(1.83100408895216,1.,-0.410641256301675));
#29287=CARTESIAN_POINT('Ctrl Pts',(1.83808953475839,1.,-0.412633125322162));
#29288=CARTESIAN_POINT('Ctrl Pts',(1.8440575707371,1.,-0.41448743825434));
#29289=CARTESIAN_POINT('Ctrl Pts',(1.84929312929882,1.,-0.416300022038864));
#29290=CARTESIAN_POINT('Ctrl Pts',(1.85417632856234,1.,-0.418164129143534));
#29291=CARTESIAN_POINT('Ctrl Pts',(1.85903281096686,1.,-0.42015728797562));
#29292=CARTESIAN_POINT('Ctrl Pts',(1.86408083334028,1.,-0.422327307418275));
#29293=CARTESIAN_POINT('Ctrl Pts',(1.86937803944323,1.,-0.424678177291359));
#29294=CARTESIAN_POINT('Ctrl Pts',(1.87486989291484,1.,-0.427183828519102));
#29295=CARTESIAN_POINT('Ctrl Pts',(1.88044229001832,1.,-0.429803062482345));
#29296=CARTESIAN_POINT('Ctrl Pts',(1.88596913666793,1.,-0.432493038548748));
#29297=CARTESIAN_POINT('Ctrl Pts',(1.89136993975504,1.,-0.435225660963383));
#29298=CARTESIAN_POINT('Ctrl Pts',(1.89663648956466,1.,-0.437995003948244));
#29299=CARTESIAN_POINT('Ctrl Pts',(1.90180124389086,1.,-0.440807833704038));
#29300=CARTESIAN_POINT('Ctrl Pts',(1.90691756144898,1.,-0.443677556849151));
#29301=CARTESIAN_POINT('Ctrl Pts',(1.9120369998112,1.,-0.446617343485711));
#29302=CARTESIAN_POINT('Ctrl Pts',(1.91718342555755,1.,-0.449632260106662));
#29303=CARTESIAN_POINT('Ctrl Pts',(1.92235380648502,1.,-0.452719478359433));
#29304=CARTESIAN_POINT('Ctrl Pts',(1.92753067150476,1.,-0.455872005174371));
#29305=CARTESIAN_POINT('Ctrl Pts',(1.93269066517934,1.,-0.459081234547926));
#29306=CARTESIAN_POINT('Ctrl Pts',(1.93781486640821,1.,-0.462340031009057));
#29307=CARTESIAN_POINT('Ctrl Pts',(1.9428979419619,1.,-0.46564546202603));
#29308=CARTESIAN_POINT('Ctrl Pts',(1.94794381136514,1.,-0.468997482913135));
#29309=CARTESIAN_POINT('Ctrl Pts',(1.95296148278133,1.,-0.472397672264072));
#29310=CARTESIAN_POINT('Ctrl Pts',(1.95796111148177,1.,-0.475848034683176));
#29311=CARTESIAN_POINT('Ctrl Pts',(1.96294933055943,1.,-0.479349583074855));
#29312=CARTESIAN_POINT('Ctrl Pts',(1.96792703422362,1.,-0.482901662120691));
#29313=CARTESIAN_POINT('Ctrl Pts',(1.97289186263272,1.,-0.486502692907659));
#29314=CARTESIAN_POINT('Ctrl Pts',(1.97783973019229,1.,-0.490150627860953));
#29315=CARTESIAN_POINT('Ctrl Pts',(1.98276658761821,1.,-0.493843476541495));
#29316=CARTESIAN_POINT('Ctrl Pts',(1.98767044752932,1.,-0.497579909545574));
#29317=CARTESIAN_POINT('Ctrl Pts',(1.99255149126155,1.,-0.501359287727146));
#29318=CARTESIAN_POINT('Ctrl Pts',(1.99741107463572,1.,-0.505181361323026));
#29319=CARTESIAN_POINT('Ctrl Pts',(2.00225107134734,1.,-0.509046069886157));
#29320=CARTESIAN_POINT('Ctrl Pts',(2.00707309946949,1.,-0.512953306961793));
#29321=CARTESIAN_POINT('Ctrl Pts',(2.01187773939242,1.,-0.516902681728687));
#29322=CARTESIAN_POINT('Ctrl Pts',(2.01666477917286,1.,-0.520893590399371));
#29323=CARTESIAN_POINT('Ctrl Pts',(2.02143356304698,1.,-0.524925318333476));
#29324=CARTESIAN_POINT('Ctrl Pts',(2.0261832908329,1.,-0.528997127241914));
#29325=CARTESIAN_POINT('Ctrl Pts',(2.03091336214426,1.,-0.533108355132977));
#29326=CARTESIAN_POINT('Ctrl Pts',(2.03562362954037,1.,-0.537258489833262));
#29327=CARTESIAN_POINT('Ctrl Pts',(2.04031422690527,1.,-0.541447120615659));
#29328=CARTESIAN_POINT('Ctrl Pts',(2.04498544714588,1.,-0.54567390381743));
#29329=CARTESIAN_POINT('Ctrl Pts',(2.04963761077958,1.,-0.549938525150295));
#29330=CARTESIAN_POINT('Ctrl Pts',(2.05427091604413,1.,-0.554240657463906));
#29331=CARTESIAN_POINT('Ctrl Pts',(2.05888537756462,1.,-0.558579940185152));
#29332=CARTESIAN_POINT('Ctrl Pts',(2.06348090160589,1.,-0.562955993082262));
#29333=CARTESIAN_POINT('Ctrl Pts',(2.06805732997334,1.,-0.567368421181087));
#29334=CARTESIAN_POINT('Ctrl Pts',(2.07261449292824,1.,-0.571816823242603));
#29335=CARTESIAN_POINT('Ctrl Pts',(2.07715226767559,1.,-0.576300797416845));
#29336=CARTESIAN_POINT('Ctrl Pts',(2.08167059018418,1.,-0.580819952108064));
#29337=CARTESIAN_POINT('Ctrl Pts',(2.08616943727951,1.,-0.585373918991617));
#29338=CARTESIAN_POINT('Ctrl Pts',(2.09064881812129,1.,-0.589962365403406));
#29339=CARTESIAN_POINT('Ctrl Pts',(2.0951087622027,1.,-0.594585006052162));
#29340=CARTESIAN_POINT('Ctrl Pts',(2.0995493086477,1.,-0.599241616420534));
#29341=CARTESIAN_POINT('Ctrl Pts',(2.10397049886949,1.,-0.60393203073603));
#29342=CARTESIAN_POINT('Ctrl Pts',(2.1074919961518,1.,-0.607711315454876));
#29343=CARTESIAN_POINT('Ctrl Pts',(2.11012443807238,1.,-0.610560911689899));
#29344=CARTESIAN_POINT('Ctrl Pts',(2.11187554259986,1.,-0.6124673655618));
#29345=CARTESIAN_POINT('Ctrl Pts',(2.11275013067528,1.,-0.61342227326009));
#29346=CARTESIAN_POINT('',(1.7075470150345,0.,-0.383122945602001));
#29347=CARTESIAN_POINT('Origin',(0.,0.,0.));
#29348=CARTESIAN_POINT('',(1.74236521665491,1.,-0.163289472382896));
#29349=CARTESIAN_POINT('Origin',(0.,1.,0.));
#29350=CARTESIAN_POINT('',(1.74236521665491,0.,-0.163289472382896));
#29351=CARTESIAN_POINT('Ctrl Pts',(2.19890268624765,-1.,-0.0694764450219582));
#29352=CARTESIAN_POINT('Ctrl Pts',(2.19890268624765,1.,-0.0694764450219582));
#29353=CARTESIAN_POINT('Ctrl Pts',(2.19777582085423,-1.,-0.0701143536325491));
#29354=CARTESIAN_POINT('Ctrl Pts',(2.19777582085423,1.,-0.0701143536325491));
#29355=CARTESIAN_POINT('Ctrl Pts',(2.19552129484002,-1.,-0.0713863779526155));
#29356=CARTESIAN_POINT('Ctrl Pts',(2.19552129484002,1.,-0.0713863779526155));
#29357=CARTESIAN_POINT('Ctrl Pts',(2.19213712013662,-1.,-0.0732830357306726));
#29358=CARTESIAN_POINT('Ctrl Pts',(2.19213712013662,1.,-0.0732830357306726));
#29359=CARTESIAN_POINT('Ctrl Pts',(2.1876201139953,-1.,-0.0757891465836149));
#29360=CARTESIAN_POINT('Ctrl Pts',(2.1876201139953,1.,-0.0757891465836149));
#29361=CARTESIAN_POINT('Ctrl Pts',(2.18196589448887,-1.,-0.0788837727685244));
#29362=CARTESIAN_POINT('Ctrl Pts',(2.18196589448887,1.,-0.0788837727685244));
#29363=CARTESIAN_POINT('Ctrl Pts',(2.176303712113,-1.,-0.0819402680872767));
#29364=CARTESIAN_POINT('Ctrl Pts',(2.176303712113,1.,-0.0819402680872767));
#29365=CARTESIAN_POINT('Ctrl Pts',(2.17063357870952,-1.,-0.0849584620835374));
#29366=CARTESIAN_POINT('Ctrl Pts',(2.17063357870952,1.,-0.0849584620835374));
#29367=CARTESIAN_POINT('Ctrl Pts',(2.16495552645014,-1.,-0.0879381291386924));
#29368=CARTESIAN_POINT('Ctrl Pts',(2.16495552645014,1.,-0.0879381291386924));
#29369=CARTESIAN_POINT('Ctrl Pts',(2.15926961544516,-1.,-0.0908789888107267));
#29370=CARTESIAN_POINT('Ctrl Pts',(2.15926961544516,1.,-0.0908789888107267));
#29371=CARTESIAN_POINT('Ctrl Pts',(2.1535759397817,-1.,-0.0937807218867645));
#29372=CARTESIAN_POINT('Ctrl Pts',(2.1535759397817,1.,-0.0937807218867645));
#29373=CARTESIAN_POINT('Ctrl Pts',(2.14787463531795,-1.,-0.096642985230546));
#29374=CARTESIAN_POINT('Ctrl Pts',(2.14787463531795,1.,-0.096642985230546));
#29375=CARTESIAN_POINT('Ctrl Pts',(2.14216588396025,-1.,-0.0994654261990917));
#29376=CARTESIAN_POINT('Ctrl Pts',(2.14216588396025,1.,-0.0994654261990917));
#29377=CARTESIAN_POINT('Ctrl Pts',(2.13644992667165,-1.,-0.102247700556101));
#29378=CARTESIAN_POINT('Ctrl Pts',(2.13644992667165,1.,-0.102247700556101));
#29379=CARTESIAN_POINT('Ctrl Pts',(2.13072704887293,-1.,-0.10498947915274));
#29380=CARTESIAN_POINT('Ctrl Pts',(2.13072704887293,1.,-0.10498947915274));
#29381=CARTESIAN_POINT('Ctrl Pts',(2.12499752307,-1.,-0.10769043523109));
#29382=CARTESIAN_POINT('Ctrl Pts',(2.12499752307,1.,-0.10769043523109));
#29383=CARTESIAN_POINT('Ctrl Pts',(2.11926155590865,-1.,-0.110350236135025));
#29384=CARTESIAN_POINT('Ctrl Pts',(2.11926155590865,1.,-0.110350236135025));
#29385=CARTESIAN_POINT('Ctrl Pts',(2.11351924490306,-1.,-0.112968534419737));
#29386=CARTESIAN_POINT('Ctrl Pts',(2.11351924490306,1.,-0.112968534419737));
#29387=CARTESIAN_POINT('Ctrl Pts',(2.10777050261309,-1.,-0.115544957687927));
#29388=CARTESIAN_POINT('Ctrl Pts',(2.10777050261309,1.,-0.115544957687927));
#29389=CARTESIAN_POINT('Ctrl Pts',(2.102015121329,-1.,-0.118079107988356));
#29390=CARTESIAN_POINT('Ctrl Pts',(2.102015121329,1.,-0.118079107988356));
#29391=CARTESIAN_POINT('Ctrl Pts',(2.0962529286773,-1.,-0.120570567965122));
#29392=CARTESIAN_POINT('Ctrl Pts',(2.0962529286773,1.,-0.120570567965122));
#29393=CARTESIAN_POINT('Ctrl Pts',(2.09048392424825,-1.,-0.123018905621083));
#29394=CARTESIAN_POINT('Ctrl Pts',(2.09048392424825,1.,-0.123018905621083));
#29395=CARTESIAN_POINT('Ctrl Pts',(2.08470840653643,-1.,-0.125423679412062));
#29396=CARTESIAN_POINT('Ctrl Pts',(2.08470840653643,1.,-0.125423679412062));
#29397=CARTESIAN_POINT('Ctrl Pts',(2.07892715110987,-1.,-0.12778444527612));
#29398=CARTESIAN_POINT('Ctrl Pts',(2.07892715110987,1.,-0.12778444527612));
#29399=CARTESIAN_POINT('Ctrl Pts',(2.07314114713063,-1.,-0.130100748328404));
#29400=CARTESIAN_POINT('Ctrl Pts',(2.07314114713063,1.,-0.130100748328404));
#29401=CARTESIAN_POINT('Ctrl Pts',(2.06735123910326,-1.,-0.132372111547711));
#29402=CARTESIAN_POINT('Ctrl Pts',(2.06735123910326,1.,-0.132372111547711));
#29403=CARTESIAN_POINT('Ctrl Pts',(2.06155781517842,-1.,-0.134598026192106));
#29404=CARTESIAN_POINT('Ctrl Pts',(2.06155781517842,1.,-0.134598026192106));
#29405=CARTESIAN_POINT('Ctrl Pts',(2.05576044414264,-1.,-0.136777941218044));
#29406=CARTESIAN_POINT('Ctrl Pts',(2.05576044414264,1.,-0.136777941218044));
#29407=CARTESIAN_POINT('Ctrl Pts',(2.04995762001328,-1.,-0.138911255368966));
#29408=CARTESIAN_POINT('Ctrl Pts',(2.04995762001328,1.,-0.138911255368966));
#29409=CARTESIAN_POINT('Ctrl Pts',(2.04414757947916,-1.,-0.140997332152546));
#29410=CARTESIAN_POINT('Ctrl Pts',(2.04414757947916,1.,-0.140997332152546));
#29411=CARTESIAN_POINT('Ctrl Pts',(2.03832911025912,-1.,-0.143035515058209));
#29412=CARTESIAN_POINT('Ctrl Pts',(2.03832911025912,1.,-0.143035515058209));
#29413=CARTESIAN_POINT('Ctrl Pts',(2.03250223739942,-1.,-0.145025140186058));
#29414=CARTESIAN_POINT('Ctrl Pts',(2.03250223739942,1.,-0.145025140186058));
#29415=CARTESIAN_POINT('Ctrl Pts',(2.02666926182017,-1.,-0.146965557332583));
#29416=CARTESIAN_POINT('Ctrl Pts',(2.02666926182017,1.,-0.146965557332583));
#29417=CARTESIAN_POINT('Ctrl Pts',(2.02083464969894,-1.,-0.148856124775337));
#29418=CARTESIAN_POINT('Ctrl Pts',(2.02083464969894,1.,-0.148856124775337));
#29419=CARTESIAN_POINT('Ctrl Pts',(2.01500291940238,-1.,-0.150696157673078));
#29420=CARTESIAN_POINT('Ctrl Pts',(2.01500291940238,1.,-0.150696157673078));
#29421=CARTESIAN_POINT('Ctrl Pts',(2.00917680318424,-1.,-0.15248488362145));
#29422=CARTESIAN_POINT('Ctrl Pts',(2.00917680318424,1.,-0.15248488362145));
#29423=CARTESIAN_POINT('Ctrl Pts',(2.00335565310543,-1.,-0.154221403049722));
#29424=CARTESIAN_POINT('Ctrl Pts',(2.00335565310543,1.,-0.154221403049722));
#29425=CARTESIAN_POINT('Ctrl Pts',(1.99753284771497,-1.,-0.155904629548784));
#29426=CARTESIAN_POINT('Ctrl Pts',(1.99753284771497,1.,-0.155904629548784));
#29427=CARTESIAN_POINT('Ctrl Pts',(1.99169810931908,-1.,-0.157533331459227));
#29428=CARTESIAN_POINT('Ctrl Pts',(1.99169810931908,1.,-0.157533331459227));
#29429=CARTESIAN_POINT('Ctrl Pts',(1.98584238283292,-1.,-0.159106226437299));
#29430=CARTESIAN_POINT('Ctrl Pts',(1.98584238283292,1.,-0.159106226437299));
#29431=CARTESIAN_POINT('Ctrl Pts',(1.97996195437559,-1.,-0.160622060784611));
#29432=CARTESIAN_POINT('Ctrl Pts',(1.97996195437559,1.,-0.160622060784611));
#29433=CARTESIAN_POINT('Ctrl Pts',(1.97406280235188,-1.,-0.162079693556289));
#29434=CARTESIAN_POINT('Ctrl Pts',(1.97406280235188,1.,-0.162079693556289));
#29435=CARTESIAN_POINT('Ctrl Pts',(1.96816512677967,-1.,-0.163478185457734));
#29436=CARTESIAN_POINT('Ctrl Pts',(1.96816512677967,1.,-0.163478185457734));
#29437=CARTESIAN_POINT('Ctrl Pts',(1.96229379940136,-1.,-0.164816568920269));
#29438=CARTESIAN_POINT('Ctrl Pts',(1.96229379940136,1.,-0.164816568920269));
#29439=CARTESIAN_POINT('Ctrl Pts',(1.9564675971873,-1.,-0.166093592002813));
#29440=CARTESIAN_POINT('Ctrl Pts',(1.9564675971873,1.,-0.166093592002813));
#29441=CARTESIAN_POINT('Ctrl Pts',(1.95069027794294,-1.,-0.167307501784476));
#29442=CARTESIAN_POINT('Ctrl Pts',(1.95069027794294,1.,-0.167307501784476));
#29443=CARTESIAN_POINT('Ctrl Pts',(1.94493757756931,-1.,-0.168455741607556));
#29444=CARTESIAN_POINT('Ctrl Pts',(1.94493757756931,1.,-0.168455741607556));
#29445=CARTESIAN_POINT('Ctrl Pts',(1.93915639211581,-1.,-0.169534904817491));
#29446=CARTESIAN_POINT('Ctrl Pts',(1.93915639211581,1.,-0.169534904817491));
#29447=CARTESIAN_POINT('Ctrl Pts',(1.93329183155539,-1.,-0.170541253116202));
#29448=CARTESIAN_POINT('Ctrl Pts',(1.93329183155539,1.,-0.170541253116202));
#29449=CARTESIAN_POINT('Ctrl Pts',(1.92731093582036,-1.,-0.171471191532988));
#29450=CARTESIAN_POINT('Ctrl Pts',(1.92731093582036,1.,-0.171471191532988));
#29451=CARTESIAN_POINT('Ctrl Pts',(1.9212233439798,-1.,-0.172321621259514));
#29452=CARTESIAN_POINT('Ctrl Pts',(1.9212233439798,1.,-0.172321621259514));
#29453=CARTESIAN_POINT('Ctrl Pts',(1.91511429159527,-1.,-0.173090695383496));
#29454=CARTESIAN_POINT('Ctrl Pts',(1.91511429159527,1.,-0.173090695383496));
#29455=CARTESIAN_POINT('Ctrl Pts',(1.90911693975267,-1.,-0.173776635257817));
#29456=CARTESIAN_POINT('Ctrl Pts',(1.90911693975267,1.,-0.173776635257817));
#29457=CARTESIAN_POINT('Ctrl Pts',(1.90335253862834,-1.,-0.174375518661085));
#29458=CARTESIAN_POINT('Ctrl Pts',(1.90335253862834,1.,-0.174375518661085));
#29459=CARTESIAN_POINT('Ctrl Pts',(1.89788101117132,-1.,-0.174879405091263));
#29460=CARTESIAN_POINT('Ctrl Pts',(1.89788101117132,1.,-0.174879405091263));
#29461=CARTESIAN_POINT('Ctrl Pts',(1.892646301985,-1.,-0.175274276190844));
#29462=CARTESIAN_POINT('Ctrl Pts',(1.892646301985,1.,-0.175274276190844));
#29463=CARTESIAN_POINT('Ctrl Pts',(1.88742606273259,-1.,-0.175538155840648));
#29464=CARTESIAN_POINT('Ctrl Pts',(1.88742606273259,1.,-0.175538155840648));
#29465=CARTESIAN_POINT('Ctrl Pts',(1.88188663145367,-1.,-0.175644148889699));
#29466=CARTESIAN_POINT('Ctrl Pts',(1.88188663145367,1.,-0.175644148889699));
#29467=CARTESIAN_POINT('Ctrl Pts',(1.87563767773588,-1.,-0.175563480746485));
#29468=CARTESIAN_POINT('Ctrl Pts',(1.87563767773588,1.,-0.175563480746485));
#29469=CARTESIAN_POINT('Ctrl Pts',(1.86828349694799,-1.,-0.175268337590758));
#29470=CARTESIAN_POINT('Ctrl Pts',(1.86828349694799,1.,-0.175268337590758));
#29471=CARTESIAN_POINT('Ctrl Pts',(1.85948367088837,-1.,-0.17473525927603));
#29472=CARTESIAN_POINT('Ctrl Pts',(1.85948367088837,1.,-0.17473525927603));
#29473=CARTESIAN_POINT('Ctrl Pts',(1.8489811319852,-1.,-0.173946627587732));
#29474=CARTESIAN_POINT('Ctrl Pts',(1.8489811319852,1.,-0.173946627587732));
#29475=CARTESIAN_POINT('Ctrl Pts',(1.83658380527692,-1.,-0.1728894428919));
#29476=CARTESIAN_POINT('Ctrl Pts',(1.83658380527692,1.,-0.1728894428919));
#29477=CARTESIAN_POINT('Ctrl Pts',(1.82215766811545,-1.,-0.171554770204119));
#29478=CARTESIAN_POINT('Ctrl Pts',(1.82215766811545,1.,-0.171554770204119));
#29479=CARTESIAN_POINT('Ctrl Pts',(1.80561530629706,-1.,-0.169936923904608));
#29480=CARTESIAN_POINT('Ctrl Pts',(1.80561530629706,1.,-0.169936923904608));
#29481=CARTESIAN_POINT('Ctrl Pts',(1.7869064998507,-1.,-0.168032772805197));
#29482=CARTESIAN_POINT('Ctrl Pts',(1.7869064998507,1.,-0.168032772805197));
#29483=CARTESIAN_POINT('Ctrl Pts',(1.77018771684844,-1.,-0.1662793551464));
#29484=CARTESIAN_POINT('Ctrl Pts',(1.77018771684844,1.,-0.1662793551464));
#29485=CARTESIAN_POINT('Ctrl Pts',(1.75666056638427,-1.,-0.164834765707159));
#29486=CARTESIAN_POINT('Ctrl Pts',(1.75666056638427,1.,-0.164834765707159));
#29487=CARTESIAN_POINT('Ctrl Pts',(1.7472034950333,-1.,-0.163814161002002));
#29488=CARTESIAN_POINT('Ctrl Pts',(1.7472034950333,1.,-0.163814161002002));
#29489=CARTESIAN_POINT('Ctrl Pts',(1.74236521665491,-1.,-0.163289472382896));
#29490=CARTESIAN_POINT('Ctrl Pts',(1.74236521665491,1.,-0.163289472382896));
#29491=CARTESIAN_POINT('',(2.19890268624765,1.,-0.0694764450219582));
#29492=CARTESIAN_POINT('Ctrl Pts',(2.19890268624765,1.,-0.0694764450219582));
#29493=CARTESIAN_POINT('Ctrl Pts',(2.19777582085423,1.,-0.0701143536325491));
#29494=CARTESIAN_POINT('Ctrl Pts',(2.19552129484002,1.,-0.0713863779526155));
#29495=CARTESIAN_POINT('Ctrl Pts',(2.19213712013662,1.,-0.0732830357306726));
#29496=CARTESIAN_POINT('Ctrl Pts',(2.1876201139953,1.,-0.0757891465836149));
#29497=CARTESIAN_POINT('Ctrl Pts',(2.18196589448887,1.,-0.0788837727685244));
#29498=CARTESIAN_POINT('Ctrl Pts',(2.176303712113,1.,-0.0819402680872767));
#29499=CARTESIAN_POINT('Ctrl Pts',(2.17063357870952,1.,-0.0849584620835374));
#29500=CARTESIAN_POINT('Ctrl Pts',(2.16495552645014,1.,-0.0879381291386924));
#29501=CARTESIAN_POINT('Ctrl Pts',(2.15926961544516,1.,-0.0908789888107267));
#29502=CARTESIAN_POINT('Ctrl Pts',(2.1535759397817,1.,-0.0937807218867645));
#29503=CARTESIAN_POINT('Ctrl Pts',(2.14787463531795,1.,-0.096642985230546));
#29504=CARTESIAN_POINT('Ctrl Pts',(2.14216588396025,1.,-0.0994654261990917));
#29505=CARTESIAN_POINT('Ctrl Pts',(2.13644992667165,1.,-0.102247700556101));
#29506=CARTESIAN_POINT('Ctrl Pts',(2.13072704887293,1.,-0.10498947915274));
#29507=CARTESIAN_POINT('Ctrl Pts',(2.12499752307,1.,-0.10769043523109));
#29508=CARTESIAN_POINT('Ctrl Pts',(2.11926155590865,1.,-0.110350236135025));
#29509=CARTESIAN_POINT('Ctrl Pts',(2.11351924490306,1.,-0.112968534419737));
#29510=CARTESIAN_POINT('Ctrl Pts',(2.10777050261309,1.,-0.115544957687927));
#29511=CARTESIAN_POINT('Ctrl Pts',(2.102015121329,1.,-0.118079107988356));
#29512=CARTESIAN_POINT('Ctrl Pts',(2.0962529286773,1.,-0.120570567965122));
#29513=CARTESIAN_POINT('Ctrl Pts',(2.09048392424825,1.,-0.123018905621083));
#29514=CARTESIAN_POINT('Ctrl Pts',(2.08470840653643,1.,-0.125423679412062));
#29515=CARTESIAN_POINT('Ctrl Pts',(2.07892715110987,1.,-0.12778444527612));
#29516=CARTESIAN_POINT('Ctrl Pts',(2.07314114713063,1.,-0.130100748328404));
#29517=CARTESIAN_POINT('Ctrl Pts',(2.06735123910326,1.,-0.132372111547711));
#29518=CARTESIAN_POINT('Ctrl Pts',(2.06155781517842,1.,-0.134598026192106));
#29519=CARTESIAN_POINT('Ctrl Pts',(2.05576044414264,1.,-0.136777941218044));
#29520=CARTESIAN_POINT('Ctrl Pts',(2.04995762001328,1.,-0.138911255368966));
#29521=CARTESIAN_POINT('Ctrl Pts',(2.04414757947916,1.,-0.140997332152546));
#29522=CARTESIAN_POINT('Ctrl Pts',(2.03832911025912,1.,-0.143035515058209));
#29523=CARTESIAN_POINT('Ctrl Pts',(2.03250223739942,1.,-0.145025140186058));
#29524=CARTESIAN_POINT('Ctrl Pts',(2.02666926182017,1.,-0.146965557332583));
#29525=CARTESIAN_POINT('Ctrl Pts',(2.02083464969894,1.,-0.148856124775337));
#29526=CARTESIAN_POINT('Ctrl Pts',(2.01500291940238,1.,-0.150696157673078));
#29527=CARTESIAN_POINT('Ctrl Pts',(2.00917680318424,1.,-0.15248488362145));
#29528=CARTESIAN_POINT('Ctrl Pts',(2.00335565310543,1.,-0.154221403049722));
#29529=CARTESIAN_POINT('Ctrl Pts',(1.99753284771497,1.,-0.155904629548784));
#29530=CARTESIAN_POINT('Ctrl Pts',(1.99169810931908,1.,-0.157533331459227));
#29531=CARTESIAN_POINT('Ctrl Pts',(1.98584238283292,1.,-0.159106226437299));
#29532=CARTESIAN_POINT('Ctrl Pts',(1.97996195437559,1.,-0.160622060784611));
#29533=CARTESIAN_POINT('Ctrl Pts',(1.97406280235188,1.,-0.162079693556289));
#29534=CARTESIAN_POINT('Ctrl Pts',(1.96816512677967,1.,-0.163478185457734));
#29535=CARTESIAN_POINT('Ctrl Pts',(1.96229379940136,1.,-0.164816568920269));
#29536=CARTESIAN_POINT('Ctrl Pts',(1.9564675971873,1.,-0.166093592002813));
#29537=CARTESIAN_POINT('Ctrl Pts',(1.95069027794294,1.,-0.167307501784476));
#29538=CARTESIAN_POINT('Ctrl Pts',(1.94493757756931,1.,-0.168455741607556));
#29539=CARTESIAN_POINT('Ctrl Pts',(1.93915639211581,1.,-0.169534904817491));
#29540=CARTESIAN_POINT('Ctrl Pts',(1.93329183155539,1.,-0.170541253116202));
#29541=CARTESIAN_POINT('Ctrl Pts',(1.92731093582036,1.,-0.171471191532988));
#29542=CARTESIAN_POINT('Ctrl Pts',(1.9212233439798,1.,-0.172321621259514));
#29543=CARTESIAN_POINT('Ctrl Pts',(1.91511429159527,1.,-0.173090695383496));
#29544=CARTESIAN_POINT('Ctrl Pts',(1.90911693975267,1.,-0.173776635257817));
#29545=CARTESIAN_POINT('Ctrl Pts',(1.90335253862834,1.,-0.174375518661085));
#29546=CARTESIAN_POINT('Ctrl Pts',(1.89788101117132,1.,-0.174879405091263));
#29547=CARTESIAN_POINT('Ctrl Pts',(1.892646301985,1.,-0.175274276190844));
#29548=CARTESIAN_POINT('Ctrl Pts',(1.88742606273259,1.,-0.175538155840648));
#29549=CARTESIAN_POINT('Ctrl Pts',(1.88188663145367,1.,-0.175644148889699));
#29550=CARTESIAN_POINT('Ctrl Pts',(1.87563767773588,1.,-0.175563480746485));
#29551=CARTESIAN_POINT('Ctrl Pts',(1.86828349694799,1.,-0.175268337590758));
#29552=CARTESIAN_POINT('Ctrl Pts',(1.85948367088837,1.,-0.17473525927603));
#29553=CARTESIAN_POINT('Ctrl Pts',(1.8489811319852,1.,-0.173946627587732));
#29554=CARTESIAN_POINT('Ctrl Pts',(1.83658380527692,1.,-0.1728894428919));
#29555=CARTESIAN_POINT('Ctrl Pts',(1.82215766811545,1.,-0.171554770204119));
#29556=CARTESIAN_POINT('Ctrl Pts',(1.80561530629706,1.,-0.169936923904608));
#29557=CARTESIAN_POINT('Ctrl Pts',(1.7869064998507,1.,-0.168032772805197));
#29558=CARTESIAN_POINT('Ctrl Pts',(1.77018771684844,1.,-0.1662793551464));
#29559=CARTESIAN_POINT('Ctrl Pts',(1.75666056638427,1.,-0.164834765707159));
#29560=CARTESIAN_POINT('Ctrl Pts',(1.7472034950333,1.,-0.163814161002002));
#29561=CARTESIAN_POINT('Ctrl Pts',(1.74236521665491,1.,-0.163289472382896));
#29562=CARTESIAN_POINT('',(2.19890268624765,0.,-0.0694764450219582));
#29563=CARTESIAN_POINT('Origin',(2.19890268624765,0.,0.0694764450219582));
#29564=CARTESIAN_POINT('',(2.19890268624765,1.,0.0694764450219582));
#29565=CARTESIAN_POINT('',(2.19890268624765,1.,-0.0694764450219582));
#29566=CARTESIAN_POINT('',(2.19890268624765,0.,0.0694764450219582));
#29567=CARTESIAN_POINT('Ctrl Pts',(1.74236521665491,-1.,0.163289472382896));
#29568=CARTESIAN_POINT('Ctrl Pts',(1.74236521665491,1.,0.163289472382896));
#29569=CARTESIAN_POINT('Ctrl Pts',(1.74720349503904,-1.,0.163814161002474));
#29570=CARTESIAN_POINT('Ctrl Pts',(1.74720349503904,1.,0.163814161002474));
#29571=CARTESIAN_POINT('Ctrl Pts',(1.75666056640041,-1.,0.164834765708484));
#29572=CARTESIAN_POINT('Ctrl Pts',(1.75666056640041,1.,0.164834765708484));
#29573=CARTESIAN_POINT('Ctrl Pts',(1.77018771687692,-1.,0.166279355148738));
#29574=CARTESIAN_POINT('Ctrl Pts',(1.77018771687692,1.,0.166279355148738));
#29575=CARTESIAN_POINT('Ctrl Pts',(1.78690649988931,-1.,0.16803277280837));
#29576=CARTESIAN_POINT('Ctrl Pts',(1.78690649988931,1.,0.16803277280837));
#29577=CARTESIAN_POINT('Ctrl Pts',(1.80561530633924,-1.,0.169936923908078));
#29578=CARTESIAN_POINT('Ctrl Pts',(1.80561530633924,1.,0.169936923908078));
#29579=CARTESIAN_POINT('Ctrl Pts',(1.82215766815414,-1.,0.171554770207306));
#29580=CARTESIAN_POINT('Ctrl Pts',(1.82215766815414,1.,0.171554770207306));
#29581=CARTESIAN_POINT('Ctrl Pts',(1.83658380530747,-1.,0.17288944289442));
#29582=CARTESIAN_POINT('Ctrl Pts',(1.83658380530747,1.,0.17288944289442));
#29583=CARTESIAN_POINT('Ctrl Pts',(1.84898113200543,-1.,0.173946627589401));
#29584=CARTESIAN_POINT('Ctrl Pts',(1.84898113200543,1.,0.173946627589401));
#29585=CARTESIAN_POINT('Ctrl Pts',(1.85948367089838,-1.,0.174735259276856));
#29586=CARTESIAN_POINT('Ctrl Pts',(1.85948367089838,1.,0.174735259276856));
#29587=CARTESIAN_POINT('Ctrl Pts',(1.86828349694972,-1.,0.1752683375909));
#29588=CARTESIAN_POINT('Ctrl Pts',(1.86828349694972,1.,0.1752683375909));
#29589=CARTESIAN_POINT('Ctrl Pts',(1.87563767773249,-1.,0.175563480746205));
#29590=CARTESIAN_POINT('Ctrl Pts',(1.87563767773249,1.,0.175563480746205));
#29591=CARTESIAN_POINT('Ctrl Pts',(1.88188663144846,-1.,0.175644148889271));
#29592=CARTESIAN_POINT('Ctrl Pts',(1.88188663144846,1.,0.175644148889271));
#29593=CARTESIAN_POINT('Ctrl Pts',(1.88742606272818,-1.,0.175538155840286));
#29594=CARTESIAN_POINT('Ctrl Pts',(1.88742606272818,1.,0.175538155840286));
#29595=CARTESIAN_POINT('Ctrl Pts',(1.89264630198279,-1.,0.175274276190664));
#29596=CARTESIAN_POINT('Ctrl Pts',(1.89264630198279,1.,0.175274276190664));
#29597=CARTESIAN_POINT('Ctrl Pts',(1.89788101117148,-1.,0.174879405091277));
#29598=CARTESIAN_POINT('Ctrl Pts',(1.89788101117148,1.,0.174879405091277));
#29599=CARTESIAN_POINT('Ctrl Pts',(1.90335253863003,-1.,0.174375518661222));
#29600=CARTESIAN_POINT('Ctrl Pts',(1.90335253863003,1.,0.174375518661222));
#29601=CARTESIAN_POINT('Ctrl Pts',(1.90911693975475,-1.,0.173776635257983));
#29602=CARTESIAN_POINT('Ctrl Pts',(1.90911693975475,1.,0.173776635257983));
#29603=CARTESIAN_POINT('Ctrl Pts',(1.91511429159681,-1.,0.173090695383619));
#29604=CARTESIAN_POINT('Ctrl Pts',(1.91511429159681,1.,0.173090695383619));
#29605=CARTESIAN_POINT('Ctrl Pts',(1.92122334398034,-1.,0.172321621259556));
#29606=CARTESIAN_POINT('Ctrl Pts',(1.92122334398034,1.,0.172321621259556));
#29607=CARTESIAN_POINT('Ctrl Pts',(1.92731093582,-1.,0.17147119153296));
#29608=CARTESIAN_POINT('Ctrl Pts',(1.92731093582,1.,0.17147119153296));
#29609=CARTESIAN_POINT('Ctrl Pts',(1.93329183155455,-1.,0.170541253116136));
#29610=CARTESIAN_POINT('Ctrl Pts',(1.93329183155455,1.,0.170541253116136));
#29611=CARTESIAN_POINT('Ctrl Pts',(1.93915639211497,-1.,0.169534904817425));
#29612=CARTESIAN_POINT('Ctrl Pts',(1.93915639211497,1.,0.169534904817425));
#29613=CARTESIAN_POINT('Ctrl Pts',(1.94493757756879,-1.,0.168455741607515));
#29614=CARTESIAN_POINT('Ctrl Pts',(1.94493757756879,1.,0.168455741607515));
#29615=CARTESIAN_POINT('Ctrl Pts',(1.95069027794286,-1.,0.167307501784469));
#29616=CARTESIAN_POINT('Ctrl Pts',(1.95069027794286,1.,0.167307501784469));
#29617=CARTESIAN_POINT('Ctrl Pts',(1.95646759718755,-1.,0.166093592002832));
#29618=CARTESIAN_POINT('Ctrl Pts',(1.95646759718755,1.,0.166093592002832));
#29619=CARTESIAN_POINT('Ctrl Pts',(1.96229379940174,-1.,0.1648165689203));
#29620=CARTESIAN_POINT('Ctrl Pts',(1.96229379940174,1.,0.1648165689203));
#29621=CARTESIAN_POINT('Ctrl Pts',(1.96816512678,-1.,0.16347818545776));
#29622=CARTESIAN_POINT('Ctrl Pts',(1.96816512678,1.,0.16347818545776));
#29623=CARTESIAN_POINT('Ctrl Pts',(1.97406280235204,-1.,0.162079693556302));
#29624=CARTESIAN_POINT('Ctrl Pts',(1.97406280235204,1.,0.162079693556302));
#29625=CARTESIAN_POINT('Ctrl Pts',(1.97996195437557,-1.,0.16062206078461));
#29626=CARTESIAN_POINT('Ctrl Pts',(1.97996195437557,1.,0.16062206078461));
#29627=CARTESIAN_POINT('Ctrl Pts',(1.98584238283279,-1.,0.159106226437288));
#29628=CARTESIAN_POINT('Ctrl Pts',(1.98584238283279,1.,0.159106226437288));
#29629=CARTESIAN_POINT('Ctrl Pts',(1.99169810931893,-1.,0.157533331459215));
#29630=CARTESIAN_POINT('Ctrl Pts',(1.99169810931893,1.,0.157533331459215));
#29631=CARTESIAN_POINT('Ctrl Pts',(1.99753284771487,-1.,0.155904629548774));
#29632=CARTESIAN_POINT('Ctrl Pts',(1.99753284771487,1.,0.155904629548774));
#29633=CARTESIAN_POINT('Ctrl Pts',(2.00335565310539,-1.,0.154221403049719));
#29634=CARTESIAN_POINT('Ctrl Pts',(2.00335565310539,1.,0.154221403049719));
#29635=CARTESIAN_POINT('Ctrl Pts',(2.00917680318426,-1.,0.152484883621452));
#29636=CARTESIAN_POINT('Ctrl Pts',(2.00917680318426,1.,0.152484883621452));
#29637=CARTESIAN_POINT('Ctrl Pts',(2.01500291940243,-1.,0.150696157673084));
#29638=CARTESIAN_POINT('Ctrl Pts',(2.01500291940243,1.,0.150696157673084));
#29639=CARTESIAN_POINT('Ctrl Pts',(2.02083464969897,-1.,0.148856124775342));
#29640=CARTESIAN_POINT('Ctrl Pts',(2.02083464969897,1.,0.148856124775342));
#29641=CARTESIAN_POINT('Ctrl Pts',(2.02666926182017,-1.,0.146965557332586));
#29642=CARTESIAN_POINT('Ctrl Pts',(2.02666926182017,1.,0.146965557332586));
#29643=CARTESIAN_POINT('Ctrl Pts',(2.03250223739941,-1.,0.145025140186058));
#29644=CARTESIAN_POINT('Ctrl Pts',(2.03250223739941,1.,0.145025140186058));
#29645=CARTESIAN_POINT('Ctrl Pts',(2.03832911025913,-1.,0.143035515058208));
#29646=CARTESIAN_POINT('Ctrl Pts',(2.03832911025913,1.,0.143035515058208));
#29647=CARTESIAN_POINT('Ctrl Pts',(2.04414757947919,-1.,0.140997332152545));
#29648=CARTESIAN_POINT('Ctrl Pts',(2.04414757947919,1.,0.140997332152545));
#29649=CARTESIAN_POINT('Ctrl Pts',(2.04995762001333,-1.,0.138911255368966));
#29650=CARTESIAN_POINT('Ctrl Pts',(2.04995762001333,1.,0.138911255368966));
#29651=CARTESIAN_POINT('Ctrl Pts',(2.0557604441427,-1.,0.136777941218044));
#29652=CARTESIAN_POINT('Ctrl Pts',(2.0557604441427,1.,0.136777941218044));
#29653=CARTESIAN_POINT('Ctrl Pts',(2.06155781517844,-1.,0.134598026192107));
#29654=CARTESIAN_POINT('Ctrl Pts',(2.06155781517844,1.,0.134598026192107));
#29655=CARTESIAN_POINT('Ctrl Pts',(2.06735123910319,-1.,0.132372111547709));
#29656=CARTESIAN_POINT('Ctrl Pts',(2.06735123910319,1.,0.132372111547709));
#29657=CARTESIAN_POINT('Ctrl Pts',(2.07314114713047,-1.,0.1301007483284));
#29658=CARTESIAN_POINT('Ctrl Pts',(2.07314114713047,1.,0.1301007483284));
#29659=CARTESIAN_POINT('Ctrl Pts',(2.07892715110967,-1.,0.127784445276116));
#29660=CARTESIAN_POINT('Ctrl Pts',(2.07892715110967,1.,0.127784445276116));
#29661=CARTESIAN_POINT('Ctrl Pts',(2.08470840653628,-1.,0.125423679412058));
#29662=CARTESIAN_POINT('Ctrl Pts',(2.08470840653628,1.,0.125423679412058));
#29663=CARTESIAN_POINT('Ctrl Pts',(2.09048392424826,-1.,0.123018905621083));
#29664=CARTESIAN_POINT('Ctrl Pts',(2.09048392424826,1.,0.123018905621083));
#29665=CARTESIAN_POINT('Ctrl Pts',(2.09625292867756,-1.,0.120570567965129));
#29666=CARTESIAN_POINT('Ctrl Pts',(2.09625292867756,1.,0.120570567965129));
#29667=CARTESIAN_POINT('Ctrl Pts',(2.10201512132945,-1.,0.118079107988368));
#29668=CARTESIAN_POINT('Ctrl Pts',(2.10201512132945,1.,0.118079107988368));
#29669=CARTESIAN_POINT('Ctrl Pts',(2.10777050261359,-1.,0.11554495768794));
#29670=CARTESIAN_POINT('Ctrl Pts',(2.10777050261359,1.,0.11554495768794));
#29671=CARTESIAN_POINT('Ctrl Pts',(2.11351924490335,-1.,0.112968534419746));
#29672=CARTESIAN_POINT('Ctrl Pts',(2.11351924490335,1.,0.112968534419746));
#29673=CARTESIAN_POINT('Ctrl Pts',(2.11926155590849,-1.,0.11035023613502));
#29674=CARTESIAN_POINT('Ctrl Pts',(2.11926155590849,1.,0.11035023613502));
#29675=CARTESIAN_POINT('Ctrl Pts',(2.12499752306927,-1.,0.107690435231068));
#29676=CARTESIAN_POINT('Ctrl Pts',(2.12499752306927,1.,0.107690435231068));
#29677=CARTESIAN_POINT('Ctrl Pts',(2.1307270488718,-1.,0.104989479152703));
#29678=CARTESIAN_POINT('Ctrl Pts',(2.1307270488718,1.,0.104989479152703));
#29679=CARTESIAN_POINT('Ctrl Pts',(2.13644992667052,-1.,0.102247700556063));
#29680=CARTESIAN_POINT('Ctrl Pts',(2.13644992667052,1.,0.102247700556063));
#29681=CARTESIAN_POINT('Ctrl Pts',(2.14216588395974,-1.,0.0994654261990741));
#29682=CARTESIAN_POINT('Ctrl Pts',(2.14216588395974,1.,0.0994654261990741));
#29683=CARTESIAN_POINT('Ctrl Pts',(2.14787463531864,-1.,0.0966429852305688));
#29684=CARTESIAN_POINT('Ctrl Pts',(2.14787463531864,1.,0.0966429852305688));
#29685=CARTESIAN_POINT('Ctrl Pts',(2.15357593978377,-1.,0.0937807218868344));
#29686=CARTESIAN_POINT('Ctrl Pts',(2.15357593978377,1.,0.0937807218868344));
#29687=CARTESIAN_POINT('Ctrl Pts',(2.15926961544808,-1.,0.0908789888108265));
#29688=CARTESIAN_POINT('Ctrl Pts',(2.15926961544808,1.,0.0908789888108265));
#29689=CARTESIAN_POINT('Ctrl Pts',(2.16495552645275,-1.,0.0879381291387821));
#29690=CARTESIAN_POINT('Ctrl Pts',(2.16495552645275,1.,0.0879381291387821));
#29691=CARTESIAN_POINT('Ctrl Pts',(2.17063357871031,-1.,0.0849584620835642));
#29692=CARTESIAN_POINT('Ctrl Pts',(2.17063357871031,1.,0.0849584620835642));
#29693=CARTESIAN_POINT('Ctrl Pts',(2.1763037121106,-1.,0.0819402680871938));
#29694=CARTESIAN_POINT('Ctrl Pts',(2.1763037121106,1.,0.0819402680871938));
#29695=CARTESIAN_POINT('Ctrl Pts',(2.18196589448304,-1.,0.0788837727683226));
#29696=CARTESIAN_POINT('Ctrl Pts',(2.18196589448304,1.,0.0788837727683226));
#29697=CARTESIAN_POINT('Ctrl Pts',(2.1876201139874,-1.,0.075789146583341));
#29698=CARTESIAN_POINT('Ctrl Pts',(2.1876201139874,1.,0.075789146583341));
#29699=CARTESIAN_POINT('Ctrl Pts',(2.19213712012956,-1.,0.0732830357304275));
#29700=CARTESIAN_POINT('Ctrl Pts',(2.19213712012956,1.,0.0732830357304275));
#29701=CARTESIAN_POINT('Ctrl Pts',(2.19552129483562,-1.,0.0713863779524626));
#29702=CARTESIAN_POINT('Ctrl Pts',(2.19552129483562,1.,0.0713863779524626));
#29703=CARTESIAN_POINT('Ctrl Pts',(2.19777582085261,-1.,0.0701143536324925));
#29704=CARTESIAN_POINT('Ctrl Pts',(2.19777582085261,1.,0.0701143536324925));
#29705=CARTESIAN_POINT('Ctrl Pts',(2.19890268624765,-1.,0.0694764450219582));
#29706=CARTESIAN_POINT('Ctrl Pts',(2.19890268624765,1.,0.0694764450219582));
#29707=CARTESIAN_POINT('',(1.74236521665491,1.,0.163289472382896));
#29708=CARTESIAN_POINT('Ctrl Pts',(1.74236521665491,1.,0.163289472382896));
#29709=CARTESIAN_POINT('Ctrl Pts',(1.74720349503904,1.,0.163814161002474));
#29710=CARTESIAN_POINT('Ctrl Pts',(1.75666056640041,1.,0.164834765708484));
#29711=CARTESIAN_POINT('Ctrl Pts',(1.77018771687692,1.,0.166279355148738));
#29712=CARTESIAN_POINT('Ctrl Pts',(1.78690649988931,1.,0.16803277280837));
#29713=CARTESIAN_POINT('Ctrl Pts',(1.80561530633924,1.,0.169936923908078));
#29714=CARTESIAN_POINT('Ctrl Pts',(1.82215766815414,1.,0.171554770207306));
#29715=CARTESIAN_POINT('Ctrl Pts',(1.83658380530747,1.,0.17288944289442));
#29716=CARTESIAN_POINT('Ctrl Pts',(1.84898113200543,1.,0.173946627589401));
#29717=CARTESIAN_POINT('Ctrl Pts',(1.85948367089838,1.,0.174735259276856));
#29718=CARTESIAN_POINT('Ctrl Pts',(1.86828349694972,1.,0.1752683375909));
#29719=CARTESIAN_POINT('Ctrl Pts',(1.87563767773249,1.,0.175563480746205));
#29720=CARTESIAN_POINT('Ctrl Pts',(1.88188663144846,1.,0.175644148889271));
#29721=CARTESIAN_POINT('Ctrl Pts',(1.88742606272818,1.,0.175538155840286));
#29722=CARTESIAN_POINT('Ctrl Pts',(1.89264630198279,1.,0.175274276190664));
#29723=CARTESIAN_POINT('Ctrl Pts',(1.89788101117148,1.,0.174879405091277));
#29724=CARTESIAN_POINT('Ctrl Pts',(1.90335253863003,1.,0.174375518661222));
#29725=CARTESIAN_POINT('Ctrl Pts',(1.90911693975475,1.,0.173776635257983));
#29726=CARTESIAN_POINT('Ctrl Pts',(1.91511429159681,1.,0.173090695383619));
#29727=CARTESIAN_POINT('Ctrl Pts',(1.92122334398034,1.,0.172321621259556));
#29728=CARTESIAN_POINT('Ctrl Pts',(1.92731093582,1.,0.17147119153296));
#29729=CARTESIAN_POINT('Ctrl Pts',(1.93329183155455,1.,0.170541253116136));
#29730=CARTESIAN_POINT('Ctrl Pts',(1.93915639211497,1.,0.169534904817425));
#29731=CARTESIAN_POINT('Ctrl Pts',(1.94493757756879,1.,0.168455741607515));
#29732=CARTESIAN_POINT('Ctrl Pts',(1.95069027794286,1.,0.167307501784469));
#29733=CARTESIAN_POINT('Ctrl Pts',(1.95646759718755,1.,0.166093592002832));
#29734=CARTESIAN_POINT('Ctrl Pts',(1.96229379940174,1.,0.1648165689203));
#29735=CARTESIAN_POINT('Ctrl Pts',(1.96816512678,1.,0.16347818545776));
#29736=CARTESIAN_POINT('Ctrl Pts',(1.97406280235204,1.,0.162079693556302));
#29737=CARTESIAN_POINT('Ctrl Pts',(1.97996195437557,1.,0.16062206078461));
#29738=CARTESIAN_POINT('Ctrl Pts',(1.98584238283279,1.,0.159106226437288));
#29739=CARTESIAN_POINT('Ctrl Pts',(1.99169810931893,1.,0.157533331459215));
#29740=CARTESIAN_POINT('Ctrl Pts',(1.99753284771487,1.,0.155904629548774));
#29741=CARTESIAN_POINT('Ctrl Pts',(2.00335565310539,1.,0.154221403049719));
#29742=CARTESIAN_POINT('Ctrl Pts',(2.00917680318426,1.,0.152484883621452));
#29743=CARTESIAN_POINT('Ctrl Pts',(2.01500291940243,1.,0.150696157673084));
#29744=CARTESIAN_POINT('Ctrl Pts',(2.02083464969897,1.,0.148856124775342));
#29745=CARTESIAN_POINT('Ctrl Pts',(2.02666926182017,1.,0.146965557332586));
#29746=CARTESIAN_POINT('Ctrl Pts',(2.03250223739941,1.,0.145025140186058));
#29747=CARTESIAN_POINT('Ctrl Pts',(2.03832911025913,1.,0.143035515058208));
#29748=CARTESIAN_POINT('Ctrl Pts',(2.04414757947919,1.,0.140997332152545));
#29749=CARTESIAN_POINT('Ctrl Pts',(2.04995762001333,1.,0.138911255368966));
#29750=CARTESIAN_POINT('Ctrl Pts',(2.0557604441427,1.,0.136777941218044));
#29751=CARTESIAN_POINT('Ctrl Pts',(2.06155781517844,1.,0.134598026192107));
#29752=CARTESIAN_POINT('Ctrl Pts',(2.06735123910319,1.,0.132372111547709));
#29753=CARTESIAN_POINT('Ctrl Pts',(2.07314114713047,1.,0.1301007483284));
#29754=CARTESIAN_POINT('Ctrl Pts',(2.07892715110967,1.,0.127784445276116));
#29755=CARTESIAN_POINT('Ctrl Pts',(2.08470840653628,1.,0.125423679412058));
#29756=CARTESIAN_POINT('Ctrl Pts',(2.09048392424826,1.,0.123018905621083));
#29757=CARTESIAN_POINT('Ctrl Pts',(2.09625292867756,1.,0.120570567965129));
#29758=CARTESIAN_POINT('Ctrl Pts',(2.10201512132945,1.,0.118079107988368));
#29759=CARTESIAN_POINT('Ctrl Pts',(2.10777050261359,1.,0.11554495768794));
#29760=CARTESIAN_POINT('Ctrl Pts',(2.11351924490335,1.,0.112968534419746));
#29761=CARTESIAN_POINT('Ctrl Pts',(2.11926155590849,1.,0.11035023613502));
#29762=CARTESIAN_POINT('Ctrl Pts',(2.12499752306927,1.,0.107690435231068));
#29763=CARTESIAN_POINT('Ctrl Pts',(2.1307270488718,1.,0.104989479152703));
#29764=CARTESIAN_POINT('Ctrl Pts',(2.13644992667052,1.,0.102247700556063));
#29765=CARTESIAN_POINT('Ctrl Pts',(2.14216588395974,1.,0.0994654261990741));
#29766=CARTESIAN_POINT('Ctrl Pts',(2.14787463531864,1.,0.0966429852305688));
#29767=CARTESIAN_POINT('Ctrl Pts',(2.15357593978377,1.,0.0937807218868344));
#29768=CARTESIAN_POINT('Ctrl Pts',(2.15926961544808,1.,0.0908789888108265));
#29769=CARTESIAN_POINT('Ctrl Pts',(2.16495552645275,1.,0.0879381291387821));
#29770=CARTESIAN_POINT('Ctrl Pts',(2.17063357871031,1.,0.0849584620835642));
#29771=CARTESIAN_POINT('Ctrl Pts',(2.1763037121106,1.,0.0819402680871938));
#29772=CARTESIAN_POINT('Ctrl Pts',(2.18196589448304,1.,0.0788837727683226));
#29773=CARTESIAN_POINT('Ctrl Pts',(2.1876201139874,1.,0.075789146583341));
#29774=CARTESIAN_POINT('Ctrl Pts',(2.19213712012956,1.,0.0732830357304275));
#29775=CARTESIAN_POINT('Ctrl Pts',(2.19552129483562,1.,0.0713863779524626));
#29776=CARTESIAN_POINT('Ctrl Pts',(2.19777582085261,1.,0.0701143536324925));
#29777=CARTESIAN_POINT('Ctrl Pts',(2.19890268624765,1.,0.0694764450219582));
#29778=CARTESIAN_POINT('',(1.74236521665491,0.,0.163289472382896));
#29779=CARTESIAN_POINT('Origin',(0.,1.,0.));
#29780=CARTESIAN_POINT('Origin',(0.,1.,0.));
#29781=CARTESIAN_POINT('Origin',(0.,0.,0.));
#53846=UNCERTAINTY_MEASURE_WITH_UNIT(LENGTH_MEASURE(0.001),#53910,
'DISTANCE_ACCURACY_VALUE',
'Maximum model space distance between geometric entities at asserted c
onnectivities');
#53859=UNCERTAINTY_MEASURE_WITH_UNIT(LENGTH_MEASURE(0.001),#53910,
'DISTANCE_ACCURACY_VALUE',
'Maximum model space distance between geometric entities at asserted c
onnectivities');
#53896=(
GEOMETRIC_REPRESENTATION_CONTEXT(3)
GLOBAL_UNCERTAINTY_ASSIGNED_CONTEXT((#53846))
GLOBAL_UNIT_ASSIGNED_CONTEXT((#53910,#53912,#53913))
REPRESENTATION_CONTEXT('','3D')
);
#53909=(
GEOMETRIC_REPRESENTATION_CONTEXT(3)
GLOBAL_UNCERTAINTY_ASSIGNED_CONTEXT((#53859))
GLOBAL_UNIT_ASSIGNED_CONTEXT((#53910,#53912,#53913))
REPRESENTATION_CONTEXT('','3D')
);
#53910=(
LENGTH_UNIT()
NAMED_UNIT(*)
SI_UNIT(.CENTI.,.METRE.)
);
#53912=(
NAMED_UNIT(*)
PLANE_ANGLE_UNIT()
SI_UNIT($,.RADIAN.)
);
#53913=(
NAMED_UNIT(*)
SI_UNIT($,.STERADIAN.)
SOLID_ANGLE_UNIT()
);
#53950=SHAPE_DEFINITION_REPRESENTATION(#54048,#54122);
#54048=PRODUCT_DEFINITION_SHAPE('',$,#54172);
#54122=SHAPE_REPRESENTATION('',(#12560),#53896);
#54135=PRODUCT_DEFINITION_CONTEXT('part definition',#54284,'design');
#54172=PRODUCT_DEFINITION('Spur Gear - Module 2, 20 Teeth, 12 mm Bore',
'Spur Gear - Module 2, 20 Teeth, 12 mm Bore',#54221,#54135);
#54221=PRODUCT_DEFINITION_FORMATION('',$,#54322);
#54284=APPLICATION_CONTEXT(
'Core Data for Automotive Mechanical Design Process');
#54285=PRODUCT_CONTEXT('part definition',#54284,'mechanical');
#54322=PRODUCT('Spur Gear - Module 2, 20 Teeth, 12 mm Bore',
'Spur Gear - Module 2, 20 Teeth, 12 mm Bore',
'Spur Gear - Module 2, 20 Teeth, 12 mm Bore',(#54285));
#54405=COLOUR_RGB('Off White',0.89,0.88,0.83);
#54406=FILL_AREA_STYLE_COLOUR('',#54405);
#54407=FILL_AREA_STYLE('',(#54406));
#54408=SURFACE_STYLE_FILL_AREA(#54407);
#54409=SURFACE_SIDE_STYLE('',(#54408));
#54410=SURFACE_STYLE_USAGE(.BOTH.,#54409);
#54411=PRESENTATION_STYLE_ASSIGNMENT((#54410));
ENDSEC;
END-ISO-10303-21;
